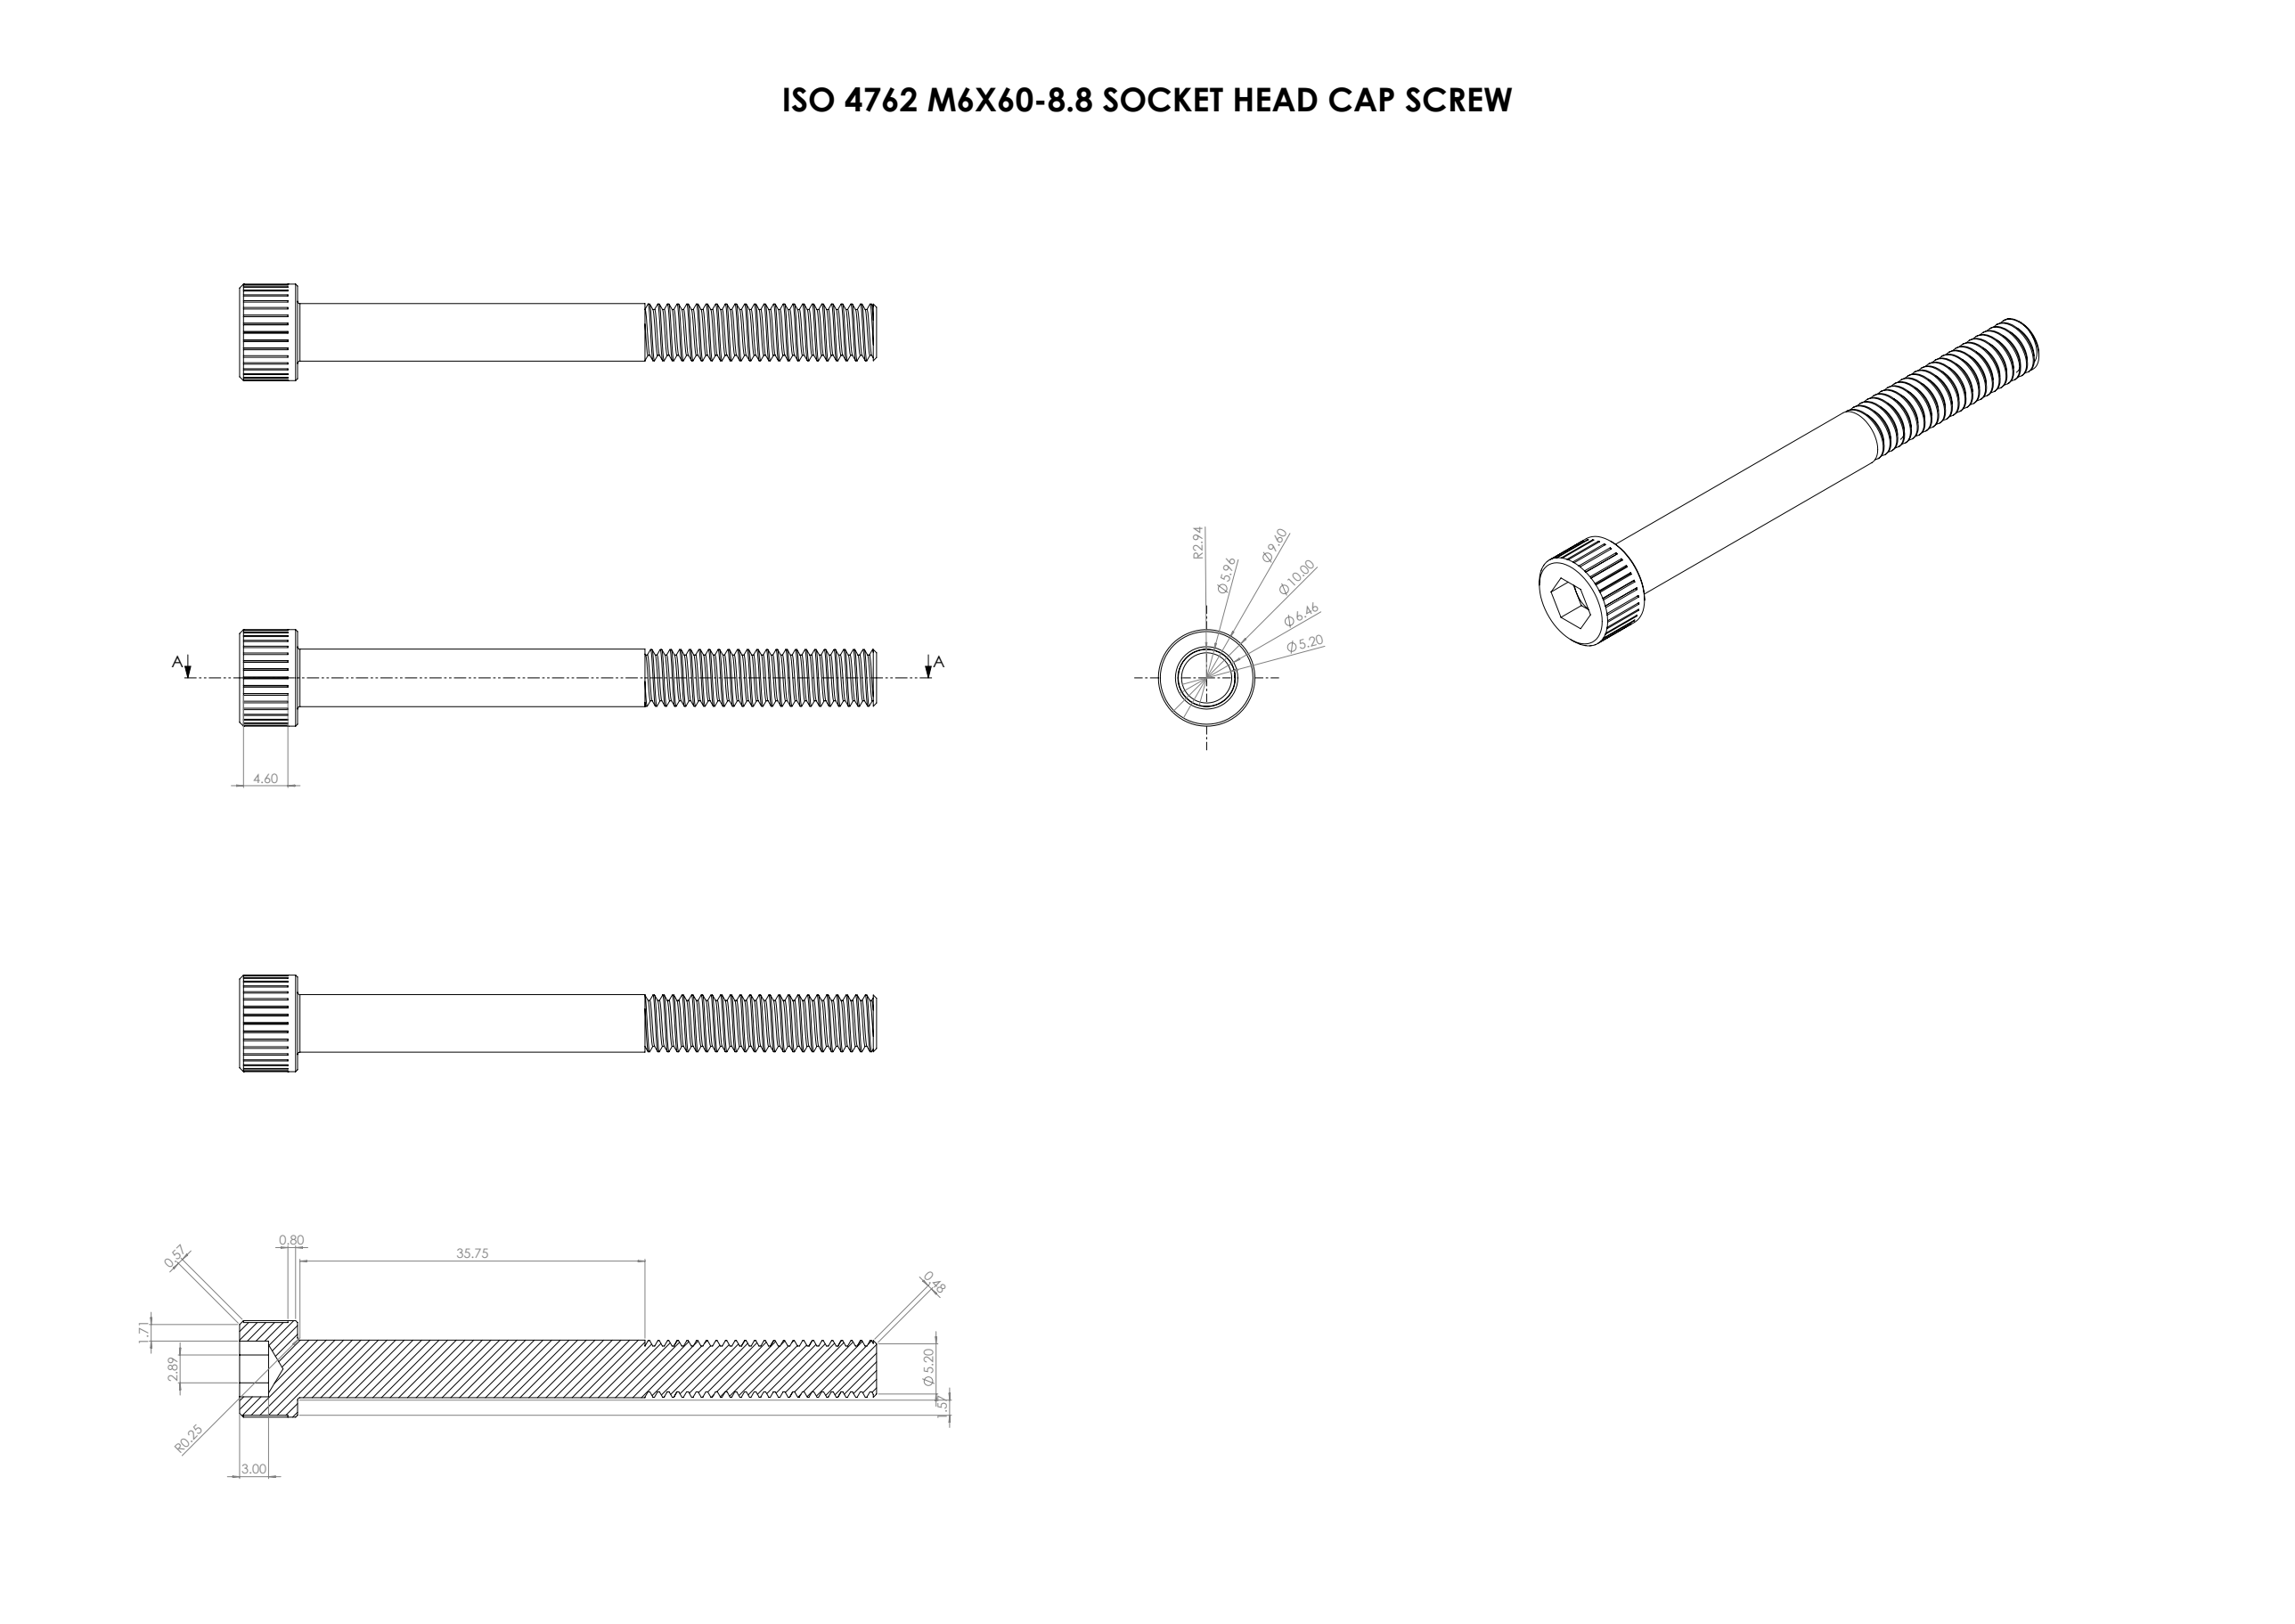
ISO-10303-21;
HEADER;
/* Generated by software containing ST-Developer
 * from STEP Tools, Inc. (www.steptools.com) 
 */

FILE_DESCRIPTION(
/* description */ (''),
/* implementation_level */ '2;1');

FILE_NAME(
/* name */ 
'09_ISO_4762_M6x60-8.8_Socket_Head_Cap_Screw.step',
/* time_stamp */ '2026-10-22T00:21:42-07:00',
/* author */ (''),
/* organization */ (''),
/* preprocessor_version */ 'ST-DEVELOPER v20.2',
/* originating_system */ 'Autodesk Translation Framework v15.15.0.0',
/* authorisation */ '');

FILE_SCHEMA (('AUTOMOTIVE_DESIGN { 1 0 10303 214 3 1 1 }'));
ENDSEC;

DATA;
#10=MECHANICAL_DESIGN_GEOMETRIC_PRESENTATION_REPRESENTATION('',(#213),#31638);
#191=SHAPE_REPRESENTATION_RELATIONSHIP('SRR','None',#31713,#202);
#202=ADVANCED_BREP_SHAPE_REPRESENTATION('',(#224),#31635);
#213=STYLED_ITEM('',(#31837),#224);
#224=MANIFOLD_SOLID_BREP('Socket head cap screw',#12488);
#245=TOROIDAL_SURFACE('',#13459,0.323,0.025);
#307=CYLINDRICAL_SURFACE('',#13176,0.2942);
#308=CYLINDRICAL_SURFACE('',#13178,0.2942);
#309=CYLINDRICAL_SURFACE('',#13179,0.2942);
#310=CYLINDRICAL_SURFACE('',#13180,0.2942);
#311=CYLINDRICAL_SURFACE('',#13181,0.2942);
#312=CYLINDRICAL_SURFACE('',#13182,0.2942);
#313=CYLINDRICAL_SURFACE('',#13183,0.2942);
#314=CYLINDRICAL_SURFACE('',#13184,0.2942);
#315=CYLINDRICAL_SURFACE('',#13185,0.2942);
#316=CYLINDRICAL_SURFACE('',#13186,0.2942);
#317=CYLINDRICAL_SURFACE('',#13187,0.2942);
#318=CYLINDRICAL_SURFACE('',#13188,0.2942);
#319=CYLINDRICAL_SURFACE('',#13189,0.2942);
#320=CYLINDRICAL_SURFACE('',#13190,0.2942);
#321=CYLINDRICAL_SURFACE('',#13191,0.2942);
#322=CYLINDRICAL_SURFACE('',#13192,0.2942);
#323=CYLINDRICAL_SURFACE('',#13193,0.2942);
#324=CYLINDRICAL_SURFACE('',#13194,0.2942);
#325=CYLINDRICAL_SURFACE('',#13195,0.2942);
#326=CYLINDRICAL_SURFACE('',#13196,0.2942);
#327=CYLINDRICAL_SURFACE('',#13197,0.2942);
#328=CYLINDRICAL_SURFACE('',#13198,0.2942);
#329=CYLINDRICAL_SURFACE('',#13199,0.2942);
#330=CYLINDRICAL_SURFACE('',#13200,0.2942);
#331=CYLINDRICAL_SURFACE('',#13201,0.237175);
#332=CYLINDRICAL_SURFACE('',#13203,0.237175);
#333=CYLINDRICAL_SURFACE('',#13205,0.237175);
#334=CYLINDRICAL_SURFACE('',#13206,0.237175);
#335=CYLINDRICAL_SURFACE('',#13207,0.237175);
#336=CYLINDRICAL_SURFACE('',#13208,0.237175);
#337=CYLINDRICAL_SURFACE('',#13209,0.237175);
#338=CYLINDRICAL_SURFACE('',#13210,0.237175);
#339=CYLINDRICAL_SURFACE('',#13211,0.237175);
#340=CYLINDRICAL_SURFACE('',#13212,0.237175);
#341=CYLINDRICAL_SURFACE('',#13213,0.237175);
#342=CYLINDRICAL_SURFACE('',#13214,0.237175);
#343=CYLINDRICAL_SURFACE('',#13215,0.237175);
#344=CYLINDRICAL_SURFACE('',#13216,0.237175);
#345=CYLINDRICAL_SURFACE('',#13217,0.237175);
#346=CYLINDRICAL_SURFACE('',#13218,0.237175);
#347=CYLINDRICAL_SURFACE('',#13219,0.237175);
#348=CYLINDRICAL_SURFACE('',#13220,0.237175);
#349=CYLINDRICAL_SURFACE('',#13221,0.237175);
#350=CYLINDRICAL_SURFACE('',#13222,0.237175);
#351=CYLINDRICAL_SURFACE('',#13223,0.237175);
#352=CYLINDRICAL_SURFACE('',#13224,0.237175);
#353=CYLINDRICAL_SURFACE('',#13225,0.237175);
#354=CYLINDRICAL_SURFACE('',#13226,0.237175);
#355=CYLINDRICAL_SURFACE('',#13231,0.237175);
#356=CYLINDRICAL_SURFACE('',#13463,0.298);
#357=CYLINDRICAL_SURFACE('',#13470,0.2942);
#358=CYLINDRICAL_SURFACE('',#13475,0.5);
#437=CONICAL_SURFACE('',#13232,0.124996333279554,1.03037682652431);
#438=CONICAL_SURFACE('',#13469,0.28,0.785398163397448);
#439=CONICAL_SURFACE('',#13473,0.49,0.785398163397449);
#440=CONICAL_SURFACE('',#13512,0.48,0.785398163397448);
#1046=B_SPLINE_CURVE_WITH_KNOTS('',3,(#26914,#26915,#26916,#26917,#26918,
#26919,#26920,#26921,#26922,#26923),.UNSPECIFIED.,.F.,.F.,(4,3,3,4),(-4.09293042013064,
-3.99248307740831,-2.99436230805624,-2.06863817490914),.UNSPECIFIED.);
#1047=B_SPLINE_CURVE_WITH_KNOTS('',3,(#26926,#26927,#26928,#26929,#26930,
#26931,#26932),.UNSPECIFIED.,.F.,.F.,(4,3,4),(0.,0.998120769352068,1.11730040836818),
 .UNSPECIFIED.);
#1048=B_SPLINE_CURVE_WITH_KNOTS('',3,(#26937,#26938,#26939,#26940,#26941,
#26942,#26943,#26944,#26945,#26946,#26947,#26948,#26949,#26950,#26951,#26952,
#26953,#26954,#26955,#26956,#26957,#26958),.UNSPECIFIED.,.F.,.F.,(4,3,3,
3,3,3,3,4),(-10.3761157273103,-9.98120769352079,-8.98308692416871,-7.98496615481663,
-6.98684538546455,-5.98872461611248,-4.99060384676039,-4.09293042013064),
 .UNSPECIFIED.);
#1049=B_SPLINE_CURVE_WITH_KNOTS('',3,(#26959,#26960,#26961,#26962,#26963,
#26964,#26965,#26966,#26967,#26968,#26969,#26970,#26971,#26972,#26973,#26974,
#26975,#26976,#26977,#26978,#26979,#26980),.UNSPECIFIED.,.F.,.F.,(4,3,3,
3,3,3,3,4),(1.11730040836818,1.99624153870415,2.99436230805623,3.99248307740831,
4.99060384676039,5.98872461611247,6.98684538546454,7.40048571554779),
 .UNSPECIFIED.);
#1050=B_SPLINE_CURVE_WITH_KNOTS('',3,(#26985,#26986,#26987,#26988,#26989,
#26990,#26991,#26992,#26993,#26994,#26995,#26996,#26997,#26998,#26999,#27000,
#27001,#27002,#27003,#27004,#27005,#27006),.UNSPECIFIED.,.F.,.F.,(4,3,3,
3,3,3,3,4),(-16.6593010344898,-15.9699323096333,-14.9718115402812,-13.9736907709291,
-12.975570001577,-11.9774492322249,-10.9793284628729,-10.3761157273103),
 .UNSPECIFIED.);
#1051=B_SPLINE_CURVE_WITH_KNOTS('',3,(#27007,#27008,#27009,#27010,#27011,
#27012,#27013,#27014,#27015,#27016,#27017,#27018,#27019,#27020,#27021,#27022,
#27023,#27024,#27025,#27026,#27027,#27028),.UNSPECIFIED.,.F.,.F.,(4,3,3,
3,3,3,3,4),(7.40048571554779,7.98496615481663,8.9830869241687,9.98120769352078,
10.9793284628729,11.9774492322249,12.975570001577,13.6836710227274),
 .UNSPECIFIED.);
#1052=B_SPLINE_CURVE_WITH_KNOTS('',3,(#27033,#27034,#27035,#27036,#27037,
#27038,#27039,#27040,#27041,#27042,#27043,#27044,#27045,#27046,#27047,#27048,
#27049,#27050,#27051,#27052,#27053,#27054),.UNSPECIFIED.,.F.,.F.,(4,3,3,
3,3,3,3,4),(-22.9424863416694,-21.9586569257457,-20.9605361563937,-19.9624153870416,
-18.9642946176895,-17.9661738483374,-16.9680530789853,-16.6593010344898),
 .UNSPECIFIED.);
#1053=B_SPLINE_CURVE_WITH_KNOTS('',3,(#27055,#27056,#27057,#27058,#27059,
#27060,#27061,#27062,#27063,#27064,#27065,#27066,#27067,#27068,#27069,#27070,
#27071,#27072,#27073,#27074,#27075,#27076,#27077,#27078,#27079),
 .UNSPECIFIED.,.F.,.F.,(4,3,3,3,3,3,3,3,4),(13.6836710227274,13.9736907709291,
14.9718115402812,15.9699323096333,16.9680530789853,17.9661738483374,18.9642946176895,
19.9624153870416,19.966856329907),.UNSPECIFIED.);
#1054=B_SPLINE_CURVE_WITH_KNOTS('',3,(#27084,#27085,#27086,#27087,#27088,
#27089,#27090,#27091,#27092,#27093,#27094,#27095,#27096,#27097,#27098,#27099,
#27100,#27101,#27102,#27103,#27104,#27105,#27106,#27107,#27108),
 .UNSPECIFIED.,.F.,.F.,(4,3,3,3,3,3,3,3,4),(-29.225671648849,-28.9455023112103,
-27.9473815418582,-26.9492607725061,-25.9511400031541,-24.953019233802,
-23.9548984644499,-22.9567776950978,-22.9424863416694),.UNSPECIFIED.);
#1055=B_SPLINE_CURVE_WITH_KNOTS('',3,(#27109,#27110,#27111,#27112,#27113,
#27114,#27115,#27116,#27117,#27118,#27119,#27120,#27121,#27122,#27123,#27124,
#27125,#27126,#27127,#27128,#27129,#27130),.UNSPECIFIED.,.F.,.F.,(4,3,3,
3,3,3,3,4),(19.966856329907,20.9605361563937,21.9586569257457,22.9567776950978,
23.9548984644499,24.953019233802,25.9511400031541,26.2500416370865),
 .UNSPECIFIED.);
#1056=B_SPLINE_CURVE_WITH_KNOTS('',3,(#27135,#27136,#27137,#27138,#27139,
#27140,#27141,#27142,#27143,#27144,#27145,#27146,#27147,#27148,#27149,#27150,
#27151,#27152,#27153,#27154,#27155,#27156),.UNSPECIFIED.,.F.,.F.,(4,3,3,
3,3,3,3,4),(-35.5088569560286,-34.9342269273228,-33.9361061579707,-32.9379853886186,
-31.9398646192665,-30.9417438499144,-29.9436230805624,-29.225671648849),
 .UNSPECIFIED.);
#1057=B_SPLINE_CURVE_WITH_KNOTS('',3,(#27157,#27158,#27159,#27160,#27161,
#27162,#27163,#27164,#27165,#27166,#27167,#27168,#27169,#27170,#27171,#27172,
#27173,#27174,#27175,#27176,#27177,#27178),.UNSPECIFIED.,.F.,.F.,(4,3,3,
3,3,3,3,4),(26.2500416370865,26.9492607725061,27.9473815418582,28.9455023112103,
29.9436230805624,30.9417438499144,31.9398646192665,32.5332269442662),
 .UNSPECIFIED.);
#1058=B_SPLINE_CURVE_WITH_KNOTS('',3,(#27183,#27184,#27185,#27186,#27187,
#27188,#27189,#27190,#27191,#27192,#27193,#27194,#27195,#27196,#27197,#27198,
#27199,#27200,#27201,#27202,#27203,#27204),.UNSPECIFIED.,.F.,.F.,(4,3,3,
3,3,3,3,4),(-41.7920422632082,-40.9229515434352,-39.9248307740831,-38.9267100047311,
-37.928589235379,-36.9304684660269,-35.9323476966748,-35.5088569560286),
 .UNSPECIFIED.);
#1059=B_SPLINE_CURVE_WITH_KNOTS('',3,(#27205,#27206,#27207,#27208,#27209,
#27210,#27211,#27212,#27213,#27214,#27215,#27216,#27217,#27218,#27219,#27220,
#27221,#27222,#27223,#27224,#27225,#27226),.UNSPECIFIED.,.F.,.F.,(4,3,3,
3,3,3,3,4),(32.5332269442662,32.9379853886186,33.9361061579707,34.9342269273227,
35.9323476966748,36.9304684660269,37.928589235379,38.8164122514457),
 .UNSPECIFIED.);
#1060=B_SPLINE_CURVE_WITH_KNOTS('',3,(#27231,#27232,#27233,#27234,#27235,
#27236,#27237,#27238,#27239,#27240,#27241,#27242,#27243,#27244,#27245,#27246,
#27247,#27248,#27249,#27250,#27251,#27252,#27253,#27254,#27255),
 .UNSPECIFIED.,.F.,.F.,(4,3,3,3,3,3,3,3,4),(-48.0752275703878,-47.9097969288998,
-46.9116761595477,-45.9135553901956,-44.9154346208435,-43.9173138514915,
-42.9191930821394,-41.9210723127873,-41.7920422632082),.UNSPECIFIED.);
#1061=B_SPLINE_CURVE_WITH_KNOTS('',3,(#27256,#27257,#27258,#27259,#27260,
#27261,#27262,#27263,#27264,#27265,#27266,#27267,#27268,#27269,#27270,#27271,
#27272,#27273,#27274,#27275,#27276,#27277,#27278,#27279,#27280),
 .UNSPECIFIED.,.F.,.F.,(4,3,3,3,3,3,3,3,4),(38.8164122514457,38.9267100047311,
39.9248307740831,40.9229515434352,41.9210723127873,42.9191930821394,43.9173138514915,
44.9154346208435,45.0995975586253),.UNSPECIFIED.);
#1062=B_SPLINE_CURVE_WITH_KNOTS('',3,(#27285,#27286,#27287,#27288,#27289,
#27290,#27291,#27292,#27293,#27294,#27295,#27296,#27297,#27298,#27299,#27300,
#27301,#27302,#27303,#27304,#27305,#27306),.UNSPECIFIED.,.F.,.F.,(4,3,3,
3,3,3,3,4),(-54.3584128775674,-53.8985215450123,-52.9004007756602,-51.9022800063081,
-50.904159236956,-49.9060384676039,-48.9079176982519,-48.0752275703878),
 .UNSPECIFIED.);
#1063=B_SPLINE_CURVE_WITH_KNOTS('',3,(#27307,#27308,#27309,#27310,#27311,
#27312,#27313,#27314,#27315,#27316,#27317,#27318,#27319,#27320,#27321,#27322,
#27323,#27324,#27325,#27326,#27327,#27328),.UNSPECIFIED.,.F.,.F.,(4,3,3,
3,3,3,3,4),(45.0995975586253,45.9135553901956,46.9116761595477,47.9097969288998,
48.9079176982519,49.9060384676039,50.904159236956,51.3827828658049),
 .UNSPECIFIED.);
#1064=B_SPLINE_CURVE_WITH_KNOTS('',3,(#27333,#27334,#27335,#27336,#27337,
#27338,#27339,#27340,#27341,#27342,#27343,#27344,#27345,#27346,#27347,#27348,
#27349,#27350,#27351,#27352,#27353,#27354),.UNSPECIFIED.,.F.,.F.,(4,3,3,
3,3,3,3,4),(-60.6415981847469,-59.8872461611247,-58.8891253917727,-57.8910046224206,
-56.8928838530685,-55.8947630837164,-54.8966423143643,-54.3584128775674),
 .UNSPECIFIED.);
#1065=B_SPLINE_CURVE_WITH_KNOTS('',3,(#27355,#27356,#27357,#27358,#27359,
#27360,#27361,#27362,#27363,#27364,#27365,#27366,#27367,#27368,#27369,#27370,
#27371,#27372,#27373,#27374,#27375,#27376),.UNSPECIFIED.,.F.,.F.,(4,3,3,
3,3,3,3,4),(51.3827828658049,51.9022800063081,52.9004007756602,53.8985215450123,
54.8966423143643,55.8947630837164,56.8928838530685,57.6659681729845),
 .UNSPECIFIED.);
#1066=B_SPLINE_CURVE_WITH_KNOTS('',3,(#27381,#27382,#27383,#27384,#27385,
#27386,#27387,#27388,#27389,#27390,#27391,#27392,#27393,#27394,#27395,#27396,
#27397,#27398,#27399,#27400,#27401,#27402,#27403,#27404,#27405),
 .UNSPECIFIED.,.F.,.F.,(4,3,3,3,3,3,3,3,4),(-66.9247834919266,-66.8740915465893,
-65.8759707772372,-64.8778500078851,-63.879729238533,-62.881608469181,-61.8834876998289,
-60.8853669304768,-60.6415981847469),.UNSPECIFIED.);
#1067=B_SPLINE_CURVE_WITH_KNOTS('',3,(#27406,#27407,#27408,#27409,#27410,
#27411,#27412,#27413,#27414,#27415,#27416,#27417,#27418,#27419,#27420,#27421,
#27422,#27423,#27424,#27425,#27426,#27427,#27428,#27429,#27430),
 .UNSPECIFIED.,.F.,.F.,(4,3,3,3,3,3,3,3,4),(57.6659681729845,57.8910046224206,
58.8891253917727,59.8872461611247,60.8853669304768,61.8834876998289,62.881608469181,
63.8797292385331,63.9491534801641),.UNSPECIFIED.);
#1068=B_SPLINE_CURVE_WITH_KNOTS('',3,(#27435,#27436,#27437,#27438,#27439,
#27440,#27441,#27442,#27443,#27444,#27445,#27446,#27447,#27448,#27449,#27450,
#27451,#27452,#27453,#27454,#27455,#27456),.UNSPECIFIED.,.F.,.F.,(4,3,3,
3,3,3,3,4),(-73.2079687991062,-72.8628161627017,-71.8646953933497,-70.8665746239976,
-69.8684538546455,-68.8703330852934,-67.8722123159413,-66.9247834919266),
 .UNSPECIFIED.);
#1069=B_SPLINE_CURVE_WITH_KNOTS('',3,(#27457,#27458,#27459,#27460,#27461,
#27462,#27463,#27464,#27465,#27466,#27467,#27468,#27469,#27470,#27471,#27472,
#27473,#27474,#27475,#27476,#27477,#27478),.UNSPECIFIED.,.F.,.F.,(4,3,3,
3,3,3,3,4),(63.9491534801641,64.8778500078851,65.8759707772372,66.8740915465893,
67.8722123159414,68.8703330852934,69.8684538546455,70.2323387873437),
 .UNSPECIFIED.);
#1070=B_SPLINE_CURVE_WITH_KNOTS('',3,(#27483,#27484,#27485,#27486,#27487,
#27488,#27489,#27490,#27491,#27492,#27493,#27494,#27495,#27496,#27497,#27498,
#27499,#27500,#27501,#27502,#27503,#27504),.UNSPECIFIED.,.F.,.F.,(4,3,3,
3,3,3,3,4),(-79.4911541062857,-78.8515407788142,-77.8534200094622,-76.8552992401101,
-75.857178470758,-74.8590577014059,-73.8609369320538,-73.2079687991062),
 .UNSPECIFIED.);
#1071=B_SPLINE_CURVE_WITH_KNOTS('',3,(#27505,#27506,#27507,#27508,#27509,
#27510,#27511,#27512,#27513,#27514,#27515,#27516,#27517,#27518,#27519,#27520,
#27521,#27522,#27523,#27524,#27525,#27526),.UNSPECIFIED.,.F.,.F.,(4,3,3,
3,3,3,3,4),(70.2323387873437,70.8665746239976,71.8646953933497,72.8628161627017,
73.8609369320538,74.8590577014059,75.857178470758,76.5155240945233),
 .UNSPECIFIED.);
#1072=B_SPLINE_CURVE_WITH_KNOTS('',3,(#27531,#27532,#27533,#27534,#27535,
#27536,#27537,#27538,#27539,#27540,#27541,#27542,#27543,#27544,#27545,#27546,
#27547,#27548,#27549,#27550,#27551,#27552),.UNSPECIFIED.,.F.,.F.,(4,3,3,
3,3,3,3,4),(-85.7743394134653,-84.8402653949267,-83.8421446255746,-82.8440238562225,
-81.8459030868705,-80.8477823175184,-79.8496615481663,-79.4911541062857),
 .UNSPECIFIED.);
#1073=B_SPLINE_CURVE_WITH_KNOTS('',3,(#27553,#27554,#27555,#27556,#27557,
#27558,#27559,#27560,#27561,#27562,#27563,#27564,#27565,#27566,#27567,#27568,
#27569,#27570,#27571,#27572,#27573,#27574),.UNSPECIFIED.,.F.,.F.,(4,3,3,
3,3,3,3,4),(76.5155240945233,76.8552992401101,77.8534200094622,78.8515407788142,
79.8496615481663,80.8477823175184,81.8459030868705,82.7987094017029),
 .UNSPECIFIED.);
#1074=B_SPLINE_CURVE_WITH_KNOTS('',3,(#27579,#27580,#27581,#27582,#27583,
#27584,#27585,#27586,#27587,#27588,#27589,#27590,#27591,#27592,#27593,#27594,
#27595,#27596,#27597,#27598,#27599,#27600,#27601,#27602,#27603),
 .UNSPECIFIED.,.F.,.F.,(4,3,3,3,3,3,3,3,4),(-92.0575247206449,-91.8271107803912,
-90.8289900110392,-89.8308692416871,-88.832748472335,-87.8346277029829,
-86.8365069336308,-85.8383861642788,-85.7743394134653),.UNSPECIFIED.);
#1075=B_SPLINE_CURVE_WITH_KNOTS('',3,(#27604,#27605,#27606,#27607,#27608,
#27609,#27610,#27611,#27612,#27613,#27614,#27615,#27616,#27617,#27618,#27619,
#27620,#27621,#27622,#27623,#27624,#27625,#27626,#27627,#27628),
 .UNSPECIFIED.,.F.,.F.,(4,3,3,3,3,3,3,3,4),(82.7987094017029,82.8440238562225,
83.8421446255746,84.8402653949267,85.8383861642788,86.8365069336308,87.834627702983,
88.832748472335,89.0818947088825),.UNSPECIFIED.);
#1076=B_SPLINE_CURVE_WITH_KNOTS('',3,(#27633,#27634,#27635,#27636,#27637,
#27638,#27639,#27640,#27641,#27642,#27643,#27644,#27645,#27646,#27647,#27648,
#27649,#27650,#27651,#27652,#27653,#27654),.UNSPECIFIED.,.F.,.F.,(4,3,3,
3,3,3,3,4),(-98.3407100278245,-97.8158353965037,-96.8177146271516,-95.8195938577995,
-94.8214730884475,-93.8233523190954,-92.8252315497433,-92.0575247206449),
 .UNSPECIFIED.);
#1077=B_SPLINE_CURVE_WITH_KNOTS('',3,(#27655,#27656,#27657,#27658,#27659,
#27660,#27661,#27662,#27663,#27664,#27665,#27666,#27667,#27668,#27669,#27670,
#27671,#27672,#27673,#27674,#27675,#27676),.UNSPECIFIED.,.F.,.F.,(4,3,3,
3,3,3,3,4),(89.0818947088825,89.8308692416871,90.8289900110392,91.8271107803912,
92.8252315497433,93.8233523190954,94.8214730884475,95.3650800160621),
 .UNSPECIFIED.);
#1078=B_SPLINE_CURVE_WITH_KNOTS('',3,(#27681,#27682,#27683,#27684,#27685,
#27686,#27687,#27688,#27689,#27690,#27691,#27692,#27693,#27694,#27695,#27696,
#27697,#27698,#27699,#27700,#27701,#27702),.UNSPECIFIED.,.F.,.F.,(4,3,3,
3,3,3,3,4),(-104.623895335004,-103.804560012616,-102.806439243264,-101.808318473912,
-100.81019770456,-99.8120769352079,-98.8139561658558,-98.3407100278245),
 .UNSPECIFIED.);
#1079=B_SPLINE_CURVE_WITH_KNOTS('',3,(#27703,#27704,#27705,#27706,#27707,
#27708,#27709,#27710,#27711,#27712,#27713,#27714,#27715,#27716,#27717,#27718,
#27719,#27720,#27721,#27722,#27723,#27724),.UNSPECIFIED.,.F.,.F.,(4,3,3,
3,3,3,3,4),(95.3650800160621,95.8195938577996,96.8177146271516,97.8158353965037,
98.8139561658558,99.8120769352079,100.81019770456,101.648265323242),
 .UNSPECIFIED.);
#1080=B_SPLINE_CURVE_WITH_KNOTS('',3,(#27729,#27730,#27731,#27732,#27733,
#27734,#27735,#27736,#27737,#27738,#27739,#27740,#27741,#27742,#27743,#27744,
#27745,#27746,#27747,#27748,#27749,#27750,#27751,#27752,#27753),
 .UNSPECIFIED.,.F.,.F.,(4,3,3,3,3,3,3,3,4),(-110.907080642184,-110.791405398081,
-109.793284628729,-108.795163859377,-107.797043090025,-106.798922320672,
-105.80080155132,-104.802680781968,-104.623895335004),.UNSPECIFIED.);
#1081=B_SPLINE_CURVE_WITH_KNOTS('',3,(#27754,#27755,#27756,#27757,#27758,
#27759,#27760,#27761,#27762,#27763,#27764,#27765,#27766,#27767,#27768,#27769,
#27770,#27771,#27772,#27773,#27774,#27775,#27776,#27777,#27778),
 .UNSPECIFIED.,.F.,.F.,(4,3,3,3,3,3,3,3,4),(101.648265323242,101.808318473912,
102.806439243264,103.804560012616,104.802680781968,105.80080155132,106.798922320672,
107.797043090025,107.931450630421),.UNSPECIFIED.);
#1082=B_SPLINE_CURVE_WITH_KNOTS('',3,(#27783,#27784,#27785,#27786,#27787,
#27788,#27789,#27790,#27791,#27792,#27793,#27794,#27795,#27796,#27797,#27798,
#27799,#27800,#27801,#27802,#27803,#27804),.UNSPECIFIED.,.F.,.F.,(4,3,3,
3,3,3,3,4),(-117.190265949363,-116.780130014193,-115.782009244841,-114.783888475489,
-113.785767706137,-112.787646936785,-111.789526167433,-110.907080642184),
 .UNSPECIFIED.);
#1083=B_SPLINE_CURVE_WITH_KNOTS('',3,(#27805,#27806,#27807,#27808,#27809,
#27810,#27811,#27812,#27813,#27814,#27815,#27816,#27817,#27818,#27819,#27820,
#27821,#27822,#27823,#27824,#27825,#27826),.UNSPECIFIED.,.F.,.F.,(4,3,3,
3,3,3,3,4),(107.931450630421,108.795163859377,109.793284628729,110.791405398081,
111.789526167433,112.787646936785,113.785767706137,114.214635937601),
 .UNSPECIFIED.);
#1084=B_SPLINE_CURVE_WITH_KNOTS('',3,(#27831,#27832,#27833,#27834,#27835,
#27836,#27837,#27838,#27839,#27840,#27841,#27842,#27843,#27844,#27845,#27846,
#27847,#27848,#27849,#27850,#27851,#27852),.UNSPECIFIED.,.F.,.F.,(4,3,3,
3,3,3,3,4),(-123.473451256543,-122.768854630306,-121.770733860954,-120.772613091602,
-119.774492322249,-118.776371552897,-117.778250783545,-117.190265949363),
 .UNSPECIFIED.);
#1085=B_SPLINE_CURVE_WITH_KNOTS('',3,(#27853,#27854,#27855,#27856,#27857,
#27858,#27859,#27860,#27861,#27862,#27863,#27864,#27865,#27866,#27867,#27868,
#27869,#27870,#27871,#27872,#27873,#27874),.UNSPECIFIED.,.F.,.F.,(4,3,3,
3,3,3,3,4),(114.214635937601,114.783888475489,115.782009244841,116.780130014193,
117.778250783545,118.776371552897,119.774492322249,120.49782124478),
 .UNSPECIFIED.);
#1086=B_SPLINE_CURVE_WITH_KNOTS('',3,(#27879,#27880,#27881,#27882,#27883,
#27884,#27885,#27886,#27887,#27888,#27889,#27890,#27891,#27892,#27893,#27894,
#27895,#27896,#27897,#27898,#27899,#27900),.UNSPECIFIED.,.F.,.F.,(4,3,3,
3,3,3,3,4),(-129.756636563722,-128.757579246418,-127.759458477066,-126.761337707714,
-125.763216938362,-124.76509616901,-123.766975399658,-123.473451256543),
 .UNSPECIFIED.);
#1087=B_SPLINE_CURVE_WITH_KNOTS('',3,(#27901,#27902,#27903,#27904,#27905,
#27906,#27907,#27908,#27909,#27910,#27911,#27912,#27913,#27914,#27915,#27916,
#27917,#27918,#27919,#27920,#27921,#27922,#27923,#27924,#27925),
 .UNSPECIFIED.,.F.,.F.,(4,3,3,3,3,3,3,3,4),(120.49782124478,120.772613091602,
121.770733860954,122.768854630306,123.766975399658,124.76509616901,125.763216938362,
126.761337707714,126.78100655196),.UNSPECIFIED.);
#1088=B_SPLINE_CURVE_WITH_KNOTS('',3,(#27930,#27931,#27932,#27933,#27934,
#27935,#27936,#27937,#27938,#27939,#27940,#27941,#27942,#27943,#27944,#27945,
#27946,#27947,#27948,#27949,#27950,#27951),.UNSPECIFIED.,.F.,.F.,(4,3,3,
3,3,3,3,4),(-136.039821870902,-135.744424631883,-134.746303862531,-133.748183093179,
-132.750062323826,-131.751941554474,-130.753820785122,-129.756636563722),
 .UNSPECIFIED.);
#1089=B_SPLINE_CURVE_WITH_KNOTS('',3,(#27952,#27953,#27954,#27955,#27956,
#27957,#27958,#27959,#27960,#27961,#27962,#27963,#27964,#27965,#27966,#27967,
#27968,#27969,#27970,#27971,#27972,#27973),.UNSPECIFIED.,.F.,.F.,(4,3,3,
3,3,3,3,4),(126.78100655196,127.759458477066,128.757579246418,129.75570001577,
130.753820785122,131.751941554474,132.750062323826,133.06419185914),
 .UNSPECIFIED.);
#1090=B_SPLINE_CURVE_WITH_KNOTS('',3,(#27978,#27979,#27980,#27981,#27982,
#27983,#27984,#27985,#27986,#27987,#27988,#27989,#27990,#27991,#27992,#27993,
#27994,#27995,#27996,#27997,#27998,#27999),.UNSPECIFIED.,.F.,.F.,(4,3,3,
3,3,3,3,4),(-142.323007178082,-141.733149247995,-140.735028478643,-139.736907709291,
-138.738786939939,-137.740666170587,-136.742545401235,-136.039821870902),
 .UNSPECIFIED.);
#1091=B_SPLINE_CURVE_WITH_KNOTS('',3,(#28000,#28001,#28002,#28003,#28004,
#28005,#28006,#28007,#28008,#28009,#28010,#28011,#28012,#28013,#28014,#28015,
#28016,#28017,#28018,#28019,#28020,#28021),.UNSPECIFIED.,.F.,.F.,(4,3,3,
3,3,3,3,4),(133.06419185914,133.748183093179,134.746303862531,135.744424631883,
136.742545401235,137.740666170587,138.738786939939,139.347377166319),
 .UNSPECIFIED.);
#1092=B_SPLINE_CURVE_WITH_KNOTS('',3,(#28026,#28027,#28028,#28029,#28030,
#28031,#28032,#28033,#28034,#28035,#28036,#28037,#28038,#28039,#28040,#28041,
#28042,#28043,#28044,#28045,#28046,#28047),.UNSPECIFIED.,.F.,.F.,(4,3,3,
3,3,3,3,4),(-148.606192485261,-147.721873864108,-146.723753094756,-145.725632325403,
-144.727511556051,-143.729390786699,-142.731270017347,-142.323007178082),
 .UNSPECIFIED.);
#1093=B_SPLINE_CURVE_WITH_KNOTS('',3,(#28048,#28049,#28050,#28051,#28052,
#28053,#28054,#28055,#28056,#28057,#28058,#28059,#28060,#28061,#28062,#28063,
#28064,#28065,#28066,#28067,#28068,#28069),.UNSPECIFIED.,.F.,.F.,(4,3,3,
3,3,3,3,4),(139.347377166319,139.736907709291,140.735028478643,141.733149247995,
142.731270017347,143.729390786699,144.727511556051,145.630562473499),
 .UNSPECIFIED.);
#1094=B_SPLINE_CURVE_WITH_KNOTS('',3,(#28075,#28076,#28077,#28078),
 .UNSPECIFIED.,.F.,.F.,(4,4),(160.221225333079,160.262630845073),
 .UNSPECIFIED.);
#1095=B_SPLINE_CURVE_WITH_KNOTS('',3,(#28084,#28085,#28086,#28087,#28088,
#28089,#28090,#28091,#28092,#28093),.UNSPECIFIED.,.F.,.F.,(4,1,1,1,1,1,
1,4),(153.9380400259,154.346302865166,155.344423634518,156.34254440387,
157.340665173222,158.338785942574,159.336906711926,160.221225333079),
 .UNSPECIFIED.);
#1096=B_SPLINE_CURVE_WITH_KNOTS('',3,(#28096,#28097,#28098,#28099,#28100,
#28101,#28102,#28103,#28104),.UNSPECIFIED.,.F.,.F.,(4,1,1,1,1,1,4),(153.9380400259,
154.033109877805,155.031230647157,156.029351416509,157.027472185861,158.025592955213,
159.023713724565),.UNSPECIFIED.);
#1097=B_SPLINE_CURVE_WITH_KNOTS('',3,(#28109,#28110,#28111,#28112,#28113,
#28114,#28115,#28116,#28117,#28118),.UNSPECIFIED.,.F.,.F.,(4,1,1,1,1,1,
1,4),(147.65485471872,148.357578249053,149.355699018405,150.353819787757,
151.351940557109,152.350061326461,153.348182095814,153.9380400259),
 .UNSPECIFIED.);
#1098=B_SPLINE_CURVE_WITH_KNOTS('',3,(#28119,#28120,#28121,#28122,#28123,
#28124,#28125,#28126,#28127,#28128),.UNSPECIFIED.,.F.,.F.,(4,1,1,1,1,1,
1,4),(147.65485471872,148.044385261692,149.042506031044,150.040626800396,
151.038747569748,152.0368683391,153.034989108453,153.9380400259),
 .UNSPECIFIED.);
#1099=B_SPLINE_CURVE_WITH_KNOTS('',3,(#28133,#28134,#28135,#28136,#28137,
#28138,#28139,#28140,#28141,#28142),.UNSPECIFIED.,.F.,.F.,(4,1,1,1,1,1,
1,4),(141.371669411541,142.368853632941,143.366974402293,144.365095171645,
145.363215940997,146.361336710349,147.359457479701,147.65485471872),
 .UNSPECIFIED.);
#1100=B_SPLINE_CURVE_WITH_KNOTS('',3,(#28143,#28144,#28145,#28146,#28147,
#28148,#28149,#28150,#28151,#28152),.UNSPECIFIED.,.F.,.F.,(4,1,1,1,1,1,
1,4),(141.371669411541,142.05566064558,143.053781414932,144.051902184284,
145.050022953636,146.048143722988,147.04626449234,147.65485471872),
 .UNSPECIFIED.);
#1101=B_SPLINE_CURVE_WITH_KNOTS('',3,(#28157,#28158,#28159,#28160,#28161,
#28162,#28163,#28164,#28165,#28166,#28167),.UNSPECIFIED.,.F.,.F.,(4,1,1,
1,1,1,1,1,4),(135.088484104361,135.382008247476,136.380129016828,137.37824978618,
138.376370555532,139.374491324884,140.372612094236,141.370732863589,141.371669411541),
 .UNSPECIFIED.);
#1102=B_SPLINE_CURVE_WITH_KNOTS('',3,(#28168,#28169,#28170,#28171,#28172,
#28173,#28174,#28175,#28176,#28177),.UNSPECIFIED.,.F.,.F.,(4,1,1,1,1,1,
1,4),(135.088484104361,136.066936029467,137.065056798819,138.063177568171,
139.061298337523,140.059419106876,141.057539876228,141.371669411541),
 .UNSPECIFIED.);
#1103=B_SPLINE_CURVE_WITH_KNOTS('',3,(#28182,#28183,#28184,#28185,#28186,
#28187,#28188,#28189,#28190,#28191),.UNSPECIFIED.,.F.,.F.,(4,1,1,1,1,1,
1,4),(128.805298797182,129.393283631364,130.391404400716,131.389525170068,
132.38764593942,133.385766708772,134.383887478124,135.088484104361),
 .UNSPECIFIED.);
#1104=B_SPLINE_CURVE_WITH_KNOTS('',3,(#28192,#28193,#28194,#28195,#28196,
#28197,#28198,#28199,#28200,#28201,#28202),.UNSPECIFIED.,.F.,.F.,(4,1,1,
1,1,1,1,1,4),(128.805298797182,129.080090644003,130.078211413355,131.076332182707,
132.074452952059,133.072573721411,134.070694490763,135.068815260115,135.088484104361),
 .UNSPECIFIED.);
#1105=B_SPLINE_CURVE_WITH_KNOTS('',3,(#28207,#28208,#28209,#28210,#28211,
#28212,#28213,#28214,#28215,#28216),.UNSPECIFIED.,.F.,.F.,(4,1,1,1,1,1,
1,4),(122.522113490002,123.404559015251,124.402679784603,125.400800553955,
126.398921323307,127.397042092659,128.395162862012,128.805298797182),
 .UNSPECIFIED.);
#1106=B_SPLINE_CURVE_WITH_KNOTS('',3,(#28217,#28218,#28219,#28220,#28221,
#28222,#28223,#28224,#28225,#28226),.UNSPECIFIED.,.F.,.F.,(4,1,1,1,1,1,
1,4),(122.522113490002,123.09136602789,124.089486797242,125.087607566594,
126.085728335946,127.083849105298,128.081969874651,128.805298797182),
 .UNSPECIFIED.);
#1107=B_SPLINE_CURVE_WITH_KNOTS('',3,(#28231,#28232,#28233,#28234,#28235,
#28236,#28237,#28238,#28239,#28240,#28241),.UNSPECIFIED.,.F.,.F.,(4,1,1,
1,1,1,1,1,4),(116.238928182822,116.417713629787,117.415834399139,118.413955168491,
119.412075937843,120.410196707195,121.408317476547,122.406438245899,122.522113490002),
 .UNSPECIFIED.);
#1108=B_SPLINE_CURVE_WITH_KNOTS('',3,(#28242,#28243,#28244,#28245,#28246,
#28247,#28248,#28249,#28250,#28251),.UNSPECIFIED.,.F.,.F.,(4,1,1,1,1,1,
1,4),(116.238928182822,117.102641411778,118.10076218113,119.098882950482,
120.097003719834,121.095124489186,122.093245258538,122.522113490002),
 .UNSPECIFIED.);
#1109=B_SPLINE_CURVE_WITH_KNOTS('',3,(#28256,#28257,#28258,#28259,#28260,
#28261,#28262,#28263,#28264,#28265),.UNSPECIFIED.,.F.,.F.,(4,1,1,1,1,1,
1,4),(109.955742875643,110.428989013674,111.427109783026,112.425230552378,
113.42335132173,114.421472091082,115.419592860435,116.238928182822),
 .UNSPECIFIED.);
#1110=B_SPLINE_CURVE_WITH_KNOTS('',3,(#28266,#28267,#28268,#28269,#28270,
#28271,#28272,#28273,#28274,#28275,#28276),.UNSPECIFIED.,.F.,.F.,(4,1,1,
1,1,1,1,1,4),(109.955742875643,110.115796026313,111.113916795665,112.112037565017,
113.110158334369,114.108279103721,115.106399873074,116.104520642426,116.238928182822),
 .UNSPECIFIED.);
#1111=B_SPLINE_CURVE_WITH_KNOTS('',3,(#28281,#28282,#28283,#28284,#28285,
#28286,#28287,#28288,#28289,#28290),.UNSPECIFIED.,.F.,.F.,(4,1,1,1,1,1,
1,4),(103.672557568463,104.440264397562,105.438385166914,106.436505936266,
107.434626705618,108.43274747497,109.430868244322,109.955742875643),
 .UNSPECIFIED.);
#1112=B_SPLINE_CURVE_WITH_KNOTS('',3,(#28291,#28292,#28293,#28294,#28295,
#28296,#28297,#28298,#28299,#28300),.UNSPECIFIED.,.F.,.F.,(4,1,1,1,1,1,
1,4),(103.672557568463,104.127071410201,105.125192179553,106.123312948905,
107.121433718257,108.119554487609,109.117675256961,109.955742875643),
 .UNSPECIFIED.);
#1113=B_SPLINE_CURVE_WITH_KNOTS('',3,(#28305,#28306,#28307,#28308,#28309,
#28310,#28311,#28312,#28313,#28314,#28315),.UNSPECIFIED.,.F.,.F.,(4,1,1,
1,1,1,1,1,4),(97.3893722612836,97.4534190120971,98.4515397814492,99.4496605508013,
100.447781320153,101.445902089505,102.444022858857,103.44214362821,103.672557568463),
 .UNSPECIFIED.);
#1114=B_SPLINE_CURVE_WITH_KNOTS('',3,(#28316,#28317,#28318,#28319,#28320,
#28321,#28322,#28323,#28324,#28325),.UNSPECIFIED.,.F.,.F.,(4,1,1,1,1,1,
1,4),(97.3893722612836,98.1383467940882,99.1364675634403,100.134588332792,
101.132709102144,102.130829871497,103.128950640849,103.672557568463),
 .UNSPECIFIED.);
#1115=B_SPLINE_CURVE_WITH_KNOTS('',3,(#28330,#28331,#28332,#28333,#28334,
#28335,#28336,#28337,#28338,#28339),.UNSPECIFIED.,.F.,.F.,(4,1,1,1,1,1,
1,4),(91.106186954104,91.4646943959846,92.4628151653367,93.4609359346888,
94.4590567040409,95.4571774733929,96.455298242745,97.3893722612836),
 .UNSPECIFIED.);
#1116=B_SPLINE_CURVE_WITH_KNOTS('',3,(#28340,#28341,#28342,#28343,#28344,
#28345,#28346,#28347,#28348,#28349,#28350),.UNSPECIFIED.,.F.,.F.,(4,1,1,
1,1,1,1,1,4),(91.106186954104,91.1515014086236,92.1496221779757,93.1477429473278,
94.1458637166799,95.143984486032,96.142105255384,97.1402260247361,97.3893722612836),
 .UNSPECIFIED.);
#1117=B_SPLINE_CURVE_WITH_KNOTS('',3,(#28355,#28356,#28357,#28358,#28359,
#28360,#28361,#28362,#28363,#28364),.UNSPECIFIED.,.F.,.F.,(4,1,1,1,1,1,
1,4),(84.8230016469245,85.4759697798722,86.4740905492242,87.4722113185763,
88.4703320879284,89.4684528572805,90.4665736266326,91.106186954104),
 .UNSPECIFIED.);
#1118=B_SPLINE_CURVE_WITH_KNOTS('',3,(#28365,#28366,#28367,#28368,#28369,
#28370,#28371,#28372,#28373,#28374),.UNSPECIFIED.,.F.,.F.,(4,1,1,1,1,1,
1,4),(84.8230016469245,85.1627767925112,86.1608975618633,87.1590183312153,
88.1571391005674,89.1552598699195,90.1533806392716,91.106186954104),
 .UNSPECIFIED.);
#1119=B_SPLINE_CURVE_WITH_KNOTS('',3,(#28379,#28380,#28381,#28382,#28383,
#28384,#28385,#28386,#28387,#28388),.UNSPECIFIED.,.F.,.F.,(4,1,1,1,1,1,
1,4),(78.5398163397449,79.4872451637597,80.4853659331118,81.4834867024638,
82.4816074718159,83.479728241168,84.4778490105201,84.8230016469245),
 .UNSPECIFIED.);
#1120=B_SPLINE_CURVE_WITH_KNOTS('',3,(#28389,#28390,#28391,#28392,#28393,
#28394,#28395,#28396,#28397,#28398),.UNSPECIFIED.,.F.,.F.,(4,1,1,1,1,1,
1,4),(78.5398163397449,79.1740521763987,80.1721729457508,81.1702937151029,
82.1684144844549,83.166535253807,84.1646560231591,84.8230016469245),
 .UNSPECIFIED.);
#1121=B_SPLINE_CURVE_WITH_KNOTS('',3,(#28403,#28404,#28405,#28406,#28407,
#28408,#28409,#28410,#28411,#28412,#28413),.UNSPECIFIED.,.F.,.F.,(4,1,1,
1,1,1,1,1,4),(72.2566310325653,72.5003997782951,73.4985205476472,74.4966413169993,
75.4947620863514,76.4928828557034,77.4910036250555,78.4891243944076,78.5398163397449),
 .UNSPECIFIED.);
#1122=B_SPLINE_CURVE_WITH_KNOTS('',3,(#28414,#28415,#28416,#28417,#28418,
#28419,#28420,#28421,#28422,#28423),.UNSPECIFIED.,.F.,.F.,(4,1,1,1,1,1,
1,4),(72.2566310325653,73.1853275602862,74.1834483296383,75.1815690989904,
76.1796898683425,77.1778106376945,78.1759314070466,78.5398163397449),
 .UNSPECIFIED.);
#1123=B_SPLINE_CURVE_WITH_KNOTS('',3,(#28428,#28429,#28430,#28431,#28432,
#28433,#28434,#28435,#28436,#28437),.UNSPECIFIED.,.F.,.F.,(4,1,1,1,1,1,
1,4),(65.9734457253857,66.5116751621827,67.5097959315347,68.5079167008868,
69.5060374702389,70.504158239591,71.502279008943,72.2566310325653),
 .UNSPECIFIED.);
#1124=B_SPLINE_CURVE_WITH_KNOTS('',3,(#28438,#28439,#28440,#28441,#28442,
#28443,#28444,#28445,#28446,#28447,#28448),.UNSPECIFIED.,.F.,.F.,(4,1,1,
1,1,1,1,1,4),(65.9734457253857,66.1984821748217,67.1966029441738,68.1947237135258,
69.1928444828779,70.19096525223,71.1890860215821,72.1872067909342,72.2566310325653),
 .UNSPECIFIED.);
#1125=B_SPLINE_CURVE_WITH_KNOTS('',3,(#28453,#28454,#28455,#28456,#28457,
#28458,#28459,#28460,#28461,#28462),.UNSPECIFIED.,.F.,.F.,(4,1,1,1,1,1,
1,4),(59.6902604182061,60.5229505460702,61.5210713154223,62.5191920847743,
63.5173128541264,64.5154336234785,65.5135543928306,65.9734457253857),
 .UNSPECIFIED.);
#1126=B_SPLINE_CURVE_WITH_KNOTS('',3,(#28463,#28464,#28465,#28466,#28467,
#28468,#28469,#28470,#28471,#28472),.UNSPECIFIED.,.F.,.F.,(4,1,1,1,1,1,
1,4),(59.6902604182061,60.2097575587092,61.2078783280613,62.2059990974134,
63.2041198667654,64.2022406361175,65.2003614054696,65.9734457253857),
 .UNSPECIFIED.);
#1127=B_SPLINE_CURVE_WITH_KNOTS('',3,(#28477,#28478,#28479,#28480,#28481,
#28482,#28483,#28484,#28485,#28486,#28487),.UNSPECIFIED.,.F.,.F.,(4,1,1,
1,1,1,1,1,4),(53.4070751110265,53.5361051606056,54.5342259299577,55.5323466993098,
56.5304674686619,57.528588238014,58.526709007366,59.5248297767181,59.6902604182061),
 .UNSPECIFIED.);
#1128=B_SPLINE_CURVE_WITH_KNOTS('',3,(#28488,#28489,#28490,#28491,#28492,
#28493,#28494,#28495,#28496,#28497),.UNSPECIFIED.,.F.,.F.,(4,1,1,1,1,1,
1,4),(53.4070751110265,54.2210329425967,55.2191537119488,56.2172744813009,
57.215395250653,58.213516020005,59.2116367893571,59.6902604182061),
 .UNSPECIFIED.);
#1129=B_SPLINE_CURVE_WITH_KNOTS('',3,(#28502,#28503,#28504,#28505,#28506,
#28507,#28508,#28509,#28510,#28511),.UNSPECIFIED.,.F.,.F.,(4,1,1,1,1,1,
1,4),(47.1238898038469,47.5473805444932,48.5455013138453,49.5436220831973,
50.5417428525494,51.5398636219015,52.5379843912536,53.4070751110265),
 .UNSPECIFIED.);
#1130=B_SPLINE_CURVE_WITH_KNOTS('',3,(#28512,#28513,#28514,#28515,#28516,
#28517,#28518,#28519,#28520,#28521,#28522),.UNSPECIFIED.,.F.,.F.,(4,1,1,
1,1,1,1,1,4),(47.1238898038469,47.2341875571322,48.2323083264843,49.2304290958363,
50.2285498651884,51.2266706345405,52.2247914038926,53.2229121732447,53.4070751110265),
 .UNSPECIFIED.);
#1131=B_SPLINE_CURVE_WITH_KNOTS('',3,(#28527,#28528,#28529,#28530,#28531,
#28532,#28533,#28534,#28535,#28536),.UNSPECIFIED.,.F.,.F.,(4,1,1,1,1,1,
1,4),(40.8407044966673,41.5586559283807,42.5567766977328,43.5548974670848,
44.5530182364369,45.551139005789,46.5492597751411,47.1238898038469),
 .UNSPECIFIED.);
#1132=B_SPLINE_CURVE_WITH_KNOTS('',3,(#28537,#28538,#28539,#28540,#28541,
#28542,#28543,#28544,#28545,#28546),.UNSPECIFIED.,.F.,.F.,(4,1,1,1,1,1,
1,4),(40.8407044966673,41.2454629410197,42.2435837103718,43.2417044797239,
44.2398252490759,45.237946018428,46.2360667877801,47.1238898038469),
 .UNSPECIFIED.);
#1133=B_SPLINE_CURVE_WITH_KNOTS('',3,(#28551,#28552,#28553,#28554,#28555,
#28556,#28557,#28558,#28559,#28560,#28561),.UNSPECIFIED.,.F.,.F.,(4,1,1,
1,1,1,1,1,4),(34.5575191894877,34.5718105429161,35.5699313122682,36.5680520816203,
37.5661728509724,38.5642936203245,39.5624143896765,40.5605351590286,40.8407044966673),
 .UNSPECIFIED.);
#1134=B_SPLINE_CURVE_WITH_KNOTS('',3,(#28562,#28563,#28564,#28565,#28566,
#28567,#28568,#28569,#28570,#28571),.UNSPECIFIED.,.F.,.F.,(4,1,1,1,1,1,
1,4),(34.5575191894877,35.2567383249072,36.2548590942593,37.2529798636114,
38.2511006329635,39.2492214023156,40.2473421716676,40.8407044966673),
 .UNSPECIFIED.);
#1135=B_SPLINE_CURVE_WITH_KNOTS('',3,(#28576,#28577,#28578,#28579,#28580,
#28581,#28582,#28583,#28584,#28585),.UNSPECIFIED.,.F.,.F.,(4,1,1,1,1,1,
1,4),(28.2743338823081,28.5830859268037,29.5812066961557,30.5793274655078,
31.5774482348599,32.575569004212,33.5736897735641,34.5575191894877),
 .UNSPECIFIED.);
#1136=B_SPLINE_CURVE_WITH_KNOTS('',3,(#28586,#28587,#28588,#28589,#28590,
#28591,#28592,#28593,#28594,#28595),.UNSPECIFIED.,.F.,.F.,(4,1,1,1,1,1,
1,4),(28.2743338823081,29.2680137087948,30.2661344781468,31.2642552474989,
32.262376016851,33.2604967862031,34.2586175555552,34.5575191894877),
 .UNSPECIFIED.);
#1137=B_SPLINE_CURVE_WITH_KNOTS('',3,(#28600,#28601,#28602,#28603,#28604,
#28605,#28606,#28607,#28608,#28609),.UNSPECIFIED.,.F.,.F.,(4,1,1,1,1,1,
1,4),(21.9911485751285,22.5943613106912,23.5924820800433,24.5906028493954,
25.5887236187474,26.5868443880995,27.5849651574516,28.2743338823081),
 .UNSPECIFIED.);
#1138=B_SPLINE_CURVE_WITH_KNOTS('',3,(#28610,#28611,#28612,#28613,#28614,
#28615,#28616,#28617,#28618,#28619,#28620),.UNSPECIFIED.,.F.,.F.,(4,1,1,
1,1,1,1,1,4),(21.9911485751285,22.2811683233302,23.2792890926823,24.2774098620344,
25.2755306313865,26.2736514007385,27.2717721700906,28.2698929394427,28.2743338823081),
 .UNSPECIFIED.);
#1139=B_SPLINE_CURVE_WITH_KNOTS('',3,(#28625,#28626,#28627,#28628,#28629,
#28630,#28631,#28632,#28633,#28634),.UNSPECIFIED.,.F.,.F.,(4,1,1,1,1,1,
1,4),(15.707963267949,16.6056366945787,17.6037574639308,18.6018782332829,
19.599999002635,20.598119771987,21.5962405413391,21.9911485751285),
 .UNSPECIFIED.);
#1140=B_SPLINE_CURVE_WITH_KNOTS('',3,(#28635,#28636,#28637,#28638,#28639,
#28640,#28641,#28642,#28643,#28644),.UNSPECIFIED.,.F.,.F.,(4,1,1,1,1,1,
1,4),(15.707963267949,16.2924437072177,17.2905644765698,18.2886852459219,
19.286806015274,20.2849267846261,21.2830475539781,21.9911485751285),
 .UNSPECIFIED.);
#1141=B_SPLINE_CURVE_WITH_KNOTS('',3,(#29262,#29263,#29264,#29265,#29266,
#29267,#29268,#29269,#29270,#29271,#29272,#29273,#29274,#29275,#29276,#29277,
#29278,#29279,#29280,#29281,#29282,#29283,#29284,#29285,#29286,#29287,#29288,
#29289,#29290,#29291,#29292,#29293,#29294,#29295,#29296,#29297,#29298,#29299,
#29300,#29301,#29302,#29303,#29304,#29305,#29306,#29307,#29308,#29309,#29310,
#29311,#29312,#29313,#29314,#29315,#29316,#29317,#29318,#29319),
 .UNSPECIFIED.,.F.,.F.,(4,3,3,3,3,3,3,3,3,3,3,3,3,3,3,3,3,3,3,4),(-0.552745378375043,
-0.531489243744843,-0.495108433985232,-0.477867666908701,-0.459926783852948,
-0.40834015484357,-0.390564261242345,-0.340650422189222,-0.308207347384289,
-0.294851172015872,-0.28154967607649,-0.252476072145833,-0.202914686431521,
-0.190042837184204,-0.142532127888153,-0.10590131786763,-0.092666137023641,
-0.0463330685118205,-0.0028441867201021,0.),.UNSPECIFIED.);
#1142=B_SPLINE_CURVE_WITH_KNOTS('',3,(#29320,#29321,#29322,#29323,#29324,
#29325,#29326,#29327,#29328,#29329,#29330,#29331,#29332),.UNSPECIFIED.,
 .F.,.F.,(4,3,3,3,4),(145.630562473499,145.725632325403,146.723753094756,
147.721873864108,148.647597997255),.UNSPECIFIED.);
#1143=B_SPLINE_CURVE_WITH_KNOTS('',3,(#29334,#29335,#29336,#29337,#29338,
#29339,#29340,#29341,#29342,#29343,#29344,#29345,#29346,#29347,#29348,#29349,
#29350,#29351,#29352,#29353,#29354,#29355,#29356,#29357,#29358,#29359,#29360,
#29361,#29362,#29363,#29364,#29365,#29366,#29367,#29368,#29369,#29370,#29371,
#29372,#29373,#29374,#29375,#29376,#29377,#29378,#29379,#29380,#29381,#29382,
#29383,#29384,#29385,#29386,#29387,#29388),.UNSPECIFIED.,.F.,.F.,(4,3,3,
3,3,3,3,3,3,3,3,3,3,3,3,3,3,3,4),(-0.555272788399391,-0.537829475145404,
-0.501151444327474,-0.480433685752521,-0.449607979278525,-0.430089933902533,
-0.415584630121194,-0.367513977288793,-0.334452546673387,-0.315854971100898,
-0.282472195537201,-0.247163171095051,-0.224831098912879,-0.211454760083625,
-0.161528020768348,-0.11601494941692,-0.102547348706884,-0.050144009897631,
0.),.UNSPECIFIED.);
#1144=B_SPLINE_CURVE_WITH_KNOTS('',3,(#29389,#29390,#29391,#29392,#29393,
#29394,#29395,#29396,#29397),.UNSPECIFIED.,.F.,.F.,(4,1,1,1,1,1,4),(10.3761157273103,
11.3018398604573,12.2999606298094,13.2980813991615,14.2962021685136,15.2943229378657,
15.707963267949),.UNSPECIFIED.);
#1145=B_SPLINE_CURVE_WITH_KNOTS('',3,(#29403,#29404,#29405,#29406,#29407,
#29408,#29409,#29410,#29411,#29412,#29413,#29414,#29415,#29416,#29417,#29418,
#29419,#29420,#29421,#29422,#29423,#29424,#29425,#29426,#29427,#29428,#29429,
#29430,#29431,#29432,#29433,#29434,#29435,#29436,#29437,#29438,#29439,#29440,
#29441,#29442,#29443,#29444,#29445,#29446,#29447,#29448,#29449,#29450,#29451,
#29452,#29453,#29454,#29455,#29456,#29457,#29458,#29459,#29460),
 .UNSPECIFIED.,.F.,.F.,(4,3,3,3,3,3,3,3,3,3,3,3,3,3,3,3,3,3,3,4),(-0.552745378375056,
-0.531489243744835,-0.495108428311827,-0.477867651520537,-0.45992677828748,
-0.408340146860344,-0.39056425606813,-0.34065040901948,-0.308207314423746,
-0.294851132888488,-0.28154966653563,-0.252476072145832,-0.202914855082696,
-0.190043155762275,-0.142532366821707,-0.105901640544872,-0.0926664448836297,
-0.0463332224418149,-0.00284436592965125,0.),.UNSPECIFIED.);
#1146=B_SPLINE_CURVE_WITH_KNOTS('',3,(#29463,#29464,#29465,#29466,#29467,
#29468,#29469,#29470),.UNSPECIFIED.,.F.,.F.,(4,1,1,1,1,4),(11.6150328478183,
12.6131536171704,13.6112743865225,14.6093951558746,15.6075159252266,15.707963267949),
 .UNSPECIFIED.);
#1147=B_SPLINE_CURVE_WITH_KNOTS('',3,(#30088,#30089,#30090,#30091,#30092,
#30093,#30094,#30095,#30096,#30097,#30098,#30099,#30100,#30101,#30102,#30103,
#30104,#30105,#30106,#30107,#30108,#30109,#30110,#30111,#30112,#30113,#30114,
#30115,#30116,#30117,#30118,#30119,#30120,#30121,#30122,#30123,#30124,#30125,
#30126,#30127,#30128,#30129,#30130,#30131,#30132,#30133,#30134,#30135,#30136,
#30137,#30138,#30139,#30140,#30141,#30142),.UNSPECIFIED.,.F.,.F.,(4,3,3,
3,3,3,3,3,3,3,3,3,3,3,3,3,3,3,4),(-0.55527278839943,-0.537829475145452,
-0.501151443157722,-0.480433683572202,-0.449608208717037,-0.430090720039549,
-0.415584982436066,-0.367514333548957,-0.334452908269952,-0.315854921314816,
-0.282472195537241,-0.247163171095086,-0.224831104408066,-0.211454765807094,
-0.161528018350323,-0.116014945472013,-0.102547346883912,-0.0501440159489521,
0.),.UNSPECIFIED.);
#1148=B_SPLINE_CURVE_WITH_KNOTS('',3,(#30143,#30144,#30145,#30146,#30147,
#30148,#30149,#30150,#30151,#30152),.UNSPECIFIED.,.F.,.F.,(4,3,3,4),(-150.716236172164,
-149.718115402812,-148.71999463346,-148.606192485261),.UNSPECIFIED.);
#1332=B_SPLINE_SURFACE_WITH_KNOTS('',3,3,((#28645,#28646,#28647,#28648,
#28649,#28650,#28651,#28652,#28653,#28654,#28655,#28656,#28657,#28658,#28659,
#28660,#28661,#28662,#28663,#28664,#28665,#28666,#28667,#28668,#28669,#28670,
#28671,#28672,#28673,#28674,#28675,#28676,#28677,#28678,#28679,#28680,#28681,
#28682,#28683,#28684,#28685,#28686,#28687,#28688,#28689,#28690,#28691,#28692,
#28693,#28694,#28695,#28696,#28697,#28698,#28699,#28700,#28701,#28702,#28703,
#28704,#28705,#28706,#28707,#28708,#28709,#28710,#28711,#28712,#28713,#28714,
#28715,#28716,#28717,#28718,#28719,#28720,#28721,#28722,#28723,#28724,#28725,
#28726,#28727,#28728,#28729,#28730,#28731,#28732,#28733,#28734,#28735,#28736,
#28737,#28738,#28739,#28740,#28741,#28742,#28743,#28744,#28745,#28746,#28747,
#28748,#28749,#28750,#28751,#28752,#28753,#28754,#28755,#28756,#28757,#28758,
#28759,#28760,#28761,#28762,#28763,#28764,#28765,#28766,#28767,#28768,#28769,
#28770,#28771,#28772,#28773,#28774,#28775,#28776,#28777,#28778,#28779,#28780,
#28781,#28782,#28783,#28784,#28785,#28786,#28787,#28788,#28789,#28790,#28791,
#28792,#28793,#28794,#28795,#28796,#28797,#28798),(#28799,#28800,#28801,
#28802,#28803,#28804,#28805,#28806,#28807,#28808,#28809,#28810,#28811,#28812,
#28813,#28814,#28815,#28816,#28817,#28818,#28819,#28820,#28821,#28822,#28823,
#28824,#28825,#28826,#28827,#28828,#28829,#28830,#28831,#28832,#28833,#28834,
#28835,#28836,#28837,#28838,#28839,#28840,#28841,#28842,#28843,#28844,#28845,
#28846,#28847,#28848,#28849,#28850,#28851,#28852,#28853,#28854,#28855,#28856,
#28857,#28858,#28859,#28860,#28861,#28862,#28863,#28864,#28865,#28866,#28867,
#28868,#28869,#28870,#28871,#28872,#28873,#28874,#28875,#28876,#28877,#28878,
#28879,#28880,#28881,#28882,#28883,#28884,#28885,#28886,#28887,#28888,#28889,
#28890,#28891,#28892,#28893,#28894,#28895,#28896,#28897,#28898,#28899,#28900,
#28901,#28902,#28903,#28904,#28905,#28906,#28907,#28908,#28909,#28910,#28911,
#28912,#28913,#28914,#28915,#28916,#28917,#28918,#28919,#28920,#28921,#28922,
#28923,#28924,#28925,#28926,#28927,#28928,#28929,#28930,#28931,#28932,#28933,
#28934,#28935,#28936,#28937,#28938,#28939,#28940,#28941,#28942,#28943,#28944,
#28945,#28946,#28947,#28948,#28949,#28950,#28951,#28952),(#28953,#28954,
#28955,#28956,#28957,#28958,#28959,#28960,#28961,#28962,#28963,#28964,#28965,
#28966,#28967,#28968,#28969,#28970,#28971,#28972,#28973,#28974,#28975,#28976,
#28977,#28978,#28979,#28980,#28981,#28982,#28983,#28984,#28985,#28986,#28987,
#28988,#28989,#28990,#28991,#28992,#28993,#28994,#28995,#28996,#28997,#28998,
#28999,#29000,#29001,#29002,#29003,#29004,#29005,#29006,#29007,#29008,#29009,
#29010,#29011,#29012,#29013,#29014,#29015,#29016,#29017,#29018,#29019,#29020,
#29021,#29022,#29023,#29024,#29025,#29026,#29027,#29028,#29029,#29030,#29031,
#29032,#29033,#29034,#29035,#29036,#29037,#29038,#29039,#29040,#29041,#29042,
#29043,#29044,#29045,#29046,#29047,#29048,#29049,#29050,#29051,#29052,#29053,
#29054,#29055,#29056,#29057,#29058,#29059,#29060,#29061,#29062,#29063,#29064,
#29065,#29066,#29067,#29068,#29069,#29070,#29071,#29072,#29073,#29074,#29075,
#29076,#29077,#29078,#29079,#29080,#29081,#29082,#29083,#29084,#29085,#29086,
#29087,#29088,#29089,#29090,#29091,#29092,#29093,#29094,#29095,#29096,#29097,
#29098,#29099,#29100,#29101,#29102,#29103,#29104,#29105,#29106),(#29107,
#29108,#29109,#29110,#29111,#29112,#29113,#29114,#29115,#29116,#29117,#29118,
#29119,#29120,#29121,#29122,#29123,#29124,#29125,#29126,#29127,#29128,#29129,
#29130,#29131,#29132,#29133,#29134,#29135,#29136,#29137,#29138,#29139,#29140,
#29141,#29142,#29143,#29144,#29145,#29146,#29147,#29148,#29149,#29150,#29151,
#29152,#29153,#29154,#29155,#29156,#29157,#29158,#29159,#29160,#29161,#29162,
#29163,#29164,#29165,#29166,#29167,#29168,#29169,#29170,#29171,#29172,#29173,
#29174,#29175,#29176,#29177,#29178,#29179,#29180,#29181,#29182,#29183,#29184,
#29185,#29186,#29187,#29188,#29189,#29190,#29191,#29192,#29193,#29194,#29195,
#29196,#29197,#29198,#29199,#29200,#29201,#29202,#29203,#29204,#29205,#29206,
#29207,#29208,#29209,#29210,#29211,#29212,#29213,#29214,#29215,#29216,#29217,
#29218,#29219,#29220,#29221,#29222,#29223,#29224,#29225,#29226,#29227,#29228,
#29229,#29230,#29231,#29232,#29233,#29234,#29235,#29236,#29237,#29238,#29239,
#29240,#29241,#29242,#29243,#29244,#29245,#29246,#29247,#29248,#29249,#29250,
#29251,#29252,#29253,#29254,#29255,#29256,#29257,#29258,#29259,#29260)),
 .UNSPECIFIED.,.F.,.F.,.F.,(4,4),(4,1,1,1,1,1,1,1,1,1,1,1,1,1,1,1,1,1,1,
1,1,1,1,1,1,1,1,1,1,1,1,1,1,1,1,1,1,1,1,1,1,1,1,1,1,1,1,1,1,1,1,1,1,1,1,
1,1,1,1,1,1,1,1,1,1,1,1,1,1,1,1,1,1,1,1,1,1,1,1,1,1,1,1,1,1,1,1,1,1,1,1,
1,1,1,1,1,1,1,1,1,1,1,1,1,1,1,1,1,1,1,1,1,1,1,1,1,1,1,1,1,1,1,1,1,1,1,1,
1,1,1,1,1,1,1,1,1,1,1,1,1,1,1,1,1,1,1,1,1,1,1,1,4),(0.,0.0658467982010769),
(8.30747755240111,9.30559832175319,10.3037190911053,11.3018398604573,12.2999606298094,
13.2980813991615,14.2962021685136,15.2943229378657,16.2924437072177,17.2905644765698,
18.2886852459219,19.286806015274,20.2849267846261,21.2830475539781,22.2811683233302,
23.2792890926823,24.2774098620344,25.2755306313865,26.2736514007385,27.2717721700906,
28.2698929394427,29.2680137087948,30.2661344781468,31.2642552474989,32.262376016851,
33.2604967862031,34.2586175555552,35.2567383249072,36.2548590942593,37.2529798636114,
38.2511006329635,39.2492214023156,40.2473421716676,41.2454629410197,42.2435837103718,
43.2417044797239,44.2398252490759,45.237946018428,46.2360667877801,47.2341875571322,
48.2323083264843,49.2304290958363,50.2285498651884,51.2266706345405,52.2247914038926,
53.2229121732447,54.2210329425967,55.2191537119488,56.2172744813009,57.215395250653,
58.213516020005,59.2116367893571,60.2097575587092,61.2078783280613,62.2059990974134,
63.2041198667654,64.2022406361175,65.2003614054696,66.1984821748217,67.1966029441738,
68.1947237135258,69.1928444828779,70.19096525223,71.1890860215821,72.1872067909342,
73.1853275602862,74.1834483296383,75.1815690989904,76.1796898683425,77.1778106376945,
78.1759314070466,79.1740521763987,80.1721729457508,81.1702937151029,82.1684144844549,
83.166535253807,84.1646560231591,85.1627767925112,86.1608975618633,87.1590183312153,
88.1571391005674,89.1552598699195,90.1533806392716,91.1515014086236,92.1496221779757,
93.1477429473278,94.1458637166799,95.143984486032,96.142105255384,97.1402260247361,
98.1383467940882,99.1364675634403,100.134588332792,101.132709102144,102.130829871497,
103.128950640849,104.127071410201,105.125192179553,106.123312948905,107.121433718257,
108.119554487609,109.117675256961,110.115796026313,111.113916795665,112.112037565017,
113.110158334369,114.108279103721,115.106399873074,116.104520642426,117.102641411778,
118.10076218113,119.098882950482,120.097003719834,121.095124489186,122.093245258538,
123.09136602789,124.089486797242,125.087607566594,126.085728335946,127.083849105298,
128.081969874651,129.080090644003,130.078211413355,131.076332182707,132.074452952059,
133.072573721411,134.070694490763,135.068815260115,136.066936029467,137.065056798819,
138.063177568171,139.061298337523,140.059419106876,141.057539876228,142.05566064558,
143.053781414932,144.051902184284,145.050022953636,146.048143722988,147.04626449234,
148.044385261692,149.042506031044,150.040626800396,151.038747569748,152.0368683391,
153.034989108453,154.033109877805,155.031230647157,156.029351416509,157.027472185861,
158.025592955213,159.023713724565),.UNSPECIFIED.);
#1333=B_SPLINE_SURFACE_WITH_KNOTS('',3,3,((#29471,#29472,#29473,#29474,
#29475,#29476,#29477,#29478,#29479,#29480,#29481,#29482,#29483,#29484,#29485,
#29486,#29487,#29488,#29489,#29490,#29491,#29492,#29493,#29494,#29495,#29496,
#29497,#29498,#29499,#29500,#29501,#29502,#29503,#29504,#29505,#29506,#29507,
#29508,#29509,#29510,#29511,#29512,#29513,#29514,#29515,#29516,#29517,#29518,
#29519,#29520,#29521,#29522,#29523,#29524,#29525,#29526,#29527,#29528,#29529,
#29530,#29531,#29532,#29533,#29534,#29535,#29536,#29537,#29538,#29539,#29540,
#29541,#29542,#29543,#29544,#29545,#29546,#29547,#29548,#29549,#29550,#29551,
#29552,#29553,#29554,#29555,#29556,#29557,#29558,#29559,#29560,#29561,#29562,
#29563,#29564,#29565,#29566,#29567,#29568,#29569,#29570,#29571,#29572,#29573,
#29574,#29575,#29576,#29577,#29578,#29579,#29580,#29581,#29582,#29583,#29584,
#29585,#29586,#29587,#29588,#29589,#29590,#29591,#29592,#29593,#29594,#29595,
#29596,#29597,#29598,#29599,#29600,#29601,#29602,#29603,#29604,#29605,#29606,
#29607,#29608,#29609,#29610,#29611,#29612,#29613,#29614,#29615,#29616,#29617,
#29618,#29619,#29620,#29621,#29622,#29623,#29624),(#29625,#29626,#29627,
#29628,#29629,#29630,#29631,#29632,#29633,#29634,#29635,#29636,#29637,#29638,
#29639,#29640,#29641,#29642,#29643,#29644,#29645,#29646,#29647,#29648,#29649,
#29650,#29651,#29652,#29653,#29654,#29655,#29656,#29657,#29658,#29659,#29660,
#29661,#29662,#29663,#29664,#29665,#29666,#29667,#29668,#29669,#29670,#29671,
#29672,#29673,#29674,#29675,#29676,#29677,#29678,#29679,#29680,#29681,#29682,
#29683,#29684,#29685,#29686,#29687,#29688,#29689,#29690,#29691,#29692,#29693,
#29694,#29695,#29696,#29697,#29698,#29699,#29700,#29701,#29702,#29703,#29704,
#29705,#29706,#29707,#29708,#29709,#29710,#29711,#29712,#29713,#29714,#29715,
#29716,#29717,#29718,#29719,#29720,#29721,#29722,#29723,#29724,#29725,#29726,
#29727,#29728,#29729,#29730,#29731,#29732,#29733,#29734,#29735,#29736,#29737,
#29738,#29739,#29740,#29741,#29742,#29743,#29744,#29745,#29746,#29747,#29748,
#29749,#29750,#29751,#29752,#29753,#29754,#29755,#29756,#29757,#29758,#29759,
#29760,#29761,#29762,#29763,#29764,#29765,#29766,#29767,#29768,#29769,#29770,
#29771,#29772,#29773,#29774,#29775,#29776,#29777,#29778),(#29779,#29780,
#29781,#29782,#29783,#29784,#29785,#29786,#29787,#29788,#29789,#29790,#29791,
#29792,#29793,#29794,#29795,#29796,#29797,#29798,#29799,#29800,#29801,#29802,
#29803,#29804,#29805,#29806,#29807,#29808,#29809,#29810,#29811,#29812,#29813,
#29814,#29815,#29816,#29817,#29818,#29819,#29820,#29821,#29822,#29823,#29824,
#29825,#29826,#29827,#29828,#29829,#29830,#29831,#29832,#29833,#29834,#29835,
#29836,#29837,#29838,#29839,#29840,#29841,#29842,#29843,#29844,#29845,#29846,
#29847,#29848,#29849,#29850,#29851,#29852,#29853,#29854,#29855,#29856,#29857,
#29858,#29859,#29860,#29861,#29862,#29863,#29864,#29865,#29866,#29867,#29868,
#29869,#29870,#29871,#29872,#29873,#29874,#29875,#29876,#29877,#29878,#29879,
#29880,#29881,#29882,#29883,#29884,#29885,#29886,#29887,#29888,#29889,#29890,
#29891,#29892,#29893,#29894,#29895,#29896,#29897,#29898,#29899,#29900,#29901,
#29902,#29903,#29904,#29905,#29906,#29907,#29908,#29909,#29910,#29911,#29912,
#29913,#29914,#29915,#29916,#29917,#29918,#29919,#29920,#29921,#29922,#29923,
#29924,#29925,#29926,#29927,#29928,#29929,#29930,#29931,#29932),(#29933,
#29934,#29935,#29936,#29937,#29938,#29939,#29940,#29941,#29942,#29943,#29944,
#29945,#29946,#29947,#29948,#29949,#29950,#29951,#29952,#29953,#29954,#29955,
#29956,#29957,#29958,#29959,#29960,#29961,#29962,#29963,#29964,#29965,#29966,
#29967,#29968,#29969,#29970,#29971,#29972,#29973,#29974,#29975,#29976,#29977,
#29978,#29979,#29980,#29981,#29982,#29983,#29984,#29985,#29986,#29987,#29988,
#29989,#29990,#29991,#29992,#29993,#29994,#29995,#29996,#29997,#29998,#29999,
#30000,#30001,#30002,#30003,#30004,#30005,#30006,#30007,#30008,#30009,#30010,
#30011,#30012,#30013,#30014,#30015,#30016,#30017,#30018,#30019,#30020,#30021,
#30022,#30023,#30024,#30025,#30026,#30027,#30028,#30029,#30030,#30031,#30032,
#30033,#30034,#30035,#30036,#30037,#30038,#30039,#30040,#30041,#30042,#30043,
#30044,#30045,#30046,#30047,#30048,#30049,#30050,#30051,#30052,#30053,#30054,
#30055,#30056,#30057,#30058,#30059,#30060,#30061,#30062,#30063,#30064,#30065,
#30066,#30067,#30068,#30069,#30070,#30071,#30072,#30073,#30074,#30075,#30076,
#30077,#30078,#30079,#30080,#30081,#30082,#30083,#30084,#30085,#30086)),
 .UNSPECIFIED.,.F.,.F.,.F.,(4,4),(4,1,1,1,1,1,1,1,1,1,1,1,1,1,1,1,1,1,1,
1,1,1,1,1,1,1,1,1,1,1,1,1,1,1,1,1,1,1,1,1,1,1,1,1,1,1,1,1,1,1,1,1,1,1,1,
1,1,1,1,1,1,1,1,1,1,1,1,1,1,1,1,1,1,1,1,1,1,1,1,1,1,1,1,1,1,1,1,1,1,1,1,
1,1,1,1,1,1,1,1,1,1,1,1,1,1,1,1,1,1,1,1,1,1,1,1,1,1,1,1,1,1,1,1,1,1,1,1,
1,1,1,1,1,1,1,1,1,1,1,1,1,1,1,1,1,1,1,1,1,1,1,1,4),(0.,0.0658467982010769),
(11.6150328478183,12.6131536171704,13.6112743865225,14.6093951558746,15.6075159252266,
16.6056366945787,17.6037574639308,18.6018782332829,19.599999002635,20.598119771987,
21.5962405413391,22.5943613106912,23.5924820800433,24.5906028493954,25.5887236187474,
26.5868443880995,27.5849651574516,28.5830859268037,29.5812066961557,30.5793274655078,
31.5774482348599,32.575569004212,33.5736897735641,34.5718105429161,35.5699313122682,
36.5680520816203,37.5661728509724,38.5642936203245,39.5624143896765,40.5605351590286,
41.5586559283807,42.5567766977328,43.5548974670848,44.5530182364369,45.551139005789,
46.5492597751411,47.5473805444932,48.5455013138453,49.5436220831973,50.5417428525494,
51.5398636219015,52.5379843912536,53.5361051606056,54.5342259299577,55.5323466993098,
56.5304674686619,57.528588238014,58.526709007366,59.5248297767181,60.5229505460702,
61.5210713154223,62.5191920847743,63.5173128541264,64.5154336234785,65.5135543928306,
66.5116751621827,67.5097959315347,68.5079167008868,69.5060374702389,70.504158239591,
71.502279008943,72.5003997782951,73.4985205476472,74.4966413169993,75.4947620863514,
76.4928828557034,77.4910036250555,78.4891243944076,79.4872451637597,80.4853659331118,
81.4834867024638,82.4816074718159,83.479728241168,84.4778490105201,85.4759697798722,
86.4740905492242,87.4722113185763,88.4703320879284,89.4684528572805,90.4665736266326,
91.4646943959846,92.4628151653367,93.4609359346888,94.4590567040409,95.4571774733929,
96.455298242745,97.4534190120971,98.4515397814492,99.4496605508013,100.447781320153,
101.445902089505,102.444022858857,103.44214362821,104.440264397562,105.438385166914,
106.436505936266,107.434626705618,108.43274747497,109.430868244322,110.428989013674,
111.427109783026,112.425230552378,113.42335132173,114.421472091082,115.419592860435,
116.417713629787,117.415834399139,118.413955168491,119.412075937843,120.410196707195,
121.408317476547,122.406438245899,123.404559015251,124.402679784603,125.400800553955,
126.398921323307,127.397042092659,128.395162862012,129.393283631364,130.391404400716,
131.389525170068,132.38764593942,133.385766708772,134.383887478124,135.382008247476,
136.380129016828,137.37824978618,138.376370555532,139.374491324884,140.372612094236,
141.370732863589,142.368853632941,143.366974402293,144.365095171645,145.363215940997,
146.361336710349,147.359457479701,148.357578249053,149.355699018405,150.353819787757,
151.351940557109,152.350061326461,153.348182095814,154.346302865166,155.344423634518,
156.34254440387,157.340665173222,158.338785942574,159.336906711926,160.335027481278,
161.33314825063,162.331269019982),.UNSPECIFIED.);
#1397=FACE_BOUND('',#3062,.T.);
#1398=FACE_BOUND('',#3210,.T.);
#1399=FACE_BOUND('',#3215,.T.);
#1400=FACE_BOUND('',#3220,.T.);
#1668=CIRCLE('',#13177,0.2942);
#1669=CIRCLE('',#13202,0.237175);
#1670=CIRCLE('',#13204,0.237175);
#1671=CIRCLE('',#13228,0.2942);
#1672=CIRCLE('',#13229,0.2942);
#1673=CIRCLE('',#13230,0.237175);
#1674=CIRCLE('',#13233,0.249992666559108);
#1675=CIRCLE('',#13243,0.5);
#1676=CIRCLE('',#13246,0.5);
#1677=CIRCLE('',#13249,0.5);
#1678=CIRCLE('',#13252,0.5);
#1679=CIRCLE('',#13255,0.5);
#1680=CIRCLE('',#13258,0.5);
#1681=CIRCLE('',#13261,0.5);
#1682=CIRCLE('',#13264,0.5);
#1683=CIRCLE('',#13267,0.5);
#1684=CIRCLE('',#13270,0.5);
#1685=CIRCLE('',#13273,0.5);
#1686=CIRCLE('',#13276,0.5);
#1687=CIRCLE('',#13279,0.5);
#1688=CIRCLE('',#13282,0.5);
#1689=CIRCLE('',#13285,0.5);
#1690=CIRCLE('',#13288,0.5);
#1691=CIRCLE('',#13291,0.5);
#1692=CIRCLE('',#13292,0.5);
#1693=CIRCLE('',#13295,0.5);
#1694=CIRCLE('',#13296,0.5);
#1695=CIRCLE('',#13299,0.5);
#1696=CIRCLE('',#13302,0.5);
#1697=CIRCLE('',#13305,0.5);
#1698=CIRCLE('',#13308,0.5);
#1699=CIRCLE('',#13311,0.5);
#1700=CIRCLE('',#13314,0.5);
#1701=CIRCLE('',#13317,0.5);
#1702=CIRCLE('',#13320,0.5);
#1703=CIRCLE('',#13323,0.5);
#1704=CIRCLE('',#13326,0.5);
#1705=CIRCLE('',#13329,0.5);
#1706=CIRCLE('',#13332,0.5);
#1707=CIRCLE('',#13335,0.5);
#1708=CIRCLE('',#13338,0.5);
#1709=CIRCLE('',#13341,0.5);
#1710=CIRCLE('',#13344,0.5);
#1711=CIRCLE('',#13347,0.5);
#1712=CIRCLE('',#13350,0.5);
#1713=CIRCLE('',#13353,0.5);
#1714=CIRCLE('',#13356,0.5);
#1715=CIRCLE('',#13359,0.5);
#1716=CIRCLE('',#13362,0.5);
#1717=CIRCLE('',#13365,0.5);
#1718=CIRCLE('',#13368,0.5);
#1719=CIRCLE('',#13371,0.5);
#1720=CIRCLE('',#13374,0.5);
#1721=CIRCLE('',#13377,0.5);
#1722=CIRCLE('',#13380,0.5);
#1723=CIRCLE('',#13383,0.5);
#1724=CIRCLE('',#13386,0.5);
#1725=CIRCLE('',#13389,0.5);
#1726=CIRCLE('',#13392,0.5);
#1727=CIRCLE('',#13395,0.5);
#1728=CIRCLE('',#13398,0.5);
#1729=CIRCLE('',#13400,0.5);
#1730=CIRCLE('',#13404,0.5);
#1731=CIRCLE('',#13407,0.5);
#1732=CIRCLE('',#13410,0.5);
#1733=CIRCLE('',#13413,0.5);
#1734=CIRCLE('',#13416,0.5);
#1735=CIRCLE('',#13419,0.5);
#1736=CIRCLE('',#13422,0.5);
#1737=CIRCLE('',#13425,0.5);
#1738=CIRCLE('',#13428,0.5);
#1739=CIRCLE('',#13431,0.5);
#1740=CIRCLE('',#13434,0.5);
#1741=CIRCLE('',#13437,0.5);
#1742=CIRCLE('',#13440,0.5);
#1743=CIRCLE('',#13443,0.5);
#1744=CIRCLE('',#13446,0.5);
#1745=CIRCLE('',#13449,0.5);
#1746=CIRCLE('',#13452,0.5);
#1747=CIRCLE('',#13455,0.5);
#1748=CIRCLE('',#13458,0.5);
#1749=CIRCLE('',#13460,0.298);
#1750=CIRCLE('',#13461,0.025);
#1751=CIRCLE('',#13462,0.323);
#1752=CIRCLE('',#13464,0.298);
#1753=CIRCLE('',#13466,0.48);
#1754=CIRCLE('',#13468,0.26);
#1755=CIRCLE('',#13471,0.2942);
#1756=CIRCLE('',#13474,0.5);
#1757=CIRCLE('',#13476,0.5);
#1758=CIRCLE('',#13477,0.5);
#1759=CIRCLE('',#13478,0.5);
#1760=CIRCLE('',#13479,0.5);
#1761=CIRCLE('',#13480,0.5);
#1762=CIRCLE('',#13481,0.5);
#1763=CIRCLE('',#13482,0.5);
#1764=CIRCLE('',#13483,0.5);
#1765=CIRCLE('',#13484,0.5);
#1766=CIRCLE('',#13485,0.5);
#1767=CIRCLE('',#13486,0.5);
#1768=CIRCLE('',#13487,0.5);
#1769=CIRCLE('',#13488,0.5);
#1770=CIRCLE('',#13489,0.5);
#1771=CIRCLE('',#13490,0.5);
#1772=CIRCLE('',#13491,0.5);
#1773=CIRCLE('',#13492,0.5);
#1774=CIRCLE('',#13493,0.5);
#1775=CIRCLE('',#13494,0.5);
#1776=CIRCLE('',#13495,0.5);
#1777=CIRCLE('',#13496,0.5);
#1778=CIRCLE('',#13497,0.5);
#1779=CIRCLE('',#13498,0.5);
#1780=CIRCLE('',#13499,0.5);
#1781=CIRCLE('',#13500,0.5);
#1782=CIRCLE('',#13501,0.5);
#1783=CIRCLE('',#13502,0.5);
#1784=CIRCLE('',#13503,0.5);
#1785=CIRCLE('',#13504,0.5);
#1786=CIRCLE('',#13505,0.5);
#1787=CIRCLE('',#13506,0.5);
#1788=CIRCLE('',#13507,0.5);
#1789=CIRCLE('',#13508,0.5);
#1790=CIRCLE('',#13509,0.5);
#1791=CIRCLE('',#13510,0.5);
#1792=CIRCLE('',#13511,0.5);
#1793=CIRCLE('',#13513,0.46);
#2251=FACE_OUTER_BOUND('',#3002,.T.);
#2252=FACE_OUTER_BOUND('',#3003,.T.);
#2253=FACE_OUTER_BOUND('',#3004,.T.);
#2254=FACE_OUTER_BOUND('',#3005,.T.);
#2255=FACE_OUTER_BOUND('',#3006,.T.);
#2256=FACE_OUTER_BOUND('',#3007,.T.);
#2257=FACE_OUTER_BOUND('',#3008,.T.);
#2258=FACE_OUTER_BOUND('',#3009,.T.);
#2259=FACE_OUTER_BOUND('',#3010,.T.);
#2260=FACE_OUTER_BOUND('',#3011,.T.);
#2261=FACE_OUTER_BOUND('',#3012,.T.);
#2262=FACE_OUTER_BOUND('',#3013,.T.);
#2263=FACE_OUTER_BOUND('',#3014,.T.);
#2264=FACE_OUTER_BOUND('',#3015,.T.);
#2265=FACE_OUTER_BOUND('',#3016,.T.);
#2266=FACE_OUTER_BOUND('',#3017,.T.);
#2267=FACE_OUTER_BOUND('',#3018,.T.);
#2268=FACE_OUTER_BOUND('',#3019,.T.);
#2269=FACE_OUTER_BOUND('',#3020,.T.);
#2270=FACE_OUTER_BOUND('',#3021,.T.);
#2271=FACE_OUTER_BOUND('',#3022,.T.);
#2272=FACE_OUTER_BOUND('',#3023,.T.);
#2273=FACE_OUTER_BOUND('',#3024,.T.);
#2274=FACE_OUTER_BOUND('',#3025,.T.);
#2275=FACE_OUTER_BOUND('',#3026,.T.);
#2276=FACE_OUTER_BOUND('',#3027,.T.);
#2277=FACE_OUTER_BOUND('',#3028,.T.);
#2278=FACE_OUTER_BOUND('',#3029,.T.);
#2279=FACE_OUTER_BOUND('',#3030,.T.);
#2280=FACE_OUTER_BOUND('',#3031,.T.);
#2281=FACE_OUTER_BOUND('',#3032,.T.);
#2282=FACE_OUTER_BOUND('',#3033,.T.);
#2283=FACE_OUTER_BOUND('',#3034,.T.);
#2284=FACE_OUTER_BOUND('',#3035,.T.);
#2285=FACE_OUTER_BOUND('',#3036,.T.);
#2286=FACE_OUTER_BOUND('',#3037,.T.);
#2287=FACE_OUTER_BOUND('',#3038,.T.);
#2288=FACE_OUTER_BOUND('',#3039,.T.);
#2289=FACE_OUTER_BOUND('',#3040,.T.);
#2290=FACE_OUTER_BOUND('',#3041,.T.);
#2291=FACE_OUTER_BOUND('',#3042,.T.);
#2292=FACE_OUTER_BOUND('',#3043,.T.);
#2293=FACE_OUTER_BOUND('',#3044,.T.);
#2294=FACE_OUTER_BOUND('',#3045,.T.);
#2295=FACE_OUTER_BOUND('',#3046,.T.);
#2296=FACE_OUTER_BOUND('',#3047,.T.);
#2297=FACE_OUTER_BOUND('',#3048,.T.);
#2298=FACE_OUTER_BOUND('',#3049,.T.);
#2299=FACE_OUTER_BOUND('',#3050,.T.);
#2300=FACE_OUTER_BOUND('',#3051,.T.);
#2301=FACE_OUTER_BOUND('',#3052,.T.);
#2302=FACE_OUTER_BOUND('',#3053,.T.);
#2303=FACE_OUTER_BOUND('',#3054,.T.);
#2304=FACE_OUTER_BOUND('',#3055,.T.);
#2305=FACE_OUTER_BOUND('',#3056,.T.);
#2306=FACE_OUTER_BOUND('',#3057,.T.);
#2307=FACE_OUTER_BOUND('',#3058,.T.);
#2308=FACE_OUTER_BOUND('',#3059,.T.);
#2309=FACE_OUTER_BOUND('',#3060,.T.);
#2310=FACE_OUTER_BOUND('',#3061,.T.);
#2311=FACE_OUTER_BOUND('',#3063,.T.);
#2312=FACE_OUTER_BOUND('',#3064,.T.);
#2313=FACE_OUTER_BOUND('',#3065,.T.);
#2314=FACE_OUTER_BOUND('',#3066,.T.);
#2315=FACE_OUTER_BOUND('',#3067,.T.);
#2316=FACE_OUTER_BOUND('',#3068,.T.);
#2317=FACE_OUTER_BOUND('',#3069,.T.);
#2318=FACE_OUTER_BOUND('',#3070,.T.);
#2319=FACE_OUTER_BOUND('',#3071,.T.);
#2320=FACE_OUTER_BOUND('',#3072,.T.);
#2321=FACE_OUTER_BOUND('',#3073,.T.);
#2322=FACE_OUTER_BOUND('',#3074,.T.);
#2323=FACE_OUTER_BOUND('',#3075,.T.);
#2324=FACE_OUTER_BOUND('',#3076,.T.);
#2325=FACE_OUTER_BOUND('',#3077,.T.);
#2326=FACE_OUTER_BOUND('',#3078,.T.);
#2327=FACE_OUTER_BOUND('',#3079,.T.);
#2328=FACE_OUTER_BOUND('',#3080,.T.);
#2329=FACE_OUTER_BOUND('',#3081,.T.);
#2330=FACE_OUTER_BOUND('',#3082,.T.);
#2331=FACE_OUTER_BOUND('',#3083,.T.);
#2332=FACE_OUTER_BOUND('',#3084,.T.);
#2333=FACE_OUTER_BOUND('',#3085,.T.);
#2334=FACE_OUTER_BOUND('',#3086,.T.);
#2335=FACE_OUTER_BOUND('',#3087,.T.);
#2336=FACE_OUTER_BOUND('',#3088,.T.);
#2337=FACE_OUTER_BOUND('',#3089,.T.);
#2338=FACE_OUTER_BOUND('',#3090,.T.);
#2339=FACE_OUTER_BOUND('',#3091,.T.);
#2340=FACE_OUTER_BOUND('',#3092,.T.);
#2341=FACE_OUTER_BOUND('',#3093,.T.);
#2342=FACE_OUTER_BOUND('',#3094,.T.);
#2343=FACE_OUTER_BOUND('',#3095,.T.);
#2344=FACE_OUTER_BOUND('',#3096,.T.);
#2345=FACE_OUTER_BOUND('',#3097,.T.);
#2346=FACE_OUTER_BOUND('',#3098,.T.);
#2347=FACE_OUTER_BOUND('',#3099,.T.);
#2348=FACE_OUTER_BOUND('',#3100,.T.);
#2349=FACE_OUTER_BOUND('',#3101,.T.);
#2350=FACE_OUTER_BOUND('',#3102,.T.);
#2351=FACE_OUTER_BOUND('',#3103,.T.);
#2352=FACE_OUTER_BOUND('',#3104,.T.);
#2353=FACE_OUTER_BOUND('',#3105,.T.);
#2354=FACE_OUTER_BOUND('',#3106,.T.);
#2355=FACE_OUTER_BOUND('',#3107,.T.);
#2356=FACE_OUTER_BOUND('',#3108,.T.);
#2357=FACE_OUTER_BOUND('',#3109,.T.);
#2358=FACE_OUTER_BOUND('',#3110,.T.);
#2359=FACE_OUTER_BOUND('',#3111,.T.);
#2360=FACE_OUTER_BOUND('',#3112,.T.);
#2361=FACE_OUTER_BOUND('',#3113,.T.);
#2362=FACE_OUTER_BOUND('',#3114,.T.);
#2363=FACE_OUTER_BOUND('',#3115,.T.);
#2364=FACE_OUTER_BOUND('',#3116,.T.);
#2365=FACE_OUTER_BOUND('',#3117,.T.);
#2366=FACE_OUTER_BOUND('',#3118,.T.);
#2367=FACE_OUTER_BOUND('',#3119,.T.);
#2368=FACE_OUTER_BOUND('',#3120,.T.);
#2369=FACE_OUTER_BOUND('',#3121,.T.);
#2370=FACE_OUTER_BOUND('',#3122,.T.);
#2371=FACE_OUTER_BOUND('',#3123,.T.);
#2372=FACE_OUTER_BOUND('',#3124,.T.);
#2373=FACE_OUTER_BOUND('',#3125,.T.);
#2374=FACE_OUTER_BOUND('',#3126,.T.);
#2375=FACE_OUTER_BOUND('',#3127,.T.);
#2376=FACE_OUTER_BOUND('',#3128,.T.);
#2377=FACE_OUTER_BOUND('',#3129,.T.);
#2378=FACE_OUTER_BOUND('',#3130,.T.);
#2379=FACE_OUTER_BOUND('',#3131,.T.);
#2380=FACE_OUTER_BOUND('',#3132,.T.);
#2381=FACE_OUTER_BOUND('',#3133,.T.);
#2382=FACE_OUTER_BOUND('',#3134,.T.);
#2383=FACE_OUTER_BOUND('',#3135,.T.);
#2384=FACE_OUTER_BOUND('',#3136,.T.);
#2385=FACE_OUTER_BOUND('',#3137,.T.);
#2386=FACE_OUTER_BOUND('',#3138,.T.);
#2387=FACE_OUTER_BOUND('',#3139,.T.);
#2388=FACE_OUTER_BOUND('',#3140,.T.);
#2389=FACE_OUTER_BOUND('',#3141,.T.);
#2390=FACE_OUTER_BOUND('',#3142,.T.);
#2391=FACE_OUTER_BOUND('',#3143,.T.);
#2392=FACE_OUTER_BOUND('',#3144,.T.);
#2393=FACE_OUTER_BOUND('',#3145,.T.);
#2394=FACE_OUTER_BOUND('',#3146,.T.);
#2395=FACE_OUTER_BOUND('',#3147,.T.);
#2396=FACE_OUTER_BOUND('',#3148,.T.);
#2397=FACE_OUTER_BOUND('',#3149,.T.);
#2398=FACE_OUTER_BOUND('',#3150,.T.);
#2399=FACE_OUTER_BOUND('',#3151,.T.);
#2400=FACE_OUTER_BOUND('',#3152,.T.);
#2401=FACE_OUTER_BOUND('',#3153,.T.);
#2402=FACE_OUTER_BOUND('',#3154,.T.);
#2403=FACE_OUTER_BOUND('',#3155,.T.);
#2404=FACE_OUTER_BOUND('',#3156,.T.);
#2405=FACE_OUTER_BOUND('',#3157,.T.);
#2406=FACE_OUTER_BOUND('',#3158,.T.);
#2407=FACE_OUTER_BOUND('',#3159,.T.);
#2408=FACE_OUTER_BOUND('',#3160,.T.);
#2409=FACE_OUTER_BOUND('',#3161,.T.);
#2410=FACE_OUTER_BOUND('',#3162,.T.);
#2411=FACE_OUTER_BOUND('',#3163,.T.);
#2412=FACE_OUTER_BOUND('',#3164,.T.);
#2413=FACE_OUTER_BOUND('',#3165,.T.);
#2414=FACE_OUTER_BOUND('',#3166,.T.);
#2415=FACE_OUTER_BOUND('',#3167,.T.);
#2416=FACE_OUTER_BOUND('',#3168,.T.);
#2417=FACE_OUTER_BOUND('',#3169,.T.);
#2418=FACE_OUTER_BOUND('',#3170,.T.);
#2419=FACE_OUTER_BOUND('',#3171,.T.);
#2420=FACE_OUTER_BOUND('',#3172,.T.);
#2421=FACE_OUTER_BOUND('',#3173,.T.);
#2422=FACE_OUTER_BOUND('',#3174,.T.);
#2423=FACE_OUTER_BOUND('',#3175,.T.);
#2424=FACE_OUTER_BOUND('',#3176,.T.);
#2425=FACE_OUTER_BOUND('',#3177,.T.);
#2426=FACE_OUTER_BOUND('',#3178,.T.);
#2427=FACE_OUTER_BOUND('',#3179,.T.);
#2428=FACE_OUTER_BOUND('',#3180,.T.);
#2429=FACE_OUTER_BOUND('',#3181,.T.);
#2430=FACE_OUTER_BOUND('',#3182,.T.);
#2431=FACE_OUTER_BOUND('',#3183,.T.);
#2432=FACE_OUTER_BOUND('',#3184,.T.);
#2433=FACE_OUTER_BOUND('',#3185,.T.);
#2434=FACE_OUTER_BOUND('',#3186,.T.);
#2435=FACE_OUTER_BOUND('',#3187,.T.);
#2436=FACE_OUTER_BOUND('',#3188,.T.);
#2437=FACE_OUTER_BOUND('',#3189,.T.);
#2438=FACE_OUTER_BOUND('',#3190,.T.);
#2439=FACE_OUTER_BOUND('',#3191,.T.);
#2440=FACE_OUTER_BOUND('',#3192,.T.);
#2441=FACE_OUTER_BOUND('',#3193,.T.);
#2442=FACE_OUTER_BOUND('',#3194,.T.);
#2443=FACE_OUTER_BOUND('',#3195,.T.);
#2444=FACE_OUTER_BOUND('',#3196,.T.);
#2445=FACE_OUTER_BOUND('',#3197,.T.);
#2446=FACE_OUTER_BOUND('',#3198,.T.);
#2447=FACE_OUTER_BOUND('',#3199,.T.);
#2448=FACE_OUTER_BOUND('',#3200,.T.);
#2449=FACE_OUTER_BOUND('',#3201,.T.);
#2450=FACE_OUTER_BOUND('',#3202,.T.);
#2451=FACE_OUTER_BOUND('',#3203,.T.);
#2452=FACE_OUTER_BOUND('',#3204,.T.);
#2453=FACE_OUTER_BOUND('',#3205,.T.);
#2454=FACE_OUTER_BOUND('',#3206,.T.);
#2455=FACE_OUTER_BOUND('',#3207,.T.);
#2456=FACE_OUTER_BOUND('',#3208,.T.);
#2457=FACE_OUTER_BOUND('',#3209,.T.);
#2458=FACE_OUTER_BOUND('',#3211,.T.);
#2459=FACE_OUTER_BOUND('',#3212,.T.);
#2460=FACE_OUTER_BOUND('',#3213,.T.);
#2461=FACE_OUTER_BOUND('',#3214,.T.);
#2462=FACE_OUTER_BOUND('',#3216,.T.);
#2463=FACE_OUTER_BOUND('',#3217,.T.);
#2464=FACE_OUTER_BOUND('',#3218,.T.);
#2465=FACE_OUTER_BOUND('',#3219,.T.);
#3002=EDGE_LOOP('',(#10165,#10166,#10167,#10168));
#3003=EDGE_LOOP('',(#10169,#10170,#10171,#10172));
#3004=EDGE_LOOP('',(#10173,#10174,#10175,#10176));
#3005=EDGE_LOOP('',(#10177,#10178,#10179,#10180));
#3006=EDGE_LOOP('',(#10181,#10182,#10183,#10184));
#3007=EDGE_LOOP('',(#10185,#10186,#10187,#10188));
#3008=EDGE_LOOP('',(#10189,#10190,#10191,#10192));
#3009=EDGE_LOOP('',(#10193,#10194,#10195,#10196));
#3010=EDGE_LOOP('',(#10197,#10198,#10199,#10200));
#3011=EDGE_LOOP('',(#10201,#10202,#10203,#10204));
#3012=EDGE_LOOP('',(#10205,#10206,#10207,#10208));
#3013=EDGE_LOOP('',(#10209,#10210,#10211,#10212));
#3014=EDGE_LOOP('',(#10213,#10214,#10215,#10216));
#3015=EDGE_LOOP('',(#10217,#10218,#10219,#10220));
#3016=EDGE_LOOP('',(#10221,#10222,#10223,#10224));
#3017=EDGE_LOOP('',(#10225,#10226,#10227,#10228));
#3018=EDGE_LOOP('',(#10229,#10230,#10231,#10232));
#3019=EDGE_LOOP('',(#10233,#10234,#10235,#10236));
#3020=EDGE_LOOP('',(#10237,#10238,#10239,#10240));
#3021=EDGE_LOOP('',(#10241,#10242,#10243,#10244));
#3022=EDGE_LOOP('',(#10245,#10246,#10247,#10248));
#3023=EDGE_LOOP('',(#10249,#10250,#10251,#10252));
#3024=EDGE_LOOP('',(#10253,#10254,#10255,#10256));
#3025=EDGE_LOOP('',(#10257,#10258,#10259,#10260));
#3026=EDGE_LOOP('',(#10261,#10262,#10263));
#3027=EDGE_LOOP('',(#10264,#10265,#10266,#10267,#10268));
#3028=EDGE_LOOP('',(#10269,#10270,#10271,#10272));
#3029=EDGE_LOOP('',(#10273,#10274,#10275,#10276));
#3030=EDGE_LOOP('',(#10277,#10278,#10279,#10280));
#3031=EDGE_LOOP('',(#10281,#10282,#10283,#10284));
#3032=EDGE_LOOP('',(#10285,#10286,#10287,#10288));
#3033=EDGE_LOOP('',(#10289,#10290,#10291,#10292));
#3034=EDGE_LOOP('',(#10293,#10294,#10295,#10296));
#3035=EDGE_LOOP('',(#10297,#10298,#10299,#10300));
#3036=EDGE_LOOP('',(#10301,#10302,#10303,#10304));
#3037=EDGE_LOOP('',(#10305,#10306,#10307,#10308));
#3038=EDGE_LOOP('',(#10309,#10310,#10311,#10312));
#3039=EDGE_LOOP('',(#10313,#10314,#10315,#10316));
#3040=EDGE_LOOP('',(#10317,#10318,#10319,#10320));
#3041=EDGE_LOOP('',(#10321,#10322,#10323,#10324));
#3042=EDGE_LOOP('',(#10325,#10326,#10327,#10328));
#3043=EDGE_LOOP('',(#10329,#10330,#10331,#10332));
#3044=EDGE_LOOP('',(#10333,#10334,#10335,#10336));
#3045=EDGE_LOOP('',(#10337,#10338,#10339,#10340));
#3046=EDGE_LOOP('',(#10341,#10342,#10343,#10344));
#3047=EDGE_LOOP('',(#10345,#10346,#10347,#10348));
#3048=EDGE_LOOP('',(#10349,#10350,#10351,#10352));
#3049=EDGE_LOOP('',(#10353,#10354,#10355,#10356));
#3050=EDGE_LOOP('',(#10357,#10358,#10359,#10360,#10361,#10362,#10363,#10364,
#10365,#10366,#10367,#10368,#10369,#10370,#10371,#10372,#10373,#10374,#10375,
#10376,#10377,#10378,#10379,#10380,#10381,#10382,#10383,#10384,#10385,#10386,
#10387,#10388,#10389,#10390,#10391,#10392,#10393,#10394,#10395,#10396,#10397,
#10398,#10399,#10400,#10401,#10402,#10403,#10404,#10405,#10406,#10407));
#3051=EDGE_LOOP('',(#10408,#10409,#10410,#10411,#10412));
#3052=EDGE_LOOP('',(#10413,#10414,#10415,#10416));
#3053=EDGE_LOOP('',(#10417,#10418,#10419,#10420,#10421,#10422,#10423,#10424,
#10425,#10426,#10427,#10428,#10429,#10430,#10431,#10432,#10433,#10434,#10435,
#10436,#10437,#10438,#10439,#10440,#10441,#10442,#10443,#10444,#10445,#10446,
#10447,#10448,#10449,#10450,#10451,#10452,#10453,#10454,#10455,#10456,#10457,
#10458,#10459,#10460,#10461,#10462,#10463,#10464,#10465,#10466,#10467,#10468));
#3054=EDGE_LOOP('',(#10469,#10470,#10471));
#3055=EDGE_LOOP('',(#10472,#10473,#10474,#10475));
#3056=EDGE_LOOP('',(#10476,#10477,#10478,#10479));
#3057=EDGE_LOOP('',(#10480,#10481,#10482,#10483));
#3058=EDGE_LOOP('',(#10484,#10485,#10486,#10487));
#3059=EDGE_LOOP('',(#10488,#10489,#10490,#10491));
#3060=EDGE_LOOP('',(#10492,#10493,#10494,#10495));
#3061=EDGE_LOOP('',(#10496,#10497,#10498,#10499,#10500,#10501));
#3062=EDGE_LOOP('',(#10502));
#3063=EDGE_LOOP('',(#10503,#10504,#10505,#10506));
#3064=EDGE_LOOP('',(#10507,#10508,#10509));
#3065=EDGE_LOOP('',(#10510,#10511,#10512,#10513));
#3066=EDGE_LOOP('',(#10514,#10515,#10516));
#3067=EDGE_LOOP('',(#10517,#10518,#10519,#10520));
#3068=EDGE_LOOP('',(#10521,#10522,#10523));
#3069=EDGE_LOOP('',(#10524,#10525,#10526,#10527));
#3070=EDGE_LOOP('',(#10528,#10529,#10530));
#3071=EDGE_LOOP('',(#10531,#10532,#10533,#10534));
#3072=EDGE_LOOP('',(#10535,#10536,#10537));
#3073=EDGE_LOOP('',(#10538,#10539,#10540,#10541));
#3074=EDGE_LOOP('',(#10542,#10543,#10544));
#3075=EDGE_LOOP('',(#10545,#10546,#10547,#10548));
#3076=EDGE_LOOP('',(#10549,#10550,#10551));
#3077=EDGE_LOOP('',(#10552,#10553,#10554,#10555));
#3078=EDGE_LOOP('',(#10556,#10557,#10558));
#3079=EDGE_LOOP('',(#10559,#10560,#10561,#10562));
#3080=EDGE_LOOP('',(#10563,#10564,#10565));
#3081=EDGE_LOOP('',(#10566,#10567,#10568,#10569));
#3082=EDGE_LOOP('',(#10570,#10571,#10572));
#3083=EDGE_LOOP('',(#10573,#10574,#10575,#10576));
#3084=EDGE_LOOP('',(#10577,#10578,#10579));
#3085=EDGE_LOOP('',(#10580,#10581,#10582,#10583));
#3086=EDGE_LOOP('',(#10584,#10585,#10586));
#3087=EDGE_LOOP('',(#10587,#10588,#10589,#10590));
#3088=EDGE_LOOP('',(#10591,#10592,#10593));
#3089=EDGE_LOOP('',(#10594,#10595,#10596,#10597));
#3090=EDGE_LOOP('',(#10598,#10599,#10600));
#3091=EDGE_LOOP('',(#10601,#10602,#10603,#10604));
#3092=EDGE_LOOP('',(#10605,#10606,#10607));
#3093=EDGE_LOOP('',(#10608,#10609,#10610,#10611));
#3094=EDGE_LOOP('',(#10612,#10613,#10614));
#3095=EDGE_LOOP('',(#10615,#10616,#10617,#10618));
#3096=EDGE_LOOP('',(#10619,#10620,#10621,#10622));
#3097=EDGE_LOOP('',(#10623,#10624,#10625,#10626));
#3098=EDGE_LOOP('',(#10627,#10628,#10629,#10630));
#3099=EDGE_LOOP('',(#10631,#10632,#10633,#10634));
#3100=EDGE_LOOP('',(#10635,#10636,#10637));
#3101=EDGE_LOOP('',(#10638,#10639,#10640,#10641));
#3102=EDGE_LOOP('',(#10642,#10643,#10644));
#3103=EDGE_LOOP('',(#10645,#10646,#10647,#10648));
#3104=EDGE_LOOP('',(#10649,#10650,#10651));
#3105=EDGE_LOOP('',(#10652,#10653,#10654,#10655));
#3106=EDGE_LOOP('',(#10656,#10657,#10658));
#3107=EDGE_LOOP('',(#10659,#10660,#10661,#10662));
#3108=EDGE_LOOP('',(#10663,#10664,#10665));
#3109=EDGE_LOOP('',(#10666,#10667,#10668,#10669));
#3110=EDGE_LOOP('',(#10670,#10671,#10672));
#3111=EDGE_LOOP('',(#10673,#10674,#10675,#10676));
#3112=EDGE_LOOP('',(#10677,#10678,#10679));
#3113=EDGE_LOOP('',(#10680,#10681,#10682,#10683));
#3114=EDGE_LOOP('',(#10684,#10685,#10686));
#3115=EDGE_LOOP('',(#10687,#10688,#10689,#10690));
#3116=EDGE_LOOP('',(#10691,#10692,#10693));
#3117=EDGE_LOOP('',(#10694,#10695,#10696,#10697));
#3118=EDGE_LOOP('',(#10698,#10699,#10700));
#3119=EDGE_LOOP('',(#10701,#10702,#10703,#10704));
#3120=EDGE_LOOP('',(#10705,#10706,#10707));
#3121=EDGE_LOOP('',(#10708,#10709,#10710,#10711));
#3122=EDGE_LOOP('',(#10712,#10713,#10714));
#3123=EDGE_LOOP('',(#10715,#10716,#10717,#10718));
#3124=EDGE_LOOP('',(#10719,#10720,#10721));
#3125=EDGE_LOOP('',(#10722,#10723,#10724,#10725));
#3126=EDGE_LOOP('',(#10726,#10727,#10728));
#3127=EDGE_LOOP('',(#10729,#10730,#10731,#10732));
#3128=EDGE_LOOP('',(#10733,#10734,#10735));
#3129=EDGE_LOOP('',(#10736,#10737,#10738,#10739));
#3130=EDGE_LOOP('',(#10740,#10741,#10742));
#3131=EDGE_LOOP('',(#10743,#10744,#10745,#10746));
#3132=EDGE_LOOP('',(#10747,#10748,#10749));
#3133=EDGE_LOOP('',(#10750,#10751,#10752,#10753));
#3134=EDGE_LOOP('',(#10754,#10755,#10756));
#3135=EDGE_LOOP('',(#10757,#10758,#10759,#10760));
#3136=EDGE_LOOP('',(#10761,#10762,#10763));
#3137=EDGE_LOOP('',(#10764,#10765,#10766,#10767));
#3138=EDGE_LOOP('',(#10768,#10769,#10770));
#3139=EDGE_LOOP('',(#10771,#10772,#10773,#10774));
#3140=EDGE_LOOP('',(#10775,#10776,#10777));
#3141=EDGE_LOOP('',(#10778,#10779,#10780,#10781));
#3142=EDGE_LOOP('',(#10782,#10783,#10784));
#3143=EDGE_LOOP('',(#10785,#10786,#10787,#10788));
#3144=EDGE_LOOP('',(#10789,#10790,#10791));
#3145=EDGE_LOOP('',(#10792,#10793,#10794,#10795));
#3146=EDGE_LOOP('',(#10796,#10797,#10798));
#3147=EDGE_LOOP('',(#10799,#10800,#10801,#10802));
#3148=EDGE_LOOP('',(#10803,#10804,#10805));
#3149=EDGE_LOOP('',(#10806,#10807,#10808,#10809));
#3150=EDGE_LOOP('',(#10810,#10811,#10812));
#3151=EDGE_LOOP('',(#10813,#10814,#10815,#10816));
#3152=EDGE_LOOP('',(#10817,#10818,#10819));
#3153=EDGE_LOOP('',(#10820,#10821,#10822,#10823));
#3154=EDGE_LOOP('',(#10824,#10825,#10826));
#3155=EDGE_LOOP('',(#10827,#10828,#10829,#10830));
#3156=EDGE_LOOP('',(#10831,#10832,#10833));
#3157=EDGE_LOOP('',(#10834,#10835,#10836,#10837));
#3158=EDGE_LOOP('',(#10838,#10839,#10840));
#3159=EDGE_LOOP('',(#10841,#10842,#10843,#10844));
#3160=EDGE_LOOP('',(#10845,#10846,#10847));
#3161=EDGE_LOOP('',(#10848,#10849,#10850,#10851));
#3162=EDGE_LOOP('',(#10852,#10853,#10854));
#3163=EDGE_LOOP('',(#10855,#10856,#10857,#10858));
#3164=EDGE_LOOP('',(#10859,#10860,#10861));
#3165=EDGE_LOOP('',(#10862,#10863,#10864,#10865));
#3166=EDGE_LOOP('',(#10866,#10867,#10868));
#3167=EDGE_LOOP('',(#10869,#10870,#10871));
#3168=EDGE_LOOP('',(#10872,#10873,#10874,#10875));
#3169=EDGE_LOOP('',(#10876,#10877,#10878,#10879));
#3170=EDGE_LOOP('',(#10880,#10881,#10882));
#3171=EDGE_LOOP('',(#10883,#10884,#10885,#10886));
#3172=EDGE_LOOP('',(#10887,#10888,#10889));
#3173=EDGE_LOOP('',(#10890,#10891,#10892,#10893));
#3174=EDGE_LOOP('',(#10894,#10895,#10896));
#3175=EDGE_LOOP('',(#10897,#10898,#10899,#10900));
#3176=EDGE_LOOP('',(#10901,#10902,#10903));
#3177=EDGE_LOOP('',(#10904,#10905,#10906,#10907));
#3178=EDGE_LOOP('',(#10908,#10909,#10910));
#3179=EDGE_LOOP('',(#10911,#10912,#10913,#10914));
#3180=EDGE_LOOP('',(#10915,#10916,#10917));
#3181=EDGE_LOOP('',(#10918,#10919,#10920,#10921));
#3182=EDGE_LOOP('',(#10922,#10923,#10924));
#3183=EDGE_LOOP('',(#10925,#10926,#10927,#10928));
#3184=EDGE_LOOP('',(#10929,#10930,#10931));
#3185=EDGE_LOOP('',(#10932,#10933,#10934,#10935));
#3186=EDGE_LOOP('',(#10936,#10937,#10938));
#3187=EDGE_LOOP('',(#10939,#10940,#10941,#10942));
#3188=EDGE_LOOP('',(#10943,#10944,#10945));
#3189=EDGE_LOOP('',(#10946,#10947,#10948,#10949));
#3190=EDGE_LOOP('',(#10950,#10951,#10952));
#3191=EDGE_LOOP('',(#10953,#10954,#10955,#10956));
#3192=EDGE_LOOP('',(#10957,#10958,#10959));
#3193=EDGE_LOOP('',(#10960,#10961,#10962,#10963));
#3194=EDGE_LOOP('',(#10964,#10965,#10966));
#3195=EDGE_LOOP('',(#10967,#10968,#10969,#10970));
#3196=EDGE_LOOP('',(#10971,#10972,#10973));
#3197=EDGE_LOOP('',(#10974,#10975,#10976,#10977));
#3198=EDGE_LOOP('',(#10978,#10979,#10980));
#3199=EDGE_LOOP('',(#10981,#10982,#10983,#10984));
#3200=EDGE_LOOP('',(#10985,#10986,#10987));
#3201=EDGE_LOOP('',(#10988,#10989,#10990,#10991));
#3202=EDGE_LOOP('',(#10992,#10993,#10994));
#3203=EDGE_LOOP('',(#10995,#10996,#10997,#10998));
#3204=EDGE_LOOP('',(#10999,#11000,#11001));
#3205=EDGE_LOOP('',(#11002,#11003,#11004,#11005));
#3206=EDGE_LOOP('',(#11006,#11007,#11008));
#3207=EDGE_LOOP('',(#11009,#11010,#11011,#11012));
#3208=EDGE_LOOP('',(#11013,#11014,#11015,#11016));
#3209=EDGE_LOOP('',(#11017));
#3210=EDGE_LOOP('',(#11018));
#3211=EDGE_LOOP('',(#11019));
#3212=EDGE_LOOP('',(#11020,#11021,#11022,#11023,#11024,#11025));
#3213=EDGE_LOOP('',(#11026,#11027,#11028,#11029));
#3214=EDGE_LOOP('',(#11030));
#3215=EDGE_LOOP('',(#11031,#11032,#11033,#11034,#11035));
#3216=EDGE_LOOP('',(#11036,#11037,#11038,#11039));
#3217=EDGE_LOOP('',(#11040,#11041,#11042,#11043,#11044,#11045,#11046,#11047,
#11048,#11049,#11050,#11051,#11052,#11053,#11054,#11055,#11056,#11057,#11058,
#11059,#11060,#11061,#11062,#11063,#11064,#11065,#11066,#11067,#11068,#11069,
#11070,#11071,#11072,#11073,#11074,#11075,#11076,#11077,#11078,#11079,#11080,
#11081,#11082,#11083,#11084,#11085,#11086,#11087,#11088,#11089,#11090,#11091,
#11092,#11093,#11094,#11095,#11096,#11097,#11098,#11099,#11100,#11101,#11102,
#11103,#11104,#11105,#11106,#11107,#11108,#11109,#11110,#11111,#11112,#11113,
#11114,#11115,#11116,#11117,#11118,#11119,#11120,#11121,#11122,#11123,#11124,
#11125,#11126,#11127,#11128,#11129,#11130,#11131,#11132,#11133,#11134,#11135,
#11136,#11137,#11138,#11139,#11140,#11141,#11142,#11143,#11144,#11145,#11146,
#11147,#11148,#11149,#11150,#11151,#11152,#11153,#11154,#11155,#11156,#11157,
#11158,#11159,#11160,#11161,#11162,#11163,#11164,#11165,#11166,#11167,#11168,
#11169,#11170,#11171,#11172,#11173,#11174,#11175,#11176,#11177,#11178,#11179,
#11180,#11181,#11182,#11183,#11184,#11185,#11186,#11187));
#3218=EDGE_LOOP('',(#11188,#11189,#11190,#11191,#11192,#11193,#11194,#11195,
#11196,#11197,#11198,#11199,#11200,#11201,#11202,#11203,#11204,#11205,#11206,
#11207,#11208,#11209,#11210,#11211,#11212,#11213,#11214,#11215,#11216,#11217,
#11218,#11219,#11220,#11221,#11222,#11223,#11224,#11225,#11226,#11227,#11228,
#11229,#11230,#11231,#11232,#11233,#11234,#11235,#11236,#11237,#11238,#11239,
#11240,#11241,#11242,#11243,#11244,#11245,#11246,#11247,#11248,#11249,#11250,
#11251,#11252,#11253,#11254,#11255,#11256,#11257,#11258,#11259,#11260,#11261,
#11262,#11263));
#3219=EDGE_LOOP('',(#11264));
#3220=EDGE_LOOP('',(#11265,#11266,#11267,#11268,#11269,#11270));
#3622=LINE('',#26912,#4327);
#3623=LINE('',#26936,#4328);
#3624=LINE('',#26984,#4329);
#3625=LINE('',#27032,#4330);
#3626=LINE('',#27083,#4331);
#3627=LINE('',#27134,#4332);
#3628=LINE('',#27182,#4333);
#3629=LINE('',#27230,#4334);
#3630=LINE('',#27284,#4335);
#3631=LINE('',#27332,#4336);
#3632=LINE('',#27380,#4337);
#3633=LINE('',#27434,#4338);
#3634=LINE('',#27482,#4339);
#3635=LINE('',#27530,#4340);
#3636=LINE('',#27578,#4341);
#3637=LINE('',#27632,#4342);
#3638=LINE('',#27680,#4343);
#3639=LINE('',#27728,#4344);
#3640=LINE('',#27782,#4345);
#3641=LINE('',#27830,#4346);
#3642=LINE('',#27878,#4347);
#3643=LINE('',#27929,#4348);
#3644=LINE('',#27977,#4349);
#3645=LINE('',#28025,#4350);
#3646=LINE('',#28073,#4351);
#3647=LINE('',#28083,#4352);
#3648=LINE('',#28108,#4353);
#3649=LINE('',#28132,#4354);
#3650=LINE('',#28156,#4355);
#3651=LINE('',#28181,#4356);
#3652=LINE('',#28206,#4357);
#3653=LINE('',#28230,#4358);
#3654=LINE('',#28255,#4359);
#3655=LINE('',#28280,#4360);
#3656=LINE('',#28304,#4361);
#3657=LINE('',#28329,#4362);
#3658=LINE('',#28354,#4363);
#3659=LINE('',#28378,#4364);
#3660=LINE('',#28402,#4365);
#3661=LINE('',#28427,#4366);
#3662=LINE('',#28452,#4367);
#3663=LINE('',#28476,#4368);
#3664=LINE('',#28501,#4369);
#3665=LINE('',#28526,#4370);
#3666=LINE('',#28550,#4371);
#3667=LINE('',#28575,#4372);
#3668=LINE('',#28599,#4373);
#3669=LINE('',#28624,#4374);
#3670=LINE('',#30156,#4375);
#3671=LINE('',#30161,#4376);
#3672=LINE('',#30163,#4377);
#3673=LINE('',#30165,#4378);
#3674=LINE('',#30166,#4379);
#3675=LINE('',#30169,#4380);
#3676=LINE('',#30171,#4381);
#3677=LINE('',#30172,#4382);
#3678=LINE('',#30175,#4383);
#3679=LINE('',#30177,#4384);
#3680=LINE('',#30178,#4385);
#3681=LINE('',#30181,#4386);
#3682=LINE('',#30183,#4387);
#3683=LINE('',#30184,#4388);
#3684=LINE('',#30187,#4389);
#3685=LINE('',#30189,#4390);
#3686=LINE('',#30190,#4391);
#3687=LINE('',#30192,#4392);
#3688=LINE('',#30193,#4393);
#3689=LINE('',#30198,#4394);
#3690=LINE('',#30200,#4395);
#3691=LINE('',#30202,#4396);
#3692=LINE('',#30203,#4397);
#3693=LINE('',#30207,#4398);
#3694=LINE('',#30210,#4399);
#3695=LINE('',#30211,#4400);
#3696=LINE('',#30217,#4401);
#3697=LINE('',#30219,#4402);
#3698=LINE('',#30221,#4403);
#3699=LINE('',#30222,#4404);
#3700=LINE('',#30226,#4405);
#3701=LINE('',#30229,#4406);
#3702=LINE('',#30230,#4407);
#3703=LINE('',#30236,#4408);
#3704=LINE('',#30238,#4409);
#3705=LINE('',#30240,#4410);
#3706=LINE('',#30241,#4411);
#3707=LINE('',#30245,#4412);
#3708=LINE('',#30248,#4413);
#3709=LINE('',#30249,#4414);
#3710=LINE('',#30255,#4415);
#3711=LINE('',#30257,#4416);
#3712=LINE('',#30259,#4417);
#3713=LINE('',#30260,#4418);
#3714=LINE('',#30264,#4419);
#3715=LINE('',#30267,#4420);
#3716=LINE('',#30268,#4421);
#3717=LINE('',#30274,#4422);
#3718=LINE('',#30276,#4423);
#3719=LINE('',#30278,#4424);
#3720=LINE('',#30279,#4425);
#3721=LINE('',#30283,#4426);
#3722=LINE('',#30286,#4427);
#3723=LINE('',#30287,#4428);
#3724=LINE('',#30293,#4429);
#3725=LINE('',#30295,#4430);
#3726=LINE('',#30297,#4431);
#3727=LINE('',#30298,#4432);
#3728=LINE('',#30302,#4433);
#3729=LINE('',#30305,#4434);
#3730=LINE('',#30306,#4435);
#3731=LINE('',#30312,#4436);
#3732=LINE('',#30314,#4437);
#3733=LINE('',#30316,#4438);
#3734=LINE('',#30317,#4439);
#3735=LINE('',#30321,#4440);
#3736=LINE('',#30324,#4441);
#3737=LINE('',#30325,#4442);
#3738=LINE('',#30331,#4443);
#3739=LINE('',#30333,#4444);
#3740=LINE('',#30335,#4445);
#3741=LINE('',#30336,#4446);
#3742=LINE('',#30340,#4447);
#3743=LINE('',#30343,#4448);
#3744=LINE('',#30344,#4449);
#3745=LINE('',#30350,#4450);
#3746=LINE('',#30352,#4451);
#3747=LINE('',#30354,#4452);
#3748=LINE('',#30355,#4453);
#3749=LINE('',#30360,#4454);
#3750=LINE('',#30364,#4455);
#3751=LINE('',#30365,#4456);
#3752=LINE('',#30373,#4457);
#3753=LINE('',#30375,#4458);
#3754=LINE('',#30377,#4459);
#3755=LINE('',#30378,#4460);
#3756=LINE('',#30382,#4461);
#3757=LINE('',#30385,#4462);
#3758=LINE('',#30386,#4463);
#3759=LINE('',#30392,#4464);
#3760=LINE('',#30394,#4465);
#3761=LINE('',#30396,#4466);
#3762=LINE('',#30397,#4467);
#3763=LINE('',#30401,#4468);
#3764=LINE('',#30404,#4469);
#3765=LINE('',#30405,#4470);
#3766=LINE('',#30411,#4471);
#3767=LINE('',#30413,#4472);
#3768=LINE('',#30415,#4473);
#3769=LINE('',#30416,#4474);
#3770=LINE('',#30420,#4475);
#3771=LINE('',#30423,#4476);
#3772=LINE('',#30424,#4477);
#3773=LINE('',#30430,#4478);
#3774=LINE('',#30432,#4479);
#3775=LINE('',#30434,#4480);
#3776=LINE('',#30435,#4481);
#3777=LINE('',#30439,#4482);
#3778=LINE('',#30442,#4483);
#3779=LINE('',#30443,#4484);
#3780=LINE('',#30449,#4485);
#3781=LINE('',#30451,#4486);
#3782=LINE('',#30453,#4487);
#3783=LINE('',#30454,#4488);
#3784=LINE('',#30458,#4489);
#3785=LINE('',#30461,#4490);
#3786=LINE('',#30462,#4491);
#3787=LINE('',#30468,#4492);
#3788=LINE('',#30470,#4493);
#3789=LINE('',#30472,#4494);
#3790=LINE('',#30473,#4495);
#3791=LINE('',#30477,#4496);
#3792=LINE('',#30480,#4497);
#3793=LINE('',#30481,#4498);
#3794=LINE('',#30487,#4499);
#3795=LINE('',#30489,#4500);
#3796=LINE('',#30491,#4501);
#3797=LINE('',#30492,#4502);
#3798=LINE('',#30496,#4503);
#3799=LINE('',#30499,#4504);
#3800=LINE('',#30500,#4505);
#3801=LINE('',#30506,#4506);
#3802=LINE('',#30508,#4507);
#3803=LINE('',#30510,#4508);
#3804=LINE('',#30511,#4509);
#3805=LINE('',#30515,#4510);
#3806=LINE('',#30518,#4511);
#3807=LINE('',#30519,#4512);
#3808=LINE('',#30525,#4513);
#3809=LINE('',#30527,#4514);
#3810=LINE('',#30529,#4515);
#3811=LINE('',#30530,#4516);
#3812=LINE('',#30534,#4517);
#3813=LINE('',#30537,#4518);
#3814=LINE('',#30538,#4519);
#3815=LINE('',#30544,#4520);
#3816=LINE('',#30546,#4521);
#3817=LINE('',#30548,#4522);
#3818=LINE('',#30549,#4523);
#3819=LINE('',#30553,#4524);
#3820=LINE('',#30556,#4525);
#3821=LINE('',#30557,#4526);
#3822=LINE('',#30563,#4527);
#3823=LINE('',#30565,#4528);
#3824=LINE('',#30567,#4529);
#3825=LINE('',#30568,#4530);
#3826=LINE('',#30572,#4531);
#3827=LINE('',#30575,#4532);
#3828=LINE('',#30576,#4533);
#3829=LINE('',#30582,#4534);
#3830=LINE('',#30584,#4535);
#3831=LINE('',#30586,#4536);
#3832=LINE('',#30587,#4537);
#3833=LINE('',#30591,#4538);
#3834=LINE('',#30594,#4539);
#3835=LINE('',#30595,#4540);
#3836=LINE('',#30601,#4541);
#3837=LINE('',#30603,#4542);
#3838=LINE('',#30605,#4543);
#3839=LINE('',#30606,#4544);
#3840=LINE('',#30610,#4545);
#3841=LINE('',#30613,#4546);
#3842=LINE('',#30614,#4547);
#3843=LINE('',#30620,#4548);
#3844=LINE('',#30622,#4549);
#3845=LINE('',#30624,#4550);
#3846=LINE('',#30625,#4551);
#3847=LINE('',#30629,#4552);
#3848=LINE('',#30632,#4553);
#3849=LINE('',#30633,#4554);
#3850=LINE('',#30639,#4555);
#3851=LINE('',#30641,#4556);
#3852=LINE('',#30643,#4557);
#3853=LINE('',#30644,#4558);
#3854=LINE('',#30648,#4559);
#3855=LINE('',#30651,#4560);
#3856=LINE('',#30652,#4561);
#3857=LINE('',#30658,#4562);
#3858=LINE('',#30660,#4563);
#3859=LINE('',#30662,#4564);
#3860=LINE('',#30663,#4565);
#3861=LINE('',#30667,#4566);
#3862=LINE('',#30670,#4567);
#3863=LINE('',#30671,#4568);
#3864=LINE('',#30677,#4569);
#3865=LINE('',#30679,#4570);
#3866=LINE('',#30681,#4571);
#3867=LINE('',#30682,#4572);
#3868=LINE('',#30686,#4573);
#3869=LINE('',#30689,#4574);
#3870=LINE('',#30690,#4575);
#3871=LINE('',#30698,#4576);
#3872=LINE('',#30699,#4577);
#3873=LINE('',#30702,#4578);
#3874=LINE('',#30704,#4579);
#3875=LINE('',#30705,#4580);
#3876=LINE('',#30708,#4581);
#3877=LINE('',#30709,#4582);
#3878=LINE('',#30715,#4583);
#3879=LINE('',#30717,#4584);
#3880=LINE('',#30719,#4585);
#3881=LINE('',#30720,#4586);
#3882=LINE('',#30724,#4587);
#3883=LINE('',#30727,#4588);
#3884=LINE('',#30728,#4589);
#3885=LINE('',#30734,#4590);
#3886=LINE('',#30736,#4591);
#3887=LINE('',#30738,#4592);
#3888=LINE('',#30739,#4593);
#3889=LINE('',#30743,#4594);
#3890=LINE('',#30746,#4595);
#3891=LINE('',#30747,#4596);
#3892=LINE('',#30753,#4597);
#3893=LINE('',#30755,#4598);
#3894=LINE('',#30757,#4599);
#3895=LINE('',#30758,#4600);
#3896=LINE('',#30762,#4601);
#3897=LINE('',#30765,#4602);
#3898=LINE('',#30766,#4603);
#3899=LINE('',#30772,#4604);
#3900=LINE('',#30774,#4605);
#3901=LINE('',#30776,#4606);
#3902=LINE('',#30777,#4607);
#3903=LINE('',#30781,#4608);
#3904=LINE('',#30784,#4609);
#3905=LINE('',#30785,#4610);
#3906=LINE('',#30791,#4611);
#3907=LINE('',#30793,#4612);
#3908=LINE('',#30795,#4613);
#3909=LINE('',#30796,#4614);
#3910=LINE('',#30800,#4615);
#3911=LINE('',#30803,#4616);
#3912=LINE('',#30804,#4617);
#3913=LINE('',#30810,#4618);
#3914=LINE('',#30812,#4619);
#3915=LINE('',#30814,#4620);
#3916=LINE('',#30815,#4621);
#3917=LINE('',#30819,#4622);
#3918=LINE('',#30822,#4623);
#3919=LINE('',#30823,#4624);
#3920=LINE('',#30829,#4625);
#3921=LINE('',#30831,#4626);
#3922=LINE('',#30833,#4627);
#3923=LINE('',#30834,#4628);
#3924=LINE('',#30838,#4629);
#3925=LINE('',#30841,#4630);
#3926=LINE('',#30842,#4631);
#3927=LINE('',#30848,#4632);
#3928=LINE('',#30850,#4633);
#3929=LINE('',#30852,#4634);
#3930=LINE('',#30853,#4635);
#3931=LINE('',#30857,#4636);
#3932=LINE('',#30860,#4637);
#3933=LINE('',#30861,#4638);
#3934=LINE('',#30867,#4639);
#3935=LINE('',#30869,#4640);
#3936=LINE('',#30871,#4641);
#3937=LINE('',#30872,#4642);
#3938=LINE('',#30876,#4643);
#3939=LINE('',#30879,#4644);
#3940=LINE('',#30880,#4645);
#3941=LINE('',#30891,#4646);
#3942=LINE('',#30900,#4647);
#3943=LINE('',#30907,#4648);
#3944=LINE('',#30925,#4649);
#3945=LINE('',#30949,#4650);
#4327=VECTOR('',#15098,0.3);
#4328=VECTOR('',#15103,0.3);
#4329=VECTOR('',#15106,0.3);
#4330=VECTOR('',#15109,0.3);
#4331=VECTOR('',#15112,0.3);
#4332=VECTOR('',#15115,0.3);
#4333=VECTOR('',#15118,0.3);
#4334=VECTOR('',#15121,0.3);
#4335=VECTOR('',#15124,0.3);
#4336=VECTOR('',#15127,0.3);
#4337=VECTOR('',#15130,0.3);
#4338=VECTOR('',#15133,0.3);
#4339=VECTOR('',#15136,0.3);
#4340=VECTOR('',#15139,0.3);
#4341=VECTOR('',#15142,0.3);
#4342=VECTOR('',#15145,0.3);
#4343=VECTOR('',#15148,0.3);
#4344=VECTOR('',#15151,0.3);
#4345=VECTOR('',#15154,0.3);
#4346=VECTOR('',#15157,0.3);
#4347=VECTOR('',#15160,0.3);
#4348=VECTOR('',#15163,0.3);
#4349=VECTOR('',#15166,0.3);
#4350=VECTOR('',#15169,0.3);
#4351=VECTOR('',#15172,0.237175);
#4352=VECTOR('',#15177,0.237175);
#4353=VECTOR('',#15182,0.237175);
#4354=VECTOR('',#15185,0.237175);
#4355=VECTOR('',#15188,0.237175);
#4356=VECTOR('',#15191,0.237175);
#4357=VECTOR('',#15194,0.237175);
#4358=VECTOR('',#15197,0.237175);
#4359=VECTOR('',#15200,0.237175);
#4360=VECTOR('',#15203,0.237175);
#4361=VECTOR('',#15206,0.237175);
#4362=VECTOR('',#15209,0.237175);
#4363=VECTOR('',#15212,0.237175);
#4364=VECTOR('',#15215,0.237175);
#4365=VECTOR('',#15218,0.237175);
#4366=VECTOR('',#15221,0.237175);
#4367=VECTOR('',#15224,0.237175);
#4368=VECTOR('',#15227,0.237175);
#4369=VECTOR('',#15230,0.237175);
#4370=VECTOR('',#15233,0.237175);
#4371=VECTOR('',#15236,0.237175);
#4372=VECTOR('',#15239,0.237175);
#4373=VECTOR('',#15242,0.237175);
#4374=VECTOR('',#15245,0.237175);
#4375=VECTOR('',#15258,0.124996333279554);
#4376=VECTOR('',#15263,1.);
#4377=VECTOR('',#15264,1.);
#4378=VECTOR('',#15265,1.);
#4379=VECTOR('',#15266,1.);
#4380=VECTOR('',#15269,1.);
#4381=VECTOR('',#15270,1.);
#4382=VECTOR('',#15271,1.);
#4383=VECTOR('',#15274,1.);
#4384=VECTOR('',#15275,1.);
#4385=VECTOR('',#15276,1.);
#4386=VECTOR('',#15279,1.);
#4387=VECTOR('',#15280,1.);
#4388=VECTOR('',#15281,1.);
#4389=VECTOR('',#15284,1.);
#4390=VECTOR('',#15285,1.);
#4391=VECTOR('',#15286,1.);
#4392=VECTOR('',#15289,1.);
#4393=VECTOR('',#15290,1.);
#4394=VECTOR('',#15295,1.);
#4395=VECTOR('',#15296,1.);
#4396=VECTOR('',#15297,1.);
#4397=VECTOR('',#15298,1.);
#4398=VECTOR('',#15303,1.);
#4399=VECTOR('',#15306,1.);
#4400=VECTOR('',#15307,1.);
#4401=VECTOR('',#15314,1.);
#4402=VECTOR('',#15315,1.);
#4403=VECTOR('',#15316,1.);
#4404=VECTOR('',#15317,1.);
#4405=VECTOR('',#15322,1.);
#4406=VECTOR('',#15325,1.);
#4407=VECTOR('',#15326,1.);
#4408=VECTOR('',#15333,1.);
#4409=VECTOR('',#15334,1.);
#4410=VECTOR('',#15335,1.);
#4411=VECTOR('',#15336,1.);
#4412=VECTOR('',#15341,1.);
#4413=VECTOR('',#15344,1.);
#4414=VECTOR('',#15345,1.);
#4415=VECTOR('',#15352,1.);
#4416=VECTOR('',#15353,1.);
#4417=VECTOR('',#15354,1.);
#4418=VECTOR('',#15355,1.);
#4419=VECTOR('',#15360,1.);
#4420=VECTOR('',#15363,1.);
#4421=VECTOR('',#15364,1.);
#4422=VECTOR('',#15371,1.);
#4423=VECTOR('',#15372,1.);
#4424=VECTOR('',#15373,1.);
#4425=VECTOR('',#15374,1.);
#4426=VECTOR('',#15379,1.);
#4427=VECTOR('',#15382,1.);
#4428=VECTOR('',#15383,1.);
#4429=VECTOR('',#15390,1.);
#4430=VECTOR('',#15391,1.);
#4431=VECTOR('',#15392,1.);
#4432=VECTOR('',#15393,1.);
#4433=VECTOR('',#15398,1.);
#4434=VECTOR('',#15401,1.);
#4435=VECTOR('',#15402,1.);
#4436=VECTOR('',#15409,1.);
#4437=VECTOR('',#15410,1.);
#4438=VECTOR('',#15411,1.);
#4439=VECTOR('',#15412,1.);
#4440=VECTOR('',#15417,1.);
#4441=VECTOR('',#15420,1.);
#4442=VECTOR('',#15421,1.);
#4443=VECTOR('',#15428,1.);
#4444=VECTOR('',#15429,1.);
#4445=VECTOR('',#15430,1.);
#4446=VECTOR('',#15431,1.);
#4447=VECTOR('',#15436,1.);
#4448=VECTOR('',#15439,1.);
#4449=VECTOR('',#15440,1.);
#4450=VECTOR('',#15447,1.);
#4451=VECTOR('',#15448,1.);
#4452=VECTOR('',#15449,1.);
#4453=VECTOR('',#15450,1.);
#4454=VECTOR('',#15455,1.);
#4455=VECTOR('',#15460,1.);
#4456=VECTOR('',#15461,1.);
#4457=VECTOR('',#15470,1.);
#4458=VECTOR('',#15471,1.);
#4459=VECTOR('',#15472,1.);
#4460=VECTOR('',#15473,1.);
#4461=VECTOR('',#15478,1.);
#4462=VECTOR('',#15481,1.);
#4463=VECTOR('',#15482,1.);
#4464=VECTOR('',#15489,1.);
#4465=VECTOR('',#15490,1.);
#4466=VECTOR('',#15491,1.);
#4467=VECTOR('',#15492,1.);
#4468=VECTOR('',#15497,1.);
#4469=VECTOR('',#15500,1.);
#4470=VECTOR('',#15501,1.);
#4471=VECTOR('',#15508,1.);
#4472=VECTOR('',#15509,1.);
#4473=VECTOR('',#15510,1.);
#4474=VECTOR('',#15511,1.);
#4475=VECTOR('',#15516,1.);
#4476=VECTOR('',#15519,1.);
#4477=VECTOR('',#15520,1.);
#4478=VECTOR('',#15527,1.);
#4479=VECTOR('',#15528,1.);
#4480=VECTOR('',#15529,1.);
#4481=VECTOR('',#15530,1.);
#4482=VECTOR('',#15535,1.);
#4483=VECTOR('',#15538,1.);
#4484=VECTOR('',#15539,1.);
#4485=VECTOR('',#15546,1.);
#4486=VECTOR('',#15547,1.);
#4487=VECTOR('',#15548,1.);
#4488=VECTOR('',#15549,1.);
#4489=VECTOR('',#15554,1.);
#4490=VECTOR('',#15557,1.);
#4491=VECTOR('',#15558,1.);
#4492=VECTOR('',#15565,1.);
#4493=VECTOR('',#15566,1.);
#4494=VECTOR('',#15567,1.);
#4495=VECTOR('',#15568,1.);
#4496=VECTOR('',#15573,1.);
#4497=VECTOR('',#15576,1.);
#4498=VECTOR('',#15577,1.);
#4499=VECTOR('',#15584,1.);
#4500=VECTOR('',#15585,1.);
#4501=VECTOR('',#15586,1.);
#4502=VECTOR('',#15587,1.);
#4503=VECTOR('',#15592,1.);
#4504=VECTOR('',#15595,1.);
#4505=VECTOR('',#15596,1.);
#4506=VECTOR('',#15603,1.);
#4507=VECTOR('',#15604,1.);
#4508=VECTOR('',#15605,1.);
#4509=VECTOR('',#15606,1.);
#4510=VECTOR('',#15611,1.);
#4511=VECTOR('',#15614,1.);
#4512=VECTOR('',#15615,1.);
#4513=VECTOR('',#15622,1.);
#4514=VECTOR('',#15623,1.);
#4515=VECTOR('',#15624,1.);
#4516=VECTOR('',#15625,1.);
#4517=VECTOR('',#15630,1.);
#4518=VECTOR('',#15633,1.);
#4519=VECTOR('',#15634,1.);
#4520=VECTOR('',#15641,1.);
#4521=VECTOR('',#15642,1.);
#4522=VECTOR('',#15643,1.);
#4523=VECTOR('',#15644,1.);
#4524=VECTOR('',#15649,1.);
#4525=VECTOR('',#15652,1.);
#4526=VECTOR('',#15653,1.);
#4527=VECTOR('',#15660,1.);
#4528=VECTOR('',#15661,1.);
#4529=VECTOR('',#15662,1.);
#4530=VECTOR('',#15663,1.);
#4531=VECTOR('',#15668,1.);
#4532=VECTOR('',#15671,1.);
#4533=VECTOR('',#15672,1.);
#4534=VECTOR('',#15679,1.);
#4535=VECTOR('',#15680,1.);
#4536=VECTOR('',#15681,1.);
#4537=VECTOR('',#15682,1.);
#4538=VECTOR('',#15687,1.);
#4539=VECTOR('',#15690,1.);
#4540=VECTOR('',#15691,1.);
#4541=VECTOR('',#15698,1.);
#4542=VECTOR('',#15699,1.);
#4543=VECTOR('',#15700,1.);
#4544=VECTOR('',#15701,1.);
#4545=VECTOR('',#15706,1.);
#4546=VECTOR('',#15709,1.);
#4547=VECTOR('',#15710,1.);
#4548=VECTOR('',#15717,1.);
#4549=VECTOR('',#15718,1.);
#4550=VECTOR('',#15719,1.);
#4551=VECTOR('',#15720,1.);
#4552=VECTOR('',#15725,1.);
#4553=VECTOR('',#15728,1.);
#4554=VECTOR('',#15729,1.);
#4555=VECTOR('',#15736,1.);
#4556=VECTOR('',#15737,1.);
#4557=VECTOR('',#15738,1.);
#4558=VECTOR('',#15739,1.);
#4559=VECTOR('',#15744,1.);
#4560=VECTOR('',#15747,1.);
#4561=VECTOR('',#15748,1.);
#4562=VECTOR('',#15755,1.);
#4563=VECTOR('',#15756,1.);
#4564=VECTOR('',#15757,1.);
#4565=VECTOR('',#15758,1.);
#4566=VECTOR('',#15763,1.);
#4567=VECTOR('',#15766,1.);
#4568=VECTOR('',#15767,1.);
#4569=VECTOR('',#15774,1.);
#4570=VECTOR('',#15775,1.);
#4571=VECTOR('',#15776,1.);
#4572=VECTOR('',#15777,1.);
#4573=VECTOR('',#15782,1.);
#4574=VECTOR('',#15785,1.);
#4575=VECTOR('',#15786,1.);
#4576=VECTOR('',#15795,1.);
#4577=VECTOR('',#15796,1.);
#4578=VECTOR('',#15799,1.);
#4579=VECTOR('',#15800,1.);
#4580=VECTOR('',#15801,1.);
#4581=VECTOR('',#15804,1.);
#4582=VECTOR('',#15805,1.);
#4583=VECTOR('',#15812,1.);
#4584=VECTOR('',#15813,1.);
#4585=VECTOR('',#15814,1.);
#4586=VECTOR('',#15815,1.);
#4587=VECTOR('',#15820,1.);
#4588=VECTOR('',#15823,1.);
#4589=VECTOR('',#15824,1.);
#4590=VECTOR('',#15831,1.);
#4591=VECTOR('',#15832,1.);
#4592=VECTOR('',#15833,1.);
#4593=VECTOR('',#15834,1.);
#4594=VECTOR('',#15839,1.);
#4595=VECTOR('',#15842,1.);
#4596=VECTOR('',#15843,1.);
#4597=VECTOR('',#15850,1.);
#4598=VECTOR('',#15851,1.);
#4599=VECTOR('',#15852,1.);
#4600=VECTOR('',#15853,1.);
#4601=VECTOR('',#15858,1.);
#4602=VECTOR('',#15861,1.);
#4603=VECTOR('',#15862,1.);
#4604=VECTOR('',#15869,1.);
#4605=VECTOR('',#15870,1.);
#4606=VECTOR('',#15871,1.);
#4607=VECTOR('',#15872,1.);
#4608=VECTOR('',#15877,1.);
#4609=VECTOR('',#15880,1.);
#4610=VECTOR('',#15881,1.);
#4611=VECTOR('',#15888,1.);
#4612=VECTOR('',#15889,1.);
#4613=VECTOR('',#15890,1.);
#4614=VECTOR('',#15891,1.);
#4615=VECTOR('',#15896,1.);
#4616=VECTOR('',#15899,1.);
#4617=VECTOR('',#15900,1.);
#4618=VECTOR('',#15907,1.);
#4619=VECTOR('',#15908,1.);
#4620=VECTOR('',#15909,1.);
#4621=VECTOR('',#15910,1.);
#4622=VECTOR('',#15915,1.);
#4623=VECTOR('',#15918,1.);
#4624=VECTOR('',#15919,1.);
#4625=VECTOR('',#15926,1.);
#4626=VECTOR('',#15927,1.);
#4627=VECTOR('',#15928,1.);
#4628=VECTOR('',#15929,1.);
#4629=VECTOR('',#15934,1.);
#4630=VECTOR('',#15937,1.);
#4631=VECTOR('',#15938,1.);
#4632=VECTOR('',#15945,1.);
#4633=VECTOR('',#15946,1.);
#4634=VECTOR('',#15947,1.);
#4635=VECTOR('',#15948,1.);
#4636=VECTOR('',#15953,1.);
#4637=VECTOR('',#15956,1.);
#4638=VECTOR('',#15957,1.);
#4639=VECTOR('',#15964,1.);
#4640=VECTOR('',#15965,1.);
#4641=VECTOR('',#15966,1.);
#4642=VECTOR('',#15967,1.);
#4643=VECTOR('',#15972,1.);
#4644=VECTOR('',#15975,1.);
#4645=VECTOR('',#15976,1.);
#4646=VECTOR('',#15991,0.298);
#4647=VECTOR('',#16004,0.28);
#4648=VECTOR('',#16015,0.49);
#4649=VECTOR('',#16050,0.5);
#4650=VECTOR('',#16095,0.48);
#5481=VERTEX_POINT('',#26910);
#5482=VERTEX_POINT('',#26911);
#5483=VERTEX_POINT('',#26913);
#5484=VERTEX_POINT('',#26924);
#5485=VERTEX_POINT('',#26934);
#5486=VERTEX_POINT('',#26935);
#5487=VERTEX_POINT('',#26982);
#5488=VERTEX_POINT('',#26983);
#5489=VERTEX_POINT('',#27030);
#5490=VERTEX_POINT('',#27031);
#5491=VERTEX_POINT('',#27081);
#5492=VERTEX_POINT('',#27082);
#5493=VERTEX_POINT('',#27132);
#5494=VERTEX_POINT('',#27133);
#5495=VERTEX_POINT('',#27180);
#5496=VERTEX_POINT('',#27181);
#5497=VERTEX_POINT('',#27228);
#5498=VERTEX_POINT('',#27229);
#5499=VERTEX_POINT('',#27282);
#5500=VERTEX_POINT('',#27283);
#5501=VERTEX_POINT('',#27330);
#5502=VERTEX_POINT('',#27331);
#5503=VERTEX_POINT('',#27378);
#5504=VERTEX_POINT('',#27379);
#5505=VERTEX_POINT('',#27432);
#5506=VERTEX_POINT('',#27433);
#5507=VERTEX_POINT('',#27480);
#5508=VERTEX_POINT('',#27481);
#5509=VERTEX_POINT('',#27528);
#5510=VERTEX_POINT('',#27529);
#5511=VERTEX_POINT('',#27576);
#5512=VERTEX_POINT('',#27577);
#5513=VERTEX_POINT('',#27630);
#5514=VERTEX_POINT('',#27631);
#5515=VERTEX_POINT('',#27678);
#5516=VERTEX_POINT('',#27679);
#5517=VERTEX_POINT('',#27726);
#5518=VERTEX_POINT('',#27727);
#5519=VERTEX_POINT('',#27780);
#5520=VERTEX_POINT('',#27781);
#5521=VERTEX_POINT('',#27828);
#5522=VERTEX_POINT('',#27829);
#5523=VERTEX_POINT('',#27876);
#5524=VERTEX_POINT('',#27877);
#5525=VERTEX_POINT('',#27927);
#5526=VERTEX_POINT('',#27928);
#5527=VERTEX_POINT('',#27975);
#5528=VERTEX_POINT('',#27976);
#5529=VERTEX_POINT('',#28023);
#5530=VERTEX_POINT('',#28024);
#5531=VERTEX_POINT('',#28071);
#5532=VERTEX_POINT('',#28072);
#5533=VERTEX_POINT('',#28074);
#5534=VERTEX_POINT('',#28081);
#5535=VERTEX_POINT('',#28082);
#5536=VERTEX_POINT('',#28094);
#5537=VERTEX_POINT('',#28106);
#5538=VERTEX_POINT('',#28107);
#5539=VERTEX_POINT('',#28130);
#5540=VERTEX_POINT('',#28131);
#5541=VERTEX_POINT('',#28154);
#5542=VERTEX_POINT('',#28155);
#5543=VERTEX_POINT('',#28179);
#5544=VERTEX_POINT('',#28180);
#5545=VERTEX_POINT('',#28204);
#5546=VERTEX_POINT('',#28205);
#5547=VERTEX_POINT('',#28228);
#5548=VERTEX_POINT('',#28229);
#5549=VERTEX_POINT('',#28253);
#5550=VERTEX_POINT('',#28254);
#5551=VERTEX_POINT('',#28278);
#5552=VERTEX_POINT('',#28279);
#5553=VERTEX_POINT('',#28302);
#5554=VERTEX_POINT('',#28303);
#5555=VERTEX_POINT('',#28327);
#5556=VERTEX_POINT('',#28328);
#5557=VERTEX_POINT('',#28352);
#5558=VERTEX_POINT('',#28353);
#5559=VERTEX_POINT('',#28376);
#5560=VERTEX_POINT('',#28377);
#5561=VERTEX_POINT('',#28400);
#5562=VERTEX_POINT('',#28401);
#5563=VERTEX_POINT('',#28425);
#5564=VERTEX_POINT('',#28426);
#5565=VERTEX_POINT('',#28450);
#5566=VERTEX_POINT('',#28451);
#5567=VERTEX_POINT('',#28474);
#5568=VERTEX_POINT('',#28475);
#5569=VERTEX_POINT('',#28499);
#5570=VERTEX_POINT('',#28500);
#5571=VERTEX_POINT('',#28524);
#5572=VERTEX_POINT('',#28525);
#5573=VERTEX_POINT('',#28548);
#5574=VERTEX_POINT('',#28549);
#5575=VERTEX_POINT('',#28573);
#5576=VERTEX_POINT('',#28574);
#5577=VERTEX_POINT('',#28597);
#5578=VERTEX_POINT('',#28598);
#5579=VERTEX_POINT('',#28622);
#5580=VERTEX_POINT('',#28623);
#5581=VERTEX_POINT('',#29261);
#5582=VERTEX_POINT('',#29333);
#5583=VERTEX_POINT('',#29399);
#5584=VERTEX_POINT('',#29402);
#5585=VERTEX_POINT('',#30087);
#5586=VERTEX_POINT('',#30154);
#5587=VERTEX_POINT('',#30155);
#5588=VERTEX_POINT('',#30159);
#5589=VERTEX_POINT('',#30160);
#5590=VERTEX_POINT('',#30162);
#5591=VERTEX_POINT('',#30164);
#5592=VERTEX_POINT('',#30168);
#5593=VERTEX_POINT('',#30170);
#5594=VERTEX_POINT('',#30174);
#5595=VERTEX_POINT('',#30176);
#5596=VERTEX_POINT('',#30180);
#5597=VERTEX_POINT('',#30182);
#5598=VERTEX_POINT('',#30186);
#5599=VERTEX_POINT('',#30188);
#5600=VERTEX_POINT('',#30196);
#5601=VERTEX_POINT('',#30197);
#5602=VERTEX_POINT('',#30199);
#5603=VERTEX_POINT('',#30201);
#5604=VERTEX_POINT('',#30205);
#5605=VERTEX_POINT('',#30209);
#5606=VERTEX_POINT('',#30215);
#5607=VERTEX_POINT('',#30216);
#5608=VERTEX_POINT('',#30218);
#5609=VERTEX_POINT('',#30220);
#5610=VERTEX_POINT('',#30224);
#5611=VERTEX_POINT('',#30228);
#5612=VERTEX_POINT('',#30234);
#5613=VERTEX_POINT('',#30235);
#5614=VERTEX_POINT('',#30237);
#5615=VERTEX_POINT('',#30239);
#5616=VERTEX_POINT('',#30243);
#5617=VERTEX_POINT('',#30247);
#5618=VERTEX_POINT('',#30253);
#5619=VERTEX_POINT('',#30254);
#5620=VERTEX_POINT('',#30256);
#5621=VERTEX_POINT('',#30258);
#5622=VERTEX_POINT('',#30262);
#5623=VERTEX_POINT('',#30266);
#5624=VERTEX_POINT('',#30272);
#5625=VERTEX_POINT('',#30273);
#5626=VERTEX_POINT('',#30275);
#5627=VERTEX_POINT('',#30277);
#5628=VERTEX_POINT('',#30281);
#5629=VERTEX_POINT('',#30285);
#5630=VERTEX_POINT('',#30291);
#5631=VERTEX_POINT('',#30292);
#5632=VERTEX_POINT('',#30294);
#5633=VERTEX_POINT('',#30296);
#5634=VERTEX_POINT('',#30300);
#5635=VERTEX_POINT('',#30304);
#5636=VERTEX_POINT('',#30310);
#5637=VERTEX_POINT('',#30311);
#5638=VERTEX_POINT('',#30313);
#5639=VERTEX_POINT('',#30315);
#5640=VERTEX_POINT('',#30319);
#5641=VERTEX_POINT('',#30323);
#5642=VERTEX_POINT('',#30329);
#5643=VERTEX_POINT('',#30330);
#5644=VERTEX_POINT('',#30332);
#5645=VERTEX_POINT('',#30334);
#5646=VERTEX_POINT('',#30338);
#5647=VERTEX_POINT('',#30342);
#5648=VERTEX_POINT('',#30348);
#5649=VERTEX_POINT('',#30349);
#5650=VERTEX_POINT('',#30351);
#5651=VERTEX_POINT('',#30353);
#5652=VERTEX_POINT('',#30357);
#5653=VERTEX_POINT('',#30359);
#5654=VERTEX_POINT('',#30363);
#5655=VERTEX_POINT('',#30367);
#5656=VERTEX_POINT('',#30371);
#5657=VERTEX_POINT('',#30372);
#5658=VERTEX_POINT('',#30374);
#5659=VERTEX_POINT('',#30376);
#5660=VERTEX_POINT('',#30380);
#5661=VERTEX_POINT('',#30384);
#5662=VERTEX_POINT('',#30390);
#5663=VERTEX_POINT('',#30391);
#5664=VERTEX_POINT('',#30393);
#5665=VERTEX_POINT('',#30395);
#5666=VERTEX_POINT('',#30399);
#5667=VERTEX_POINT('',#30403);
#5668=VERTEX_POINT('',#30409);
#5669=VERTEX_POINT('',#30410);
#5670=VERTEX_POINT('',#30412);
#5671=VERTEX_POINT('',#30414);
#5672=VERTEX_POINT('',#30418);
#5673=VERTEX_POINT('',#30422);
#5674=VERTEX_POINT('',#30428);
#5675=VERTEX_POINT('',#30429);
#5676=VERTEX_POINT('',#30431);
#5677=VERTEX_POINT('',#30433);
#5678=VERTEX_POINT('',#30437);
#5679=VERTEX_POINT('',#30441);
#5680=VERTEX_POINT('',#30447);
#5681=VERTEX_POINT('',#30448);
#5682=VERTEX_POINT('',#30450);
#5683=VERTEX_POINT('',#30452);
#5684=VERTEX_POINT('',#30456);
#5685=VERTEX_POINT('',#30460);
#5686=VERTEX_POINT('',#30466);
#5687=VERTEX_POINT('',#30467);
#5688=VERTEX_POINT('',#30469);
#5689=VERTEX_POINT('',#30471);
#5690=VERTEX_POINT('',#30475);
#5691=VERTEX_POINT('',#30479);
#5692=VERTEX_POINT('',#30485);
#5693=VERTEX_POINT('',#30486);
#5694=VERTEX_POINT('',#30488);
#5695=VERTEX_POINT('',#30490);
#5696=VERTEX_POINT('',#30494);
#5697=VERTEX_POINT('',#30498);
#5698=VERTEX_POINT('',#30504);
#5699=VERTEX_POINT('',#30505);
#5700=VERTEX_POINT('',#30507);
#5701=VERTEX_POINT('',#30509);
#5702=VERTEX_POINT('',#30513);
#5703=VERTEX_POINT('',#30517);
#5704=VERTEX_POINT('',#30523);
#5705=VERTEX_POINT('',#30524);
#5706=VERTEX_POINT('',#30526);
#5707=VERTEX_POINT('',#30528);
#5708=VERTEX_POINT('',#30532);
#5709=VERTEX_POINT('',#30536);
#5710=VERTEX_POINT('',#30542);
#5711=VERTEX_POINT('',#30543);
#5712=VERTEX_POINT('',#30545);
#5713=VERTEX_POINT('',#30547);
#5714=VERTEX_POINT('',#30551);
#5715=VERTEX_POINT('',#30555);
#5716=VERTEX_POINT('',#30561);
#5717=VERTEX_POINT('',#30562);
#5718=VERTEX_POINT('',#30564);
#5719=VERTEX_POINT('',#30566);
#5720=VERTEX_POINT('',#30570);
#5721=VERTEX_POINT('',#30574);
#5722=VERTEX_POINT('',#30580);
#5723=VERTEX_POINT('',#30581);
#5724=VERTEX_POINT('',#30583);
#5725=VERTEX_POINT('',#30585);
#5726=VERTEX_POINT('',#30589);
#5727=VERTEX_POINT('',#30593);
#5728=VERTEX_POINT('',#30599);
#5729=VERTEX_POINT('',#30600);
#5730=VERTEX_POINT('',#30602);
#5731=VERTEX_POINT('',#30604);
#5732=VERTEX_POINT('',#30608);
#5733=VERTEX_POINT('',#30612);
#5734=VERTEX_POINT('',#30618);
#5735=VERTEX_POINT('',#30619);
#5736=VERTEX_POINT('',#30621);
#5737=VERTEX_POINT('',#30623);
#5738=VERTEX_POINT('',#30627);
#5739=VERTEX_POINT('',#30631);
#5740=VERTEX_POINT('',#30637);
#5741=VERTEX_POINT('',#30638);
#5742=VERTEX_POINT('',#30640);
#5743=VERTEX_POINT('',#30642);
#5744=VERTEX_POINT('',#30646);
#5745=VERTEX_POINT('',#30650);
#5746=VERTEX_POINT('',#30656);
#5747=VERTEX_POINT('',#30657);
#5748=VERTEX_POINT('',#30659);
#5749=VERTEX_POINT('',#30661);
#5750=VERTEX_POINT('',#30665);
#5751=VERTEX_POINT('',#30669);
#5752=VERTEX_POINT('',#30675);
#5753=VERTEX_POINT('',#30676);
#5754=VERTEX_POINT('',#30678);
#5755=VERTEX_POINT('',#30680);
#5756=VERTEX_POINT('',#30684);
#5757=VERTEX_POINT('',#30688);
#5758=VERTEX_POINT('',#30694);
#5759=VERTEX_POINT('',#30695);
#5760=VERTEX_POINT('',#30697);
#5761=VERTEX_POINT('',#30701);
#5762=VERTEX_POINT('',#30703);
#5763=VERTEX_POINT('',#30707);
#5764=VERTEX_POINT('',#30713);
#5765=VERTEX_POINT('',#30714);
#5766=VERTEX_POINT('',#30716);
#5767=VERTEX_POINT('',#30718);
#5768=VERTEX_POINT('',#30722);
#5769=VERTEX_POINT('',#30726);
#5770=VERTEX_POINT('',#30732);
#5771=VERTEX_POINT('',#30733);
#5772=VERTEX_POINT('',#30735);
#5773=VERTEX_POINT('',#30737);
#5774=VERTEX_POINT('',#30741);
#5775=VERTEX_POINT('',#30745);
#5776=VERTEX_POINT('',#30751);
#5777=VERTEX_POINT('',#30752);
#5778=VERTEX_POINT('',#30754);
#5779=VERTEX_POINT('',#30756);
#5780=VERTEX_POINT('',#30760);
#5781=VERTEX_POINT('',#30764);
#5782=VERTEX_POINT('',#30770);
#5783=VERTEX_POINT('',#30771);
#5784=VERTEX_POINT('',#30773);
#5785=VERTEX_POINT('',#30775);
#5786=VERTEX_POINT('',#30779);
#5787=VERTEX_POINT('',#30783);
#5788=VERTEX_POINT('',#30789);
#5789=VERTEX_POINT('',#30790);
#5790=VERTEX_POINT('',#30792);
#5791=VERTEX_POINT('',#30794);
#5792=VERTEX_POINT('',#30798);
#5793=VERTEX_POINT('',#30802);
#5794=VERTEX_POINT('',#30808);
#5795=VERTEX_POINT('',#30809);
#5796=VERTEX_POINT('',#30811);
#5797=VERTEX_POINT('',#30813);
#5798=VERTEX_POINT('',#30817);
#5799=VERTEX_POINT('',#30821);
#5800=VERTEX_POINT('',#30827);
#5801=VERTEX_POINT('',#30828);
#5802=VERTEX_POINT('',#30830);
#5803=VERTEX_POINT('',#30832);
#5804=VERTEX_POINT('',#30836);
#5805=VERTEX_POINT('',#30840);
#5806=VERTEX_POINT('',#30846);
#5807=VERTEX_POINT('',#30847);
#5808=VERTEX_POINT('',#30849);
#5809=VERTEX_POINT('',#30851);
#5810=VERTEX_POINT('',#30855);
#5811=VERTEX_POINT('',#30859);
#5812=VERTEX_POINT('',#30865);
#5813=VERTEX_POINT('',#30866);
#5814=VERTEX_POINT('',#30868);
#5815=VERTEX_POINT('',#30870);
#5816=VERTEX_POINT('',#30874);
#5817=VERTEX_POINT('',#30878);
#5818=VERTEX_POINT('',#30884);
#5819=VERTEX_POINT('',#30886);
#5820=VERTEX_POINT('',#30890);
#5821=VERTEX_POINT('',#30894);
#5822=VERTEX_POINT('',#30897);
#5823=VERTEX_POINT('',#30905);
#5824=VERTEX_POINT('',#30947);
#7094=EDGE_CURVE('',#5481,#5482,#3622,.T.);
#7095=EDGE_CURVE('',#5481,#5483,#1046,.T.);
#7096=EDGE_CURVE('',#5483,#5484,#1668,.T.);
#7097=EDGE_CURVE('',#5484,#5482,#1047,.T.);
#7098=EDGE_CURVE('',#5485,#5486,#3623,.T.);
#7099=EDGE_CURVE('',#5485,#5481,#1048,.T.);
#7100=EDGE_CURVE('',#5482,#5486,#1049,.T.);
#7101=EDGE_CURVE('',#5487,#5488,#3624,.T.);
#7102=EDGE_CURVE('',#5487,#5485,#1050,.T.);
#7103=EDGE_CURVE('',#5486,#5488,#1051,.T.);
#7104=EDGE_CURVE('',#5489,#5490,#3625,.T.);
#7105=EDGE_CURVE('',#5489,#5487,#1052,.T.);
#7106=EDGE_CURVE('',#5488,#5490,#1053,.T.);
#7107=EDGE_CURVE('',#5491,#5492,#3626,.T.);
#7108=EDGE_CURVE('',#5491,#5489,#1054,.T.);
#7109=EDGE_CURVE('',#5490,#5492,#1055,.T.);
#7110=EDGE_CURVE('',#5493,#5494,#3627,.T.);
#7111=EDGE_CURVE('',#5493,#5491,#1056,.T.);
#7112=EDGE_CURVE('',#5492,#5494,#1057,.T.);
#7113=EDGE_CURVE('',#5495,#5496,#3628,.T.);
#7114=EDGE_CURVE('',#5495,#5493,#1058,.T.);
#7115=EDGE_CURVE('',#5494,#5496,#1059,.T.);
#7116=EDGE_CURVE('',#5497,#5498,#3629,.T.);
#7117=EDGE_CURVE('',#5497,#5495,#1060,.T.);
#7118=EDGE_CURVE('',#5496,#5498,#1061,.T.);
#7119=EDGE_CURVE('',#5499,#5500,#3630,.T.);
#7120=EDGE_CURVE('',#5499,#5497,#1062,.T.);
#7121=EDGE_CURVE('',#5498,#5500,#1063,.T.);
#7122=EDGE_CURVE('',#5501,#5502,#3631,.T.);
#7123=EDGE_CURVE('',#5501,#5499,#1064,.T.);
#7124=EDGE_CURVE('',#5500,#5502,#1065,.T.);
#7125=EDGE_CURVE('',#5503,#5504,#3632,.T.);
#7126=EDGE_CURVE('',#5503,#5501,#1066,.T.);
#7127=EDGE_CURVE('',#5502,#5504,#1067,.T.);
#7128=EDGE_CURVE('',#5505,#5506,#3633,.T.);
#7129=EDGE_CURVE('',#5505,#5503,#1068,.T.);
#7130=EDGE_CURVE('',#5504,#5506,#1069,.T.);
#7131=EDGE_CURVE('',#5507,#5508,#3634,.T.);
#7132=EDGE_CURVE('',#5507,#5505,#1070,.T.);
#7133=EDGE_CURVE('',#5506,#5508,#1071,.T.);
#7134=EDGE_CURVE('',#5509,#5510,#3635,.T.);
#7135=EDGE_CURVE('',#5509,#5507,#1072,.T.);
#7136=EDGE_CURVE('',#5508,#5510,#1073,.T.);
#7137=EDGE_CURVE('',#5511,#5512,#3636,.T.);
#7138=EDGE_CURVE('',#5511,#5509,#1074,.T.);
#7139=EDGE_CURVE('',#5510,#5512,#1075,.T.);
#7140=EDGE_CURVE('',#5513,#5514,#3637,.T.);
#7141=EDGE_CURVE('',#5513,#5511,#1076,.T.);
#7142=EDGE_CURVE('',#5512,#5514,#1077,.T.);
#7143=EDGE_CURVE('',#5515,#5516,#3638,.T.);
#7144=EDGE_CURVE('',#5515,#5513,#1078,.T.);
#7145=EDGE_CURVE('',#5514,#5516,#1079,.T.);
#7146=EDGE_CURVE('',#5517,#5518,#3639,.T.);
#7147=EDGE_CURVE('',#5517,#5515,#1080,.T.);
#7148=EDGE_CURVE('',#5516,#5518,#1081,.T.);
#7149=EDGE_CURVE('',#5519,#5520,#3640,.T.);
#7150=EDGE_CURVE('',#5519,#5517,#1082,.T.);
#7151=EDGE_CURVE('',#5518,#5520,#1083,.T.);
#7152=EDGE_CURVE('',#5521,#5522,#3641,.T.);
#7153=EDGE_CURVE('',#5521,#5519,#1084,.T.);
#7154=EDGE_CURVE('',#5520,#5522,#1085,.T.);
#7155=EDGE_CURVE('',#5523,#5524,#3642,.T.);
#7156=EDGE_CURVE('',#5523,#5521,#1086,.T.);
#7157=EDGE_CURVE('',#5522,#5524,#1087,.T.);
#7158=EDGE_CURVE('',#5525,#5526,#3643,.T.);
#7159=EDGE_CURVE('',#5525,#5523,#1088,.T.);
#7160=EDGE_CURVE('',#5524,#5526,#1089,.T.);
#7161=EDGE_CURVE('',#5527,#5528,#3644,.T.);
#7162=EDGE_CURVE('',#5527,#5525,#1090,.T.);
#7163=EDGE_CURVE('',#5526,#5528,#1091,.T.);
#7164=EDGE_CURVE('',#5529,#5530,#3645,.T.);
#7165=EDGE_CURVE('',#5529,#5527,#1092,.T.);
#7166=EDGE_CURVE('',#5528,#5530,#1093,.T.);
#7167=EDGE_CURVE('',#5531,#5532,#3646,.T.);
#7168=EDGE_CURVE('',#5531,#5533,#1094,.T.);
#7169=EDGE_CURVE('',#5532,#5533,#1669,.T.);
#7170=EDGE_CURVE('',#5534,#5535,#3647,.T.);
#7171=EDGE_CURVE('',#5534,#5531,#1095,.T.);
#7172=EDGE_CURVE('',#5536,#5532,#1670,.T.);
#7173=EDGE_CURVE('',#5535,#5536,#1096,.T.);
#7174=EDGE_CURVE('',#5537,#5538,#3648,.T.);
#7175=EDGE_CURVE('',#5537,#5534,#1097,.T.);
#7176=EDGE_CURVE('',#5538,#5535,#1098,.T.);
#7177=EDGE_CURVE('',#5539,#5540,#3649,.T.);
#7178=EDGE_CURVE('',#5539,#5537,#1099,.T.);
#7179=EDGE_CURVE('',#5540,#5538,#1100,.T.);
#7180=EDGE_CURVE('',#5541,#5542,#3650,.T.);
#7181=EDGE_CURVE('',#5541,#5539,#1101,.T.);
#7182=EDGE_CURVE('',#5542,#5540,#1102,.T.);
#7183=EDGE_CURVE('',#5543,#5544,#3651,.T.);
#7184=EDGE_CURVE('',#5543,#5541,#1103,.T.);
#7185=EDGE_CURVE('',#5544,#5542,#1104,.T.);
#7186=EDGE_CURVE('',#5545,#5546,#3652,.T.);
#7187=EDGE_CURVE('',#5545,#5543,#1105,.T.);
#7188=EDGE_CURVE('',#5546,#5544,#1106,.T.);
#7189=EDGE_CURVE('',#5547,#5548,#3653,.T.);
#7190=EDGE_CURVE('',#5547,#5545,#1107,.T.);
#7191=EDGE_CURVE('',#5548,#5546,#1108,.T.);
#7192=EDGE_CURVE('',#5549,#5550,#3654,.T.);
#7193=EDGE_CURVE('',#5549,#5547,#1109,.T.);
#7194=EDGE_CURVE('',#5550,#5548,#1110,.T.);
#7195=EDGE_CURVE('',#5551,#5552,#3655,.T.);
#7196=EDGE_CURVE('',#5551,#5549,#1111,.T.);
#7197=EDGE_CURVE('',#5552,#5550,#1112,.T.);
#7198=EDGE_CURVE('',#5553,#5554,#3656,.T.);
#7199=EDGE_CURVE('',#5553,#5551,#1113,.T.);
#7200=EDGE_CURVE('',#5554,#5552,#1114,.T.);
#7201=EDGE_CURVE('',#5555,#5556,#3657,.T.);
#7202=EDGE_CURVE('',#5555,#5553,#1115,.T.);
#7203=EDGE_CURVE('',#5556,#5554,#1116,.T.);
#7204=EDGE_CURVE('',#5557,#5558,#3658,.T.);
#7205=EDGE_CURVE('',#5557,#5555,#1117,.T.);
#7206=EDGE_CURVE('',#5558,#5556,#1118,.T.);
#7207=EDGE_CURVE('',#5559,#5560,#3659,.T.);
#7208=EDGE_CURVE('',#5559,#5557,#1119,.T.);
#7209=EDGE_CURVE('',#5560,#5558,#1120,.T.);
#7210=EDGE_CURVE('',#5561,#5562,#3660,.T.);
#7211=EDGE_CURVE('',#5561,#5559,#1121,.T.);
#7212=EDGE_CURVE('',#5562,#5560,#1122,.T.);
#7213=EDGE_CURVE('',#5563,#5564,#3661,.T.);
#7214=EDGE_CURVE('',#5563,#5561,#1123,.T.);
#7215=EDGE_CURVE('',#5564,#5562,#1124,.T.);
#7216=EDGE_CURVE('',#5565,#5566,#3662,.T.);
#7217=EDGE_CURVE('',#5565,#5563,#1125,.T.);
#7218=EDGE_CURVE('',#5566,#5564,#1126,.T.);
#7219=EDGE_CURVE('',#5567,#5568,#3663,.T.);
#7220=EDGE_CURVE('',#5567,#5565,#1127,.T.);
#7221=EDGE_CURVE('',#5568,#5566,#1128,.T.);
#7222=EDGE_CURVE('',#5569,#5570,#3664,.T.);
#7223=EDGE_CURVE('',#5569,#5567,#1129,.T.);
#7224=EDGE_CURVE('',#5570,#5568,#1130,.T.);
#7225=EDGE_CURVE('',#5571,#5572,#3665,.T.);
#7226=EDGE_CURVE('',#5571,#5569,#1131,.T.);
#7227=EDGE_CURVE('',#5572,#5570,#1132,.T.);
#7228=EDGE_CURVE('',#5573,#5574,#3666,.T.);
#7229=EDGE_CURVE('',#5573,#5571,#1133,.T.);
#7230=EDGE_CURVE('',#5574,#5572,#1134,.T.);
#7231=EDGE_CURVE('',#5575,#5576,#3667,.T.);
#7232=EDGE_CURVE('',#5575,#5573,#1135,.T.);
#7233=EDGE_CURVE('',#5576,#5574,#1136,.T.);
#7234=EDGE_CURVE('',#5577,#5578,#3668,.T.);
#7235=EDGE_CURVE('',#5577,#5575,#1137,.T.);
#7236=EDGE_CURVE('',#5578,#5576,#1138,.T.);
#7237=EDGE_CURVE('',#5579,#5580,#3669,.T.);
#7238=EDGE_CURVE('',#5579,#5577,#1139,.T.);
#7239=EDGE_CURVE('',#5580,#5578,#1140,.T.);
#7240=EDGE_CURVE('',#5581,#5536,#1141,.T.);
#7241=EDGE_CURVE('',#5530,#5581,#1142,.T.);
#7242=EDGE_CURVE('',#5582,#5484,#1143,.T.);
#7243=EDGE_CURVE('',#5582,#5580,#1144,.T.);
#7244=EDGE_CURVE('',#5484,#5583,#1671,.T.);
#7245=EDGE_CURVE('',#5583,#5483,#1672,.T.);
#7246=EDGE_CURVE('',#5483,#5584,#1145,.T.);
#7247=EDGE_CURVE('',#5584,#5582,#1673,.T.);
#7248=EDGE_CURVE('',#5584,#5579,#1146,.T.);
#7249=EDGE_CURVE('',#5533,#5585,#1147,.T.);
#7250=EDGE_CURVE('',#5585,#5529,#1148,.T.);
#7251=EDGE_CURVE('',#5586,#5587,#3670,.T.);
#7252=EDGE_CURVE('',#5587,#5587,#1674,.T.);
#7253=EDGE_CURVE('',#5588,#5589,#3671,.T.);
#7254=EDGE_CURVE('',#5588,#5590,#3672,.T.);
#7255=EDGE_CURVE('',#5590,#5591,#3673,.T.);
#7256=EDGE_CURVE('',#5589,#5591,#3674,.T.);
#7257=EDGE_CURVE('',#5592,#5588,#3675,.T.);
#7258=EDGE_CURVE('',#5592,#5593,#3676,.T.);
#7259=EDGE_CURVE('',#5593,#5590,#3677,.T.);
#7260=EDGE_CURVE('',#5594,#5592,#3678,.T.);
#7261=EDGE_CURVE('',#5594,#5595,#3679,.T.);
#7262=EDGE_CURVE('',#5595,#5593,#3680,.T.);
#7263=EDGE_CURVE('',#5596,#5594,#3681,.T.);
#7264=EDGE_CURVE('',#5596,#5597,#3682,.T.);
#7265=EDGE_CURVE('',#5597,#5595,#3683,.T.);
#7266=EDGE_CURVE('',#5598,#5596,#3684,.T.);
#7267=EDGE_CURVE('',#5598,#5599,#3685,.T.);
#7268=EDGE_CURVE('',#5599,#5597,#3686,.T.);
#7269=EDGE_CURVE('',#5589,#5598,#3687,.T.);
#7270=EDGE_CURVE('',#5591,#5599,#3688,.T.);
#7271=EDGE_CURVE('',#5600,#5601,#3689,.T.);
#7272=EDGE_CURVE('',#5600,#5602,#3690,.T.);
#7273=EDGE_CURVE('',#5603,#5602,#3691,.T.);
#7274=EDGE_CURVE('',#5601,#5603,#3692,.T.);
#7275=EDGE_CURVE('',#5601,#5604,#1675,.T.);
#7276=EDGE_CURVE('',#5603,#5604,#3693,.T.);
#7277=EDGE_CURVE('',#5604,#5605,#3694,.T.);
#7278=EDGE_CURVE('',#5602,#5605,#3695,.T.);
#7279=EDGE_CURVE('',#5605,#5600,#1676,.T.);
#7280=EDGE_CURVE('',#5606,#5607,#3696,.T.);
#7281=EDGE_CURVE('',#5606,#5608,#3697,.T.);
#7282=EDGE_CURVE('',#5609,#5608,#3698,.T.);
#7283=EDGE_CURVE('',#5607,#5609,#3699,.T.);
#7284=EDGE_CURVE('',#5607,#5610,#1677,.T.);
#7285=EDGE_CURVE('',#5609,#5610,#3700,.T.);
#7286=EDGE_CURVE('',#5610,#5611,#3701,.T.);
#7287=EDGE_CURVE('',#5608,#5611,#3702,.T.);
#7288=EDGE_CURVE('',#5611,#5606,#1678,.T.);
#7289=EDGE_CURVE('',#5612,#5613,#3703,.T.);
#7290=EDGE_CURVE('',#5612,#5614,#3704,.T.);
#7291=EDGE_CURVE('',#5615,#5614,#3705,.T.);
#7292=EDGE_CURVE('',#5613,#5615,#3706,.T.);
#7293=EDGE_CURVE('',#5613,#5616,#1679,.T.);
#7294=EDGE_CURVE('',#5615,#5616,#3707,.T.);
#7295=EDGE_CURVE('',#5616,#5617,#3708,.T.);
#7296=EDGE_CURVE('',#5614,#5617,#3709,.T.);
#7297=EDGE_CURVE('',#5617,#5612,#1680,.T.);
#7298=EDGE_CURVE('',#5618,#5619,#3710,.T.);
#7299=EDGE_CURVE('',#5618,#5620,#3711,.T.);
#7300=EDGE_CURVE('',#5621,#5620,#3712,.T.);
#7301=EDGE_CURVE('',#5619,#5621,#3713,.T.);
#7302=EDGE_CURVE('',#5619,#5622,#1681,.T.);
#7303=EDGE_CURVE('',#5621,#5622,#3714,.T.);
#7304=EDGE_CURVE('',#5622,#5623,#3715,.T.);
#7305=EDGE_CURVE('',#5620,#5623,#3716,.T.);
#7306=EDGE_CURVE('',#5623,#5618,#1682,.T.);
#7307=EDGE_CURVE('',#5624,#5625,#3717,.T.);
#7308=EDGE_CURVE('',#5624,#5626,#3718,.T.);
#7309=EDGE_CURVE('',#5627,#5626,#3719,.T.);
#7310=EDGE_CURVE('',#5625,#5627,#3720,.T.);
#7311=EDGE_CURVE('',#5625,#5628,#1683,.T.);
#7312=EDGE_CURVE('',#5627,#5628,#3721,.T.);
#7313=EDGE_CURVE('',#5628,#5629,#3722,.T.);
#7314=EDGE_CURVE('',#5626,#5629,#3723,.T.);
#7315=EDGE_CURVE('',#5629,#5624,#1684,.T.);
#7316=EDGE_CURVE('',#5630,#5631,#3724,.T.);
#7317=EDGE_CURVE('',#5630,#5632,#3725,.T.);
#7318=EDGE_CURVE('',#5633,#5632,#3726,.T.);
#7319=EDGE_CURVE('',#5631,#5633,#3727,.T.);
#7320=EDGE_CURVE('',#5631,#5634,#1685,.T.);
#7321=EDGE_CURVE('',#5633,#5634,#3728,.T.);
#7322=EDGE_CURVE('',#5634,#5635,#3729,.T.);
#7323=EDGE_CURVE('',#5632,#5635,#3730,.T.);
#7324=EDGE_CURVE('',#5635,#5630,#1686,.T.);
#7325=EDGE_CURVE('',#5636,#5637,#3731,.T.);
#7326=EDGE_CURVE('',#5636,#5638,#3732,.T.);
#7327=EDGE_CURVE('',#5639,#5638,#3733,.T.);
#7328=EDGE_CURVE('',#5637,#5639,#3734,.T.);
#7329=EDGE_CURVE('',#5637,#5640,#1687,.T.);
#7330=EDGE_CURVE('',#5639,#5640,#3735,.T.);
#7331=EDGE_CURVE('',#5640,#5641,#3736,.T.);
#7332=EDGE_CURVE('',#5638,#5641,#3737,.T.);
#7333=EDGE_CURVE('',#5641,#5636,#1688,.T.);
#7334=EDGE_CURVE('',#5642,#5643,#3738,.T.);
#7335=EDGE_CURVE('',#5642,#5644,#3739,.T.);
#7336=EDGE_CURVE('',#5645,#5644,#3740,.T.);
#7337=EDGE_CURVE('',#5643,#5645,#3741,.T.);
#7338=EDGE_CURVE('',#5643,#5646,#1689,.T.);
#7339=EDGE_CURVE('',#5645,#5646,#3742,.T.);
#7340=EDGE_CURVE('',#5646,#5647,#3743,.T.);
#7341=EDGE_CURVE('',#5644,#5647,#3744,.T.);
#7342=EDGE_CURVE('',#5647,#5642,#1690,.T.);
#7343=EDGE_CURVE('',#5648,#5649,#3745,.T.);
#7344=EDGE_CURVE('',#5648,#5650,#3746,.T.);
#7345=EDGE_CURVE('',#5651,#5650,#3747,.T.);
#7346=EDGE_CURVE('',#5649,#5651,#3748,.T.);
#7347=EDGE_CURVE('',#5649,#5652,#1691,.T.);
#7348=EDGE_CURVE('',#5651,#5653,#3749,.T.);
#7349=EDGE_CURVE('',#5652,#5653,#1692,.T.);
#7350=EDGE_CURVE('',#5653,#5654,#3750,.T.);
#7351=EDGE_CURVE('',#5650,#5654,#3751,.T.);
#7352=EDGE_CURVE('',#5654,#5655,#1693,.T.);
#7353=EDGE_CURVE('',#5655,#5648,#1694,.T.);
#7354=EDGE_CURVE('',#5656,#5657,#3752,.T.);
#7355=EDGE_CURVE('',#5656,#5658,#3753,.T.);
#7356=EDGE_CURVE('',#5659,#5658,#3754,.T.);
#7357=EDGE_CURVE('',#5657,#5659,#3755,.T.);
#7358=EDGE_CURVE('',#5657,#5660,#1695,.T.);
#7359=EDGE_CURVE('',#5659,#5660,#3756,.T.);
#7360=EDGE_CURVE('',#5660,#5661,#3757,.T.);
#7361=EDGE_CURVE('',#5658,#5661,#3758,.T.);
#7362=EDGE_CURVE('',#5661,#5656,#1696,.T.);
#7363=EDGE_CURVE('',#5662,#5663,#3759,.T.);
#7364=EDGE_CURVE('',#5662,#5664,#3760,.T.);
#7365=EDGE_CURVE('',#5665,#5664,#3761,.T.);
#7366=EDGE_CURVE('',#5663,#5665,#3762,.T.);
#7367=EDGE_CURVE('',#5663,#5666,#1697,.T.);
#7368=EDGE_CURVE('',#5665,#5666,#3763,.T.);
#7369=EDGE_CURVE('',#5666,#5667,#3764,.T.);
#7370=EDGE_CURVE('',#5664,#5667,#3765,.T.);
#7371=EDGE_CURVE('',#5667,#5662,#1698,.T.);
#7372=EDGE_CURVE('',#5668,#5669,#3766,.T.);
#7373=EDGE_CURVE('',#5668,#5670,#3767,.T.);
#7374=EDGE_CURVE('',#5671,#5670,#3768,.T.);
#7375=EDGE_CURVE('',#5669,#5671,#3769,.T.);
#7376=EDGE_CURVE('',#5669,#5672,#1699,.T.);
#7377=EDGE_CURVE('',#5671,#5672,#3770,.T.);
#7378=EDGE_CURVE('',#5672,#5673,#3771,.T.);
#7379=EDGE_CURVE('',#5670,#5673,#3772,.T.);
#7380=EDGE_CURVE('',#5673,#5668,#1700,.T.);
#7381=EDGE_CURVE('',#5674,#5675,#3773,.T.);
#7382=EDGE_CURVE('',#5674,#5676,#3774,.T.);
#7383=EDGE_CURVE('',#5677,#5676,#3775,.T.);
#7384=EDGE_CURVE('',#5675,#5677,#3776,.T.);
#7385=EDGE_CURVE('',#5675,#5678,#1701,.T.);
#7386=EDGE_CURVE('',#5677,#5678,#3777,.T.);
#7387=EDGE_CURVE('',#5678,#5679,#3778,.T.);
#7388=EDGE_CURVE('',#5676,#5679,#3779,.T.);
#7389=EDGE_CURVE('',#5679,#5674,#1702,.T.);
#7390=EDGE_CURVE('',#5680,#5681,#3780,.T.);
#7391=EDGE_CURVE('',#5680,#5682,#3781,.T.);
#7392=EDGE_CURVE('',#5683,#5682,#3782,.T.);
#7393=EDGE_CURVE('',#5681,#5683,#3783,.T.);
#7394=EDGE_CURVE('',#5681,#5684,#1703,.T.);
#7395=EDGE_CURVE('',#5683,#5684,#3784,.T.);
#7396=EDGE_CURVE('',#5684,#5685,#3785,.T.);
#7397=EDGE_CURVE('',#5682,#5685,#3786,.T.);
#7398=EDGE_CURVE('',#5685,#5680,#1704,.T.);
#7399=EDGE_CURVE('',#5686,#5687,#3787,.T.);
#7400=EDGE_CURVE('',#5686,#5688,#3788,.T.);
#7401=EDGE_CURVE('',#5689,#5688,#3789,.T.);
#7402=EDGE_CURVE('',#5687,#5689,#3790,.T.);
#7403=EDGE_CURVE('',#5687,#5690,#1705,.T.);
#7404=EDGE_CURVE('',#5689,#5690,#3791,.T.);
#7405=EDGE_CURVE('',#5690,#5691,#3792,.T.);
#7406=EDGE_CURVE('',#5688,#5691,#3793,.T.);
#7407=EDGE_CURVE('',#5691,#5686,#1706,.T.);
#7408=EDGE_CURVE('',#5692,#5693,#3794,.T.);
#7409=EDGE_CURVE('',#5692,#5694,#3795,.T.);
#7410=EDGE_CURVE('',#5695,#5694,#3796,.T.);
#7411=EDGE_CURVE('',#5693,#5695,#3797,.T.);
#7412=EDGE_CURVE('',#5693,#5696,#1707,.T.);
#7413=EDGE_CURVE('',#5695,#5696,#3798,.T.);
#7414=EDGE_CURVE('',#5696,#5697,#3799,.T.);
#7415=EDGE_CURVE('',#5694,#5697,#3800,.T.);
#7416=EDGE_CURVE('',#5697,#5692,#1708,.T.);
#7417=EDGE_CURVE('',#5698,#5699,#3801,.T.);
#7418=EDGE_CURVE('',#5698,#5700,#3802,.T.);
#7419=EDGE_CURVE('',#5701,#5700,#3803,.T.);
#7420=EDGE_CURVE('',#5699,#5701,#3804,.T.);
#7421=EDGE_CURVE('',#5699,#5702,#1709,.T.);
#7422=EDGE_CURVE('',#5701,#5702,#3805,.T.);
#7423=EDGE_CURVE('',#5702,#5703,#3806,.T.);
#7424=EDGE_CURVE('',#5700,#5703,#3807,.T.);
#7425=EDGE_CURVE('',#5703,#5698,#1710,.T.);
#7426=EDGE_CURVE('',#5704,#5705,#3808,.T.);
#7427=EDGE_CURVE('',#5704,#5706,#3809,.T.);
#7428=EDGE_CURVE('',#5707,#5706,#3810,.T.);
#7429=EDGE_CURVE('',#5705,#5707,#3811,.T.);
#7430=EDGE_CURVE('',#5705,#5708,#1711,.T.);
#7431=EDGE_CURVE('',#5707,#5708,#3812,.T.);
#7432=EDGE_CURVE('',#5708,#5709,#3813,.T.);
#7433=EDGE_CURVE('',#5706,#5709,#3814,.T.);
#7434=EDGE_CURVE('',#5709,#5704,#1712,.T.);
#7435=EDGE_CURVE('',#5710,#5711,#3815,.T.);
#7436=EDGE_CURVE('',#5710,#5712,#3816,.T.);
#7437=EDGE_CURVE('',#5713,#5712,#3817,.T.);
#7438=EDGE_CURVE('',#5711,#5713,#3818,.T.);
#7439=EDGE_CURVE('',#5711,#5714,#1713,.T.);
#7440=EDGE_CURVE('',#5713,#5714,#3819,.T.);
#7441=EDGE_CURVE('',#5714,#5715,#3820,.T.);
#7442=EDGE_CURVE('',#5712,#5715,#3821,.T.);
#7443=EDGE_CURVE('',#5715,#5710,#1714,.T.);
#7444=EDGE_CURVE('',#5716,#5717,#3822,.T.);
#7445=EDGE_CURVE('',#5716,#5718,#3823,.T.);
#7446=EDGE_CURVE('',#5719,#5718,#3824,.T.);
#7447=EDGE_CURVE('',#5717,#5719,#3825,.T.);
#7448=EDGE_CURVE('',#5717,#5720,#1715,.T.);
#7449=EDGE_CURVE('',#5719,#5720,#3826,.T.);
#7450=EDGE_CURVE('',#5720,#5721,#3827,.T.);
#7451=EDGE_CURVE('',#5718,#5721,#3828,.T.);
#7452=EDGE_CURVE('',#5721,#5716,#1716,.T.);
#7453=EDGE_CURVE('',#5722,#5723,#3829,.T.);
#7454=EDGE_CURVE('',#5722,#5724,#3830,.T.);
#7455=EDGE_CURVE('',#5725,#5724,#3831,.T.);
#7456=EDGE_CURVE('',#5723,#5725,#3832,.T.);
#7457=EDGE_CURVE('',#5723,#5726,#1717,.T.);
#7458=EDGE_CURVE('',#5725,#5726,#3833,.T.);
#7459=EDGE_CURVE('',#5726,#5727,#3834,.T.);
#7460=EDGE_CURVE('',#5724,#5727,#3835,.T.);
#7461=EDGE_CURVE('',#5727,#5722,#1718,.T.);
#7462=EDGE_CURVE('',#5728,#5729,#3836,.T.);
#7463=EDGE_CURVE('',#5728,#5730,#3837,.T.);
#7464=EDGE_CURVE('',#5731,#5730,#3838,.T.);
#7465=EDGE_CURVE('',#5729,#5731,#3839,.T.);
#7466=EDGE_CURVE('',#5729,#5732,#1719,.T.);
#7467=EDGE_CURVE('',#5731,#5732,#3840,.T.);
#7468=EDGE_CURVE('',#5732,#5733,#3841,.T.);
#7469=EDGE_CURVE('',#5730,#5733,#3842,.T.);
#7470=EDGE_CURVE('',#5733,#5728,#1720,.T.);
#7471=EDGE_CURVE('',#5734,#5735,#3843,.T.);
#7472=EDGE_CURVE('',#5734,#5736,#3844,.T.);
#7473=EDGE_CURVE('',#5737,#5736,#3845,.T.);
#7474=EDGE_CURVE('',#5735,#5737,#3846,.T.);
#7475=EDGE_CURVE('',#5735,#5738,#1721,.T.);
#7476=EDGE_CURVE('',#5737,#5738,#3847,.T.);
#7477=EDGE_CURVE('',#5738,#5739,#3848,.T.);
#7478=EDGE_CURVE('',#5736,#5739,#3849,.T.);
#7479=EDGE_CURVE('',#5739,#5734,#1722,.T.);
#7480=EDGE_CURVE('',#5740,#5741,#3850,.T.);
#7481=EDGE_CURVE('',#5740,#5742,#3851,.T.);
#7482=EDGE_CURVE('',#5743,#5742,#3852,.T.);
#7483=EDGE_CURVE('',#5741,#5743,#3853,.T.);
#7484=EDGE_CURVE('',#5741,#5744,#1723,.T.);
#7485=EDGE_CURVE('',#5743,#5744,#3854,.T.);
#7486=EDGE_CURVE('',#5744,#5745,#3855,.T.);
#7487=EDGE_CURVE('',#5742,#5745,#3856,.T.);
#7488=EDGE_CURVE('',#5745,#5740,#1724,.T.);
#7489=EDGE_CURVE('',#5746,#5747,#3857,.T.);
#7490=EDGE_CURVE('',#5746,#5748,#3858,.T.);
#7491=EDGE_CURVE('',#5749,#5748,#3859,.T.);
#7492=EDGE_CURVE('',#5747,#5749,#3860,.T.);
#7493=EDGE_CURVE('',#5747,#5750,#1725,.T.);
#7494=EDGE_CURVE('',#5749,#5750,#3861,.T.);
#7495=EDGE_CURVE('',#5750,#5751,#3862,.T.);
#7496=EDGE_CURVE('',#5748,#5751,#3863,.T.);
#7497=EDGE_CURVE('',#5751,#5746,#1726,.T.);
#7498=EDGE_CURVE('',#5752,#5753,#3864,.T.);
#7499=EDGE_CURVE('',#5752,#5754,#3865,.T.);
#7500=EDGE_CURVE('',#5755,#5754,#3866,.T.);
#7501=EDGE_CURVE('',#5753,#5755,#3867,.T.);
#7502=EDGE_CURVE('',#5753,#5756,#1727,.T.);
#7503=EDGE_CURVE('',#5755,#5756,#3868,.T.);
#7504=EDGE_CURVE('',#5756,#5757,#3869,.T.);
#7505=EDGE_CURVE('',#5754,#5757,#3870,.T.);
#7506=EDGE_CURVE('',#5757,#5752,#1728,.T.);
#7507=EDGE_CURVE('',#5758,#5759,#1729,.T.);
#7508=EDGE_CURVE('',#5758,#5760,#3871,.T.);
#7509=EDGE_CURVE('',#5760,#5759,#3872,.T.);
#7510=EDGE_CURVE('',#5761,#5758,#3873,.T.);
#7511=EDGE_CURVE('',#5761,#5762,#3874,.T.);
#7512=EDGE_CURVE('',#5760,#5762,#3875,.T.);
#7513=EDGE_CURVE('',#5759,#5763,#3876,.T.);
#7514=EDGE_CURVE('',#5762,#5763,#3877,.T.);
#7515=EDGE_CURVE('',#5763,#5761,#1730,.T.);
#7516=EDGE_CURVE('',#5764,#5765,#3878,.T.);
#7517=EDGE_CURVE('',#5764,#5766,#3879,.T.);
#7518=EDGE_CURVE('',#5767,#5766,#3880,.T.);
#7519=EDGE_CURVE('',#5765,#5767,#3881,.T.);
#7520=EDGE_CURVE('',#5765,#5768,#1731,.T.);
#7521=EDGE_CURVE('',#5767,#5768,#3882,.T.);
#7522=EDGE_CURVE('',#5768,#5769,#3883,.T.);
#7523=EDGE_CURVE('',#5766,#5769,#3884,.T.);
#7524=EDGE_CURVE('',#5769,#5764,#1732,.T.);
#7525=EDGE_CURVE('',#5770,#5771,#3885,.T.);
#7526=EDGE_CURVE('',#5770,#5772,#3886,.T.);
#7527=EDGE_CURVE('',#5773,#5772,#3887,.T.);
#7528=EDGE_CURVE('',#5771,#5773,#3888,.T.);
#7529=EDGE_CURVE('',#5771,#5774,#1733,.T.);
#7530=EDGE_CURVE('',#5773,#5774,#3889,.T.);
#7531=EDGE_CURVE('',#5774,#5775,#3890,.T.);
#7532=EDGE_CURVE('',#5772,#5775,#3891,.T.);
#7533=EDGE_CURVE('',#5775,#5770,#1734,.T.);
#7534=EDGE_CURVE('',#5776,#5777,#3892,.T.);
#7535=EDGE_CURVE('',#5776,#5778,#3893,.T.);
#7536=EDGE_CURVE('',#5779,#5778,#3894,.T.);
#7537=EDGE_CURVE('',#5777,#5779,#3895,.T.);
#7538=EDGE_CURVE('',#5777,#5780,#1735,.T.);
#7539=EDGE_CURVE('',#5779,#5780,#3896,.T.);
#7540=EDGE_CURVE('',#5780,#5781,#3897,.T.);
#7541=EDGE_CURVE('',#5778,#5781,#3898,.T.);
#7542=EDGE_CURVE('',#5781,#5776,#1736,.T.);
#7543=EDGE_CURVE('',#5782,#5783,#3899,.T.);
#7544=EDGE_CURVE('',#5782,#5784,#3900,.T.);
#7545=EDGE_CURVE('',#5785,#5784,#3901,.T.);
#7546=EDGE_CURVE('',#5783,#5785,#3902,.T.);
#7547=EDGE_CURVE('',#5783,#5786,#1737,.T.);
#7548=EDGE_CURVE('',#5785,#5786,#3903,.T.);
#7549=EDGE_CURVE('',#5786,#5787,#3904,.T.);
#7550=EDGE_CURVE('',#5784,#5787,#3905,.T.);
#7551=EDGE_CURVE('',#5787,#5782,#1738,.T.);
#7552=EDGE_CURVE('',#5788,#5789,#3906,.T.);
#7553=EDGE_CURVE('',#5788,#5790,#3907,.T.);
#7554=EDGE_CURVE('',#5791,#5790,#3908,.T.);
#7555=EDGE_CURVE('',#5789,#5791,#3909,.T.);
#7556=EDGE_CURVE('',#5789,#5792,#1739,.T.);
#7557=EDGE_CURVE('',#5791,#5792,#3910,.T.);
#7558=EDGE_CURVE('',#5792,#5793,#3911,.T.);
#7559=EDGE_CURVE('',#5790,#5793,#3912,.T.);
#7560=EDGE_CURVE('',#5793,#5788,#1740,.T.);
#7561=EDGE_CURVE('',#5794,#5795,#3913,.T.);
#7562=EDGE_CURVE('',#5794,#5796,#3914,.T.);
#7563=EDGE_CURVE('',#5797,#5796,#3915,.T.);
#7564=EDGE_CURVE('',#5795,#5797,#3916,.T.);
#7565=EDGE_CURVE('',#5795,#5798,#1741,.T.);
#7566=EDGE_CURVE('',#5797,#5798,#3917,.T.);
#7567=EDGE_CURVE('',#5798,#5799,#3918,.T.);
#7568=EDGE_CURVE('',#5796,#5799,#3919,.T.);
#7569=EDGE_CURVE('',#5799,#5794,#1742,.T.);
#7570=EDGE_CURVE('',#5800,#5801,#3920,.T.);
#7571=EDGE_CURVE('',#5800,#5802,#3921,.T.);
#7572=EDGE_CURVE('',#5803,#5802,#3922,.T.);
#7573=EDGE_CURVE('',#5801,#5803,#3923,.T.);
#7574=EDGE_CURVE('',#5801,#5804,#1743,.T.);
#7575=EDGE_CURVE('',#5803,#5804,#3924,.T.);
#7576=EDGE_CURVE('',#5804,#5805,#3925,.T.);
#7577=EDGE_CURVE('',#5802,#5805,#3926,.T.);
#7578=EDGE_CURVE('',#5805,#5800,#1744,.T.);
#7579=EDGE_CURVE('',#5806,#5807,#3927,.T.);
#7580=EDGE_CURVE('',#5806,#5808,#3928,.T.);
#7581=EDGE_CURVE('',#5809,#5808,#3929,.T.);
#7582=EDGE_CURVE('',#5807,#5809,#3930,.T.);
#7583=EDGE_CURVE('',#5807,#5810,#1745,.T.);
#7584=EDGE_CURVE('',#5809,#5810,#3931,.T.);
#7585=EDGE_CURVE('',#5810,#5811,#3932,.T.);
#7586=EDGE_CURVE('',#5808,#5811,#3933,.T.);
#7587=EDGE_CURVE('',#5811,#5806,#1746,.T.);
#7588=EDGE_CURVE('',#5812,#5813,#3934,.T.);
#7589=EDGE_CURVE('',#5812,#5814,#3935,.T.);
#7590=EDGE_CURVE('',#5815,#5814,#3936,.T.);
#7591=EDGE_CURVE('',#5813,#5815,#3937,.T.);
#7592=EDGE_CURVE('',#5813,#5816,#1747,.T.);
#7593=EDGE_CURVE('',#5815,#5816,#3938,.T.);
#7594=EDGE_CURVE('',#5816,#5817,#3939,.T.);
#7595=EDGE_CURVE('',#5814,#5817,#3940,.T.);
#7596=EDGE_CURVE('',#5817,#5812,#1748,.T.);
#7597=EDGE_CURVE('',#5818,#5818,#1749,.T.);
#7598=EDGE_CURVE('',#5818,#5819,#1750,.T.);
#7599=EDGE_CURVE('',#5819,#5819,#1751,.T.);
#7600=EDGE_CURVE('',#5818,#5820,#3941,.T.);
#7601=EDGE_CURVE('',#5820,#5820,#1752,.T.);
#7602=EDGE_CURVE('',#5821,#5821,#1753,.T.);
#7603=EDGE_CURVE('',#5822,#5822,#1754,.T.);
#7604=EDGE_CURVE('',#5583,#5822,#3942,.T.);
#7605=EDGE_CURVE('',#5585,#5581,#1755,.F.);
#7606=EDGE_CURVE('',#5823,#5823,#1756,.T.);
#7607=EDGE_CURVE('',#5823,#5821,#3943,.T.);
#7608=EDGE_CURVE('',#5810,#5601,#1757,.T.);
#7609=EDGE_CURVE('',#5610,#5807,#1758,.T.);
#7610=EDGE_CURVE('',#5804,#5607,#1759,.T.);
#7611=EDGE_CURVE('',#5616,#5801,#1760,.T.);
#7612=EDGE_CURVE('',#5798,#5613,#1761,.T.);
#7613=EDGE_CURVE('',#5622,#5795,#1762,.T.);
#7614=EDGE_CURVE('',#5792,#5619,#1763,.T.);
#7615=EDGE_CURVE('',#5628,#5789,#1764,.T.);
#7616=EDGE_CURVE('',#5786,#5625,#1765,.T.);
#7617=EDGE_CURVE('',#5634,#5783,#1766,.T.);
#7618=EDGE_CURVE('',#5780,#5631,#1767,.T.);
#7619=EDGE_CURVE('',#5640,#5777,#1768,.T.);
#7620=EDGE_CURVE('',#5774,#5637,#1769,.T.);
#7621=EDGE_CURVE('',#5646,#5771,#1770,.T.);
#7622=EDGE_CURVE('',#5768,#5643,#1771,.T.);
#7623=EDGE_CURVE('',#5653,#5765,#1772,.T.);
#7624=EDGE_CURVE('',#5655,#5823,#3944,.T.);
#7625=EDGE_CURVE('',#5660,#5649,#1773,.T.);
#7626=EDGE_CURVE('',#5756,#5657,#1774,.T.);
#7627=EDGE_CURVE('',#5666,#5753,#1775,.T.);
#7628=EDGE_CURVE('',#5750,#5663,#1776,.T.);
#7629=EDGE_CURVE('',#5672,#5747,#1777,.T.);
#7630=EDGE_CURVE('',#5744,#5669,#1778,.T.);
#7631=EDGE_CURVE('',#5678,#5741,#1779,.T.);
#7632=EDGE_CURVE('',#5738,#5675,#1780,.T.);
#7633=EDGE_CURVE('',#5684,#5735,#1781,.T.);
#7634=EDGE_CURVE('',#5732,#5681,#1782,.T.);
#7635=EDGE_CURVE('',#5690,#5729,#1783,.T.);
#7636=EDGE_CURVE('',#5726,#5687,#1784,.T.);
#7637=EDGE_CURVE('',#5696,#5723,#1785,.T.);
#7638=EDGE_CURVE('',#5720,#5693,#1786,.T.);
#7639=EDGE_CURVE('',#5702,#5717,#1787,.T.);
#7640=EDGE_CURVE('',#5714,#5699,#1788,.T.);
#7641=EDGE_CURVE('',#5708,#5711,#1789,.T.);
#7642=EDGE_CURVE('',#5759,#5705,#1790,.T.);
#7643=EDGE_CURVE('',#5816,#5758,#1791,.T.);
#7644=EDGE_CURVE('',#5604,#5813,#1792,.T.);
#7645=EDGE_CURVE('',#5824,#5824,#1793,.T.);
#7646=EDGE_CURVE('',#5824,#5652,#3945,.T.);
#10165=ORIENTED_EDGE('',*,*,#7094,.F.);
#10166=ORIENTED_EDGE('',*,*,#7095,.T.);
#10167=ORIENTED_EDGE('',*,*,#7096,.T.);
#10168=ORIENTED_EDGE('',*,*,#7097,.T.);
#10169=ORIENTED_EDGE('',*,*,#7098,.F.);
#10170=ORIENTED_EDGE('',*,*,#7099,.T.);
#10171=ORIENTED_EDGE('',*,*,#7094,.T.);
#10172=ORIENTED_EDGE('',*,*,#7100,.T.);
#10173=ORIENTED_EDGE('',*,*,#7101,.F.);
#10174=ORIENTED_EDGE('',*,*,#7102,.T.);
#10175=ORIENTED_EDGE('',*,*,#7098,.T.);
#10176=ORIENTED_EDGE('',*,*,#7103,.T.);
#10177=ORIENTED_EDGE('',*,*,#7104,.F.);
#10178=ORIENTED_EDGE('',*,*,#7105,.T.);
#10179=ORIENTED_EDGE('',*,*,#7101,.T.);
#10180=ORIENTED_EDGE('',*,*,#7106,.T.);
#10181=ORIENTED_EDGE('',*,*,#7107,.F.);
#10182=ORIENTED_EDGE('',*,*,#7108,.T.);
#10183=ORIENTED_EDGE('',*,*,#7104,.T.);
#10184=ORIENTED_EDGE('',*,*,#7109,.T.);
#10185=ORIENTED_EDGE('',*,*,#7110,.F.);
#10186=ORIENTED_EDGE('',*,*,#7111,.T.);
#10187=ORIENTED_EDGE('',*,*,#7107,.T.);
#10188=ORIENTED_EDGE('',*,*,#7112,.T.);
#10189=ORIENTED_EDGE('',*,*,#7113,.F.);
#10190=ORIENTED_EDGE('',*,*,#7114,.T.);
#10191=ORIENTED_EDGE('',*,*,#7110,.T.);
#10192=ORIENTED_EDGE('',*,*,#7115,.T.);
#10193=ORIENTED_EDGE('',*,*,#7116,.F.);
#10194=ORIENTED_EDGE('',*,*,#7117,.T.);
#10195=ORIENTED_EDGE('',*,*,#7113,.T.);
#10196=ORIENTED_EDGE('',*,*,#7118,.T.);
#10197=ORIENTED_EDGE('',*,*,#7119,.F.);
#10198=ORIENTED_EDGE('',*,*,#7120,.T.);
#10199=ORIENTED_EDGE('',*,*,#7116,.T.);
#10200=ORIENTED_EDGE('',*,*,#7121,.T.);
#10201=ORIENTED_EDGE('',*,*,#7122,.F.);
#10202=ORIENTED_EDGE('',*,*,#7123,.T.);
#10203=ORIENTED_EDGE('',*,*,#7119,.T.);
#10204=ORIENTED_EDGE('',*,*,#7124,.T.);
#10205=ORIENTED_EDGE('',*,*,#7125,.F.);
#10206=ORIENTED_EDGE('',*,*,#7126,.T.);
#10207=ORIENTED_EDGE('',*,*,#7122,.T.);
#10208=ORIENTED_EDGE('',*,*,#7127,.T.);
#10209=ORIENTED_EDGE('',*,*,#7128,.F.);
#10210=ORIENTED_EDGE('',*,*,#7129,.T.);
#10211=ORIENTED_EDGE('',*,*,#7125,.T.);
#10212=ORIENTED_EDGE('',*,*,#7130,.T.);
#10213=ORIENTED_EDGE('',*,*,#7131,.F.);
#10214=ORIENTED_EDGE('',*,*,#7132,.T.);
#10215=ORIENTED_EDGE('',*,*,#7128,.T.);
#10216=ORIENTED_EDGE('',*,*,#7133,.T.);
#10217=ORIENTED_EDGE('',*,*,#7134,.F.);
#10218=ORIENTED_EDGE('',*,*,#7135,.T.);
#10219=ORIENTED_EDGE('',*,*,#7131,.T.);
#10220=ORIENTED_EDGE('',*,*,#7136,.T.);
#10221=ORIENTED_EDGE('',*,*,#7137,.F.);
#10222=ORIENTED_EDGE('',*,*,#7138,.T.);
#10223=ORIENTED_EDGE('',*,*,#7134,.T.);
#10224=ORIENTED_EDGE('',*,*,#7139,.T.);
#10225=ORIENTED_EDGE('',*,*,#7140,.F.);
#10226=ORIENTED_EDGE('',*,*,#7141,.T.);
#10227=ORIENTED_EDGE('',*,*,#7137,.T.);
#10228=ORIENTED_EDGE('',*,*,#7142,.T.);
#10229=ORIENTED_EDGE('',*,*,#7143,.F.);
#10230=ORIENTED_EDGE('',*,*,#7144,.T.);
#10231=ORIENTED_EDGE('',*,*,#7140,.T.);
#10232=ORIENTED_EDGE('',*,*,#7145,.T.);
#10233=ORIENTED_EDGE('',*,*,#7146,.F.);
#10234=ORIENTED_EDGE('',*,*,#7147,.T.);
#10235=ORIENTED_EDGE('',*,*,#7143,.T.);
#10236=ORIENTED_EDGE('',*,*,#7148,.T.);
#10237=ORIENTED_EDGE('',*,*,#7149,.F.);
#10238=ORIENTED_EDGE('',*,*,#7150,.T.);
#10239=ORIENTED_EDGE('',*,*,#7146,.T.);
#10240=ORIENTED_EDGE('',*,*,#7151,.T.);
#10241=ORIENTED_EDGE('',*,*,#7152,.F.);
#10242=ORIENTED_EDGE('',*,*,#7153,.T.);
#10243=ORIENTED_EDGE('',*,*,#7149,.T.);
#10244=ORIENTED_EDGE('',*,*,#7154,.T.);
#10245=ORIENTED_EDGE('',*,*,#7155,.F.);
#10246=ORIENTED_EDGE('',*,*,#7156,.T.);
#10247=ORIENTED_EDGE('',*,*,#7152,.T.);
#10248=ORIENTED_EDGE('',*,*,#7157,.T.);
#10249=ORIENTED_EDGE('',*,*,#7158,.F.);
#10250=ORIENTED_EDGE('',*,*,#7159,.T.);
#10251=ORIENTED_EDGE('',*,*,#7155,.T.);
#10252=ORIENTED_EDGE('',*,*,#7160,.T.);
#10253=ORIENTED_EDGE('',*,*,#7161,.F.);
#10254=ORIENTED_EDGE('',*,*,#7162,.T.);
#10255=ORIENTED_EDGE('',*,*,#7158,.T.);
#10256=ORIENTED_EDGE('',*,*,#7163,.T.);
#10257=ORIENTED_EDGE('',*,*,#7164,.F.);
#10258=ORIENTED_EDGE('',*,*,#7165,.T.);
#10259=ORIENTED_EDGE('',*,*,#7161,.T.);
#10260=ORIENTED_EDGE('',*,*,#7166,.T.);
#10261=ORIENTED_EDGE('',*,*,#7167,.F.);
#10262=ORIENTED_EDGE('',*,*,#7168,.T.);
#10263=ORIENTED_EDGE('',*,*,#7169,.F.);
#10264=ORIENTED_EDGE('',*,*,#7170,.F.);
#10265=ORIENTED_EDGE('',*,*,#7171,.T.);
#10266=ORIENTED_EDGE('',*,*,#7167,.T.);
#10267=ORIENTED_EDGE('',*,*,#7172,.F.);
#10268=ORIENTED_EDGE('',*,*,#7173,.F.);
#10269=ORIENTED_EDGE('',*,*,#7174,.F.);
#10270=ORIENTED_EDGE('',*,*,#7175,.T.);
#10271=ORIENTED_EDGE('',*,*,#7170,.T.);
#10272=ORIENTED_EDGE('',*,*,#7176,.F.);
#10273=ORIENTED_EDGE('',*,*,#7177,.F.);
#10274=ORIENTED_EDGE('',*,*,#7178,.T.);
#10275=ORIENTED_EDGE('',*,*,#7174,.T.);
#10276=ORIENTED_EDGE('',*,*,#7179,.F.);
#10277=ORIENTED_EDGE('',*,*,#7180,.F.);
#10278=ORIENTED_EDGE('',*,*,#7181,.T.);
#10279=ORIENTED_EDGE('',*,*,#7177,.T.);
#10280=ORIENTED_EDGE('',*,*,#7182,.F.);
#10281=ORIENTED_EDGE('',*,*,#7183,.F.);
#10282=ORIENTED_EDGE('',*,*,#7184,.T.);
#10283=ORIENTED_EDGE('',*,*,#7180,.T.);
#10284=ORIENTED_EDGE('',*,*,#7185,.F.);
#10285=ORIENTED_EDGE('',*,*,#7186,.F.);
#10286=ORIENTED_EDGE('',*,*,#7187,.T.);
#10287=ORIENTED_EDGE('',*,*,#7183,.T.);
#10288=ORIENTED_EDGE('',*,*,#7188,.F.);
#10289=ORIENTED_EDGE('',*,*,#7189,.F.);
#10290=ORIENTED_EDGE('',*,*,#7190,.T.);
#10291=ORIENTED_EDGE('',*,*,#7186,.T.);
#10292=ORIENTED_EDGE('',*,*,#7191,.F.);
#10293=ORIENTED_EDGE('',*,*,#7192,.F.);
#10294=ORIENTED_EDGE('',*,*,#7193,.T.);
#10295=ORIENTED_EDGE('',*,*,#7189,.T.);
#10296=ORIENTED_EDGE('',*,*,#7194,.F.);
#10297=ORIENTED_EDGE('',*,*,#7195,.F.);
#10298=ORIENTED_EDGE('',*,*,#7196,.T.);
#10299=ORIENTED_EDGE('',*,*,#7192,.T.);
#10300=ORIENTED_EDGE('',*,*,#7197,.F.);
#10301=ORIENTED_EDGE('',*,*,#7198,.F.);
#10302=ORIENTED_EDGE('',*,*,#7199,.T.);
#10303=ORIENTED_EDGE('',*,*,#7195,.T.);
#10304=ORIENTED_EDGE('',*,*,#7200,.F.);
#10305=ORIENTED_EDGE('',*,*,#7201,.F.);
#10306=ORIENTED_EDGE('',*,*,#7202,.T.);
#10307=ORIENTED_EDGE('',*,*,#7198,.T.);
#10308=ORIENTED_EDGE('',*,*,#7203,.F.);
#10309=ORIENTED_EDGE('',*,*,#7204,.F.);
#10310=ORIENTED_EDGE('',*,*,#7205,.T.);
#10311=ORIENTED_EDGE('',*,*,#7201,.T.);
#10312=ORIENTED_EDGE('',*,*,#7206,.F.);
#10313=ORIENTED_EDGE('',*,*,#7207,.F.);
#10314=ORIENTED_EDGE('',*,*,#7208,.T.);
#10315=ORIENTED_EDGE('',*,*,#7204,.T.);
#10316=ORIENTED_EDGE('',*,*,#7209,.F.);
#10317=ORIENTED_EDGE('',*,*,#7210,.F.);
#10318=ORIENTED_EDGE('',*,*,#7211,.T.);
#10319=ORIENTED_EDGE('',*,*,#7207,.T.);
#10320=ORIENTED_EDGE('',*,*,#7212,.F.);
#10321=ORIENTED_EDGE('',*,*,#7213,.F.);
#10322=ORIENTED_EDGE('',*,*,#7214,.T.);
#10323=ORIENTED_EDGE('',*,*,#7210,.T.);
#10324=ORIENTED_EDGE('',*,*,#7215,.F.);
#10325=ORIENTED_EDGE('',*,*,#7216,.F.);
#10326=ORIENTED_EDGE('',*,*,#7217,.T.);
#10327=ORIENTED_EDGE('',*,*,#7213,.T.);
#10328=ORIENTED_EDGE('',*,*,#7218,.F.);
#10329=ORIENTED_EDGE('',*,*,#7219,.F.);
#10330=ORIENTED_EDGE('',*,*,#7220,.T.);
#10331=ORIENTED_EDGE('',*,*,#7216,.T.);
#10332=ORIENTED_EDGE('',*,*,#7221,.F.);
#10333=ORIENTED_EDGE('',*,*,#7222,.F.);
#10334=ORIENTED_EDGE('',*,*,#7223,.T.);
#10335=ORIENTED_EDGE('',*,*,#7219,.T.);
#10336=ORIENTED_EDGE('',*,*,#7224,.F.);
#10337=ORIENTED_EDGE('',*,*,#7225,.F.);
#10338=ORIENTED_EDGE('',*,*,#7226,.T.);
#10339=ORIENTED_EDGE('',*,*,#7222,.T.);
#10340=ORIENTED_EDGE('',*,*,#7227,.F.);
#10341=ORIENTED_EDGE('',*,*,#7228,.F.);
#10342=ORIENTED_EDGE('',*,*,#7229,.T.);
#10343=ORIENTED_EDGE('',*,*,#7225,.T.);
#10344=ORIENTED_EDGE('',*,*,#7230,.F.);
#10345=ORIENTED_EDGE('',*,*,#7231,.F.);
#10346=ORIENTED_EDGE('',*,*,#7232,.T.);
#10347=ORIENTED_EDGE('',*,*,#7228,.T.);
#10348=ORIENTED_EDGE('',*,*,#7233,.F.);
#10349=ORIENTED_EDGE('',*,*,#7234,.F.);
#10350=ORIENTED_EDGE('',*,*,#7235,.T.);
#10351=ORIENTED_EDGE('',*,*,#7231,.T.);
#10352=ORIENTED_EDGE('',*,*,#7236,.F.);
#10353=ORIENTED_EDGE('',*,*,#7237,.F.);
#10354=ORIENTED_EDGE('',*,*,#7238,.T.);
#10355=ORIENTED_EDGE('',*,*,#7234,.T.);
#10356=ORIENTED_EDGE('',*,*,#7239,.F.);
#10357=ORIENTED_EDGE('',*,*,#7240,.F.);
#10358=ORIENTED_EDGE('',*,*,#7241,.F.);
#10359=ORIENTED_EDGE('',*,*,#7166,.F.);
#10360=ORIENTED_EDGE('',*,*,#7163,.F.);
#10361=ORIENTED_EDGE('',*,*,#7160,.F.);
#10362=ORIENTED_EDGE('',*,*,#7157,.F.);
#10363=ORIENTED_EDGE('',*,*,#7154,.F.);
#10364=ORIENTED_EDGE('',*,*,#7151,.F.);
#10365=ORIENTED_EDGE('',*,*,#7148,.F.);
#10366=ORIENTED_EDGE('',*,*,#7145,.F.);
#10367=ORIENTED_EDGE('',*,*,#7142,.F.);
#10368=ORIENTED_EDGE('',*,*,#7139,.F.);
#10369=ORIENTED_EDGE('',*,*,#7136,.F.);
#10370=ORIENTED_EDGE('',*,*,#7133,.F.);
#10371=ORIENTED_EDGE('',*,*,#7130,.F.);
#10372=ORIENTED_EDGE('',*,*,#7127,.F.);
#10373=ORIENTED_EDGE('',*,*,#7124,.F.);
#10374=ORIENTED_EDGE('',*,*,#7121,.F.);
#10375=ORIENTED_EDGE('',*,*,#7118,.F.);
#10376=ORIENTED_EDGE('',*,*,#7115,.F.);
#10377=ORIENTED_EDGE('',*,*,#7112,.F.);
#10378=ORIENTED_EDGE('',*,*,#7109,.F.);
#10379=ORIENTED_EDGE('',*,*,#7106,.F.);
#10380=ORIENTED_EDGE('',*,*,#7103,.F.);
#10381=ORIENTED_EDGE('',*,*,#7100,.F.);
#10382=ORIENTED_EDGE('',*,*,#7097,.F.);
#10383=ORIENTED_EDGE('',*,*,#7242,.F.);
#10384=ORIENTED_EDGE('',*,*,#7243,.T.);
#10385=ORIENTED_EDGE('',*,*,#7239,.T.);
#10386=ORIENTED_EDGE('',*,*,#7236,.T.);
#10387=ORIENTED_EDGE('',*,*,#7233,.T.);
#10388=ORIENTED_EDGE('',*,*,#7230,.T.);
#10389=ORIENTED_EDGE('',*,*,#7227,.T.);
#10390=ORIENTED_EDGE('',*,*,#7224,.T.);
#10391=ORIENTED_EDGE('',*,*,#7221,.T.);
#10392=ORIENTED_EDGE('',*,*,#7218,.T.);
#10393=ORIENTED_EDGE('',*,*,#7215,.T.);
#10394=ORIENTED_EDGE('',*,*,#7212,.T.);
#10395=ORIENTED_EDGE('',*,*,#7209,.T.);
#10396=ORIENTED_EDGE('',*,*,#7206,.T.);
#10397=ORIENTED_EDGE('',*,*,#7203,.T.);
#10398=ORIENTED_EDGE('',*,*,#7200,.T.);
#10399=ORIENTED_EDGE('',*,*,#7197,.T.);
#10400=ORIENTED_EDGE('',*,*,#7194,.T.);
#10401=ORIENTED_EDGE('',*,*,#7191,.T.);
#10402=ORIENTED_EDGE('',*,*,#7188,.T.);
#10403=ORIENTED_EDGE('',*,*,#7185,.T.);
#10404=ORIENTED_EDGE('',*,*,#7182,.T.);
#10405=ORIENTED_EDGE('',*,*,#7179,.T.);
#10406=ORIENTED_EDGE('',*,*,#7176,.T.);
#10407=ORIENTED_EDGE('',*,*,#7173,.T.);
#10408=ORIENTED_EDGE('',*,*,#7244,.T.);
#10409=ORIENTED_EDGE('',*,*,#7245,.T.);
#10410=ORIENTED_EDGE('',*,*,#7246,.T.);
#10411=ORIENTED_EDGE('',*,*,#7247,.T.);
#10412=ORIENTED_EDGE('',*,*,#7242,.T.);
#10413=ORIENTED_EDGE('',*,*,#7237,.T.);
#10414=ORIENTED_EDGE('',*,*,#7243,.F.);
#10415=ORIENTED_EDGE('',*,*,#7247,.F.);
#10416=ORIENTED_EDGE('',*,*,#7248,.T.);
#10417=ORIENTED_EDGE('',*,*,#7249,.F.);
#10418=ORIENTED_EDGE('',*,*,#7168,.F.);
#10419=ORIENTED_EDGE('',*,*,#7171,.F.);
#10420=ORIENTED_EDGE('',*,*,#7175,.F.);
#10421=ORIENTED_EDGE('',*,*,#7178,.F.);
#10422=ORIENTED_EDGE('',*,*,#7181,.F.);
#10423=ORIENTED_EDGE('',*,*,#7184,.F.);
#10424=ORIENTED_EDGE('',*,*,#7187,.F.);
#10425=ORIENTED_EDGE('',*,*,#7190,.F.);
#10426=ORIENTED_EDGE('',*,*,#7193,.F.);
#10427=ORIENTED_EDGE('',*,*,#7196,.F.);
#10428=ORIENTED_EDGE('',*,*,#7199,.F.);
#10429=ORIENTED_EDGE('',*,*,#7202,.F.);
#10430=ORIENTED_EDGE('',*,*,#7205,.F.);
#10431=ORIENTED_EDGE('',*,*,#7208,.F.);
#10432=ORIENTED_EDGE('',*,*,#7211,.F.);
#10433=ORIENTED_EDGE('',*,*,#7214,.F.);
#10434=ORIENTED_EDGE('',*,*,#7217,.F.);
#10435=ORIENTED_EDGE('',*,*,#7220,.F.);
#10436=ORIENTED_EDGE('',*,*,#7223,.F.);
#10437=ORIENTED_EDGE('',*,*,#7226,.F.);
#10438=ORIENTED_EDGE('',*,*,#7229,.F.);
#10439=ORIENTED_EDGE('',*,*,#7232,.F.);
#10440=ORIENTED_EDGE('',*,*,#7235,.F.);
#10441=ORIENTED_EDGE('',*,*,#7238,.F.);
#10442=ORIENTED_EDGE('',*,*,#7248,.F.);
#10443=ORIENTED_EDGE('',*,*,#7246,.F.);
#10444=ORIENTED_EDGE('',*,*,#7095,.F.);
#10445=ORIENTED_EDGE('',*,*,#7099,.F.);
#10446=ORIENTED_EDGE('',*,*,#7102,.F.);
#10447=ORIENTED_EDGE('',*,*,#7105,.F.);
#10448=ORIENTED_EDGE('',*,*,#7108,.F.);
#10449=ORIENTED_EDGE('',*,*,#7111,.F.);
#10450=ORIENTED_EDGE('',*,*,#7114,.F.);
#10451=ORIENTED_EDGE('',*,*,#7117,.F.);
#10452=ORIENTED_EDGE('',*,*,#7120,.F.);
#10453=ORIENTED_EDGE('',*,*,#7123,.F.);
#10454=ORIENTED_EDGE('',*,*,#7126,.F.);
#10455=ORIENTED_EDGE('',*,*,#7129,.F.);
#10456=ORIENTED_EDGE('',*,*,#7132,.F.);
#10457=ORIENTED_EDGE('',*,*,#7135,.F.);
#10458=ORIENTED_EDGE('',*,*,#7138,.F.);
#10459=ORIENTED_EDGE('',*,*,#7141,.F.);
#10460=ORIENTED_EDGE('',*,*,#7144,.F.);
#10461=ORIENTED_EDGE('',*,*,#7147,.F.);
#10462=ORIENTED_EDGE('',*,*,#7150,.F.);
#10463=ORIENTED_EDGE('',*,*,#7153,.F.);
#10464=ORIENTED_EDGE('',*,*,#7156,.F.);
#10465=ORIENTED_EDGE('',*,*,#7159,.F.);
#10466=ORIENTED_EDGE('',*,*,#7162,.F.);
#10467=ORIENTED_EDGE('',*,*,#7165,.F.);
#10468=ORIENTED_EDGE('',*,*,#7250,.F.);
#10469=ORIENTED_EDGE('',*,*,#7251,.T.);
#10470=ORIENTED_EDGE('',*,*,#7252,.F.);
#10471=ORIENTED_EDGE('',*,*,#7251,.F.);
#10472=ORIENTED_EDGE('',*,*,#7253,.F.);
#10473=ORIENTED_EDGE('',*,*,#7254,.T.);
#10474=ORIENTED_EDGE('',*,*,#7255,.T.);
#10475=ORIENTED_EDGE('',*,*,#7256,.F.);
#10476=ORIENTED_EDGE('',*,*,#7257,.F.);
#10477=ORIENTED_EDGE('',*,*,#7258,.T.);
#10478=ORIENTED_EDGE('',*,*,#7259,.T.);
#10479=ORIENTED_EDGE('',*,*,#7254,.F.);
#10480=ORIENTED_EDGE('',*,*,#7260,.F.);
#10481=ORIENTED_EDGE('',*,*,#7261,.T.);
#10482=ORIENTED_EDGE('',*,*,#7262,.T.);
#10483=ORIENTED_EDGE('',*,*,#7258,.F.);
#10484=ORIENTED_EDGE('',*,*,#7263,.F.);
#10485=ORIENTED_EDGE('',*,*,#7264,.T.);
#10486=ORIENTED_EDGE('',*,*,#7265,.T.);
#10487=ORIENTED_EDGE('',*,*,#7261,.F.);
#10488=ORIENTED_EDGE('',*,*,#7266,.F.);
#10489=ORIENTED_EDGE('',*,*,#7267,.T.);
#10490=ORIENTED_EDGE('',*,*,#7268,.T.);
#10491=ORIENTED_EDGE('',*,*,#7264,.F.);
#10492=ORIENTED_EDGE('',*,*,#7269,.F.);
#10493=ORIENTED_EDGE('',*,*,#7256,.T.);
#10494=ORIENTED_EDGE('',*,*,#7270,.T.);
#10495=ORIENTED_EDGE('',*,*,#7267,.F.);
#10496=ORIENTED_EDGE('',*,*,#7270,.F.);
#10497=ORIENTED_EDGE('',*,*,#7255,.F.);
#10498=ORIENTED_EDGE('',*,*,#7259,.F.);
#10499=ORIENTED_EDGE('',*,*,#7262,.F.);
#10500=ORIENTED_EDGE('',*,*,#7265,.F.);
#10501=ORIENTED_EDGE('',*,*,#7268,.F.);
#10502=ORIENTED_EDGE('',*,*,#7252,.T.);
#10503=ORIENTED_EDGE('',*,*,#7271,.F.);
#10504=ORIENTED_EDGE('',*,*,#7272,.T.);
#10505=ORIENTED_EDGE('',*,*,#7273,.F.);
#10506=ORIENTED_EDGE('',*,*,#7274,.F.);
#10507=ORIENTED_EDGE('',*,*,#7275,.F.);
#10508=ORIENTED_EDGE('',*,*,#7274,.T.);
#10509=ORIENTED_EDGE('',*,*,#7276,.T.);
#10510=ORIENTED_EDGE('',*,*,#7277,.F.);
#10511=ORIENTED_EDGE('',*,*,#7276,.F.);
#10512=ORIENTED_EDGE('',*,*,#7273,.T.);
#10513=ORIENTED_EDGE('',*,*,#7278,.T.);
#10514=ORIENTED_EDGE('',*,*,#7279,.F.);
#10515=ORIENTED_EDGE('',*,*,#7278,.F.);
#10516=ORIENTED_EDGE('',*,*,#7272,.F.);
#10517=ORIENTED_EDGE('',*,*,#7280,.F.);
#10518=ORIENTED_EDGE('',*,*,#7281,.T.);
#10519=ORIENTED_EDGE('',*,*,#7282,.F.);
#10520=ORIENTED_EDGE('',*,*,#7283,.F.);
#10521=ORIENTED_EDGE('',*,*,#7284,.F.);
#10522=ORIENTED_EDGE('',*,*,#7283,.T.);
#10523=ORIENTED_EDGE('',*,*,#7285,.T.);
#10524=ORIENTED_EDGE('',*,*,#7286,.F.);
#10525=ORIENTED_EDGE('',*,*,#7285,.F.);
#10526=ORIENTED_EDGE('',*,*,#7282,.T.);
#10527=ORIENTED_EDGE('',*,*,#7287,.T.);
#10528=ORIENTED_EDGE('',*,*,#7288,.F.);
#10529=ORIENTED_EDGE('',*,*,#7287,.F.);
#10530=ORIENTED_EDGE('',*,*,#7281,.F.);
#10531=ORIENTED_EDGE('',*,*,#7289,.F.);
#10532=ORIENTED_EDGE('',*,*,#7290,.T.);
#10533=ORIENTED_EDGE('',*,*,#7291,.F.);
#10534=ORIENTED_EDGE('',*,*,#7292,.F.);
#10535=ORIENTED_EDGE('',*,*,#7293,.F.);
#10536=ORIENTED_EDGE('',*,*,#7292,.T.);
#10537=ORIENTED_EDGE('',*,*,#7294,.T.);
#10538=ORIENTED_EDGE('',*,*,#7295,.F.);
#10539=ORIENTED_EDGE('',*,*,#7294,.F.);
#10540=ORIENTED_EDGE('',*,*,#7291,.T.);
#10541=ORIENTED_EDGE('',*,*,#7296,.T.);
#10542=ORIENTED_EDGE('',*,*,#7297,.F.);
#10543=ORIENTED_EDGE('',*,*,#7296,.F.);
#10544=ORIENTED_EDGE('',*,*,#7290,.F.);
#10545=ORIENTED_EDGE('',*,*,#7298,.F.);
#10546=ORIENTED_EDGE('',*,*,#7299,.T.);
#10547=ORIENTED_EDGE('',*,*,#7300,.F.);
#10548=ORIENTED_EDGE('',*,*,#7301,.F.);
#10549=ORIENTED_EDGE('',*,*,#7302,.F.);
#10550=ORIENTED_EDGE('',*,*,#7301,.T.);
#10551=ORIENTED_EDGE('',*,*,#7303,.T.);
#10552=ORIENTED_EDGE('',*,*,#7304,.F.);
#10553=ORIENTED_EDGE('',*,*,#7303,.F.);
#10554=ORIENTED_EDGE('',*,*,#7300,.T.);
#10555=ORIENTED_EDGE('',*,*,#7305,.T.);
#10556=ORIENTED_EDGE('',*,*,#7306,.F.);
#10557=ORIENTED_EDGE('',*,*,#7305,.F.);
#10558=ORIENTED_EDGE('',*,*,#7299,.F.);
#10559=ORIENTED_EDGE('',*,*,#7307,.F.);
#10560=ORIENTED_EDGE('',*,*,#7308,.T.);
#10561=ORIENTED_EDGE('',*,*,#7309,.F.);
#10562=ORIENTED_EDGE('',*,*,#7310,.F.);
#10563=ORIENTED_EDGE('',*,*,#7311,.F.);
#10564=ORIENTED_EDGE('',*,*,#7310,.T.);
#10565=ORIENTED_EDGE('',*,*,#7312,.T.);
#10566=ORIENTED_EDGE('',*,*,#7313,.F.);
#10567=ORIENTED_EDGE('',*,*,#7312,.F.);
#10568=ORIENTED_EDGE('',*,*,#7309,.T.);
#10569=ORIENTED_EDGE('',*,*,#7314,.T.);
#10570=ORIENTED_EDGE('',*,*,#7315,.F.);
#10571=ORIENTED_EDGE('',*,*,#7314,.F.);
#10572=ORIENTED_EDGE('',*,*,#7308,.F.);
#10573=ORIENTED_EDGE('',*,*,#7316,.F.);
#10574=ORIENTED_EDGE('',*,*,#7317,.T.);
#10575=ORIENTED_EDGE('',*,*,#7318,.F.);
#10576=ORIENTED_EDGE('',*,*,#7319,.F.);
#10577=ORIENTED_EDGE('',*,*,#7320,.F.);
#10578=ORIENTED_EDGE('',*,*,#7319,.T.);
#10579=ORIENTED_EDGE('',*,*,#7321,.T.);
#10580=ORIENTED_EDGE('',*,*,#7322,.F.);
#10581=ORIENTED_EDGE('',*,*,#7321,.F.);
#10582=ORIENTED_EDGE('',*,*,#7318,.T.);
#10583=ORIENTED_EDGE('',*,*,#7323,.T.);
#10584=ORIENTED_EDGE('',*,*,#7324,.F.);
#10585=ORIENTED_EDGE('',*,*,#7323,.F.);
#10586=ORIENTED_EDGE('',*,*,#7317,.F.);
#10587=ORIENTED_EDGE('',*,*,#7325,.F.);
#10588=ORIENTED_EDGE('',*,*,#7326,.T.);
#10589=ORIENTED_EDGE('',*,*,#7327,.F.);
#10590=ORIENTED_EDGE('',*,*,#7328,.F.);
#10591=ORIENTED_EDGE('',*,*,#7329,.F.);
#10592=ORIENTED_EDGE('',*,*,#7328,.T.);
#10593=ORIENTED_EDGE('',*,*,#7330,.T.);
#10594=ORIENTED_EDGE('',*,*,#7331,.F.);
#10595=ORIENTED_EDGE('',*,*,#7330,.F.);
#10596=ORIENTED_EDGE('',*,*,#7327,.T.);
#10597=ORIENTED_EDGE('',*,*,#7332,.T.);
#10598=ORIENTED_EDGE('',*,*,#7333,.F.);
#10599=ORIENTED_EDGE('',*,*,#7332,.F.);
#10600=ORIENTED_EDGE('',*,*,#7326,.F.);
#10601=ORIENTED_EDGE('',*,*,#7334,.F.);
#10602=ORIENTED_EDGE('',*,*,#7335,.T.);
#10603=ORIENTED_EDGE('',*,*,#7336,.F.);
#10604=ORIENTED_EDGE('',*,*,#7337,.F.);
#10605=ORIENTED_EDGE('',*,*,#7338,.F.);
#10606=ORIENTED_EDGE('',*,*,#7337,.T.);
#10607=ORIENTED_EDGE('',*,*,#7339,.T.);
#10608=ORIENTED_EDGE('',*,*,#7340,.F.);
#10609=ORIENTED_EDGE('',*,*,#7339,.F.);
#10610=ORIENTED_EDGE('',*,*,#7336,.T.);
#10611=ORIENTED_EDGE('',*,*,#7341,.T.);
#10612=ORIENTED_EDGE('',*,*,#7342,.F.);
#10613=ORIENTED_EDGE('',*,*,#7341,.F.);
#10614=ORIENTED_EDGE('',*,*,#7335,.F.);
#10615=ORIENTED_EDGE('',*,*,#7343,.F.);
#10616=ORIENTED_EDGE('',*,*,#7344,.T.);
#10617=ORIENTED_EDGE('',*,*,#7345,.F.);
#10618=ORIENTED_EDGE('',*,*,#7346,.F.);
#10619=ORIENTED_EDGE('',*,*,#7347,.F.);
#10620=ORIENTED_EDGE('',*,*,#7346,.T.);
#10621=ORIENTED_EDGE('',*,*,#7348,.T.);
#10622=ORIENTED_EDGE('',*,*,#7349,.F.);
#10623=ORIENTED_EDGE('',*,*,#7350,.F.);
#10624=ORIENTED_EDGE('',*,*,#7348,.F.);
#10625=ORIENTED_EDGE('',*,*,#7345,.T.);
#10626=ORIENTED_EDGE('',*,*,#7351,.T.);
#10627=ORIENTED_EDGE('',*,*,#7352,.F.);
#10628=ORIENTED_EDGE('',*,*,#7351,.F.);
#10629=ORIENTED_EDGE('',*,*,#7344,.F.);
#10630=ORIENTED_EDGE('',*,*,#7353,.F.);
#10631=ORIENTED_EDGE('',*,*,#7354,.F.);
#10632=ORIENTED_EDGE('',*,*,#7355,.T.);
#10633=ORIENTED_EDGE('',*,*,#7356,.F.);
#10634=ORIENTED_EDGE('',*,*,#7357,.F.);
#10635=ORIENTED_EDGE('',*,*,#7358,.F.);
#10636=ORIENTED_EDGE('',*,*,#7357,.T.);
#10637=ORIENTED_EDGE('',*,*,#7359,.T.);
#10638=ORIENTED_EDGE('',*,*,#7360,.F.);
#10639=ORIENTED_EDGE('',*,*,#7359,.F.);
#10640=ORIENTED_EDGE('',*,*,#7356,.T.);
#10641=ORIENTED_EDGE('',*,*,#7361,.T.);
#10642=ORIENTED_EDGE('',*,*,#7362,.F.);
#10643=ORIENTED_EDGE('',*,*,#7361,.F.);
#10644=ORIENTED_EDGE('',*,*,#7355,.F.);
#10645=ORIENTED_EDGE('',*,*,#7363,.F.);
#10646=ORIENTED_EDGE('',*,*,#7364,.T.);
#10647=ORIENTED_EDGE('',*,*,#7365,.F.);
#10648=ORIENTED_EDGE('',*,*,#7366,.F.);
#10649=ORIENTED_EDGE('',*,*,#7367,.F.);
#10650=ORIENTED_EDGE('',*,*,#7366,.T.);
#10651=ORIENTED_EDGE('',*,*,#7368,.T.);
#10652=ORIENTED_EDGE('',*,*,#7369,.F.);
#10653=ORIENTED_EDGE('',*,*,#7368,.F.);
#10654=ORIENTED_EDGE('',*,*,#7365,.T.);
#10655=ORIENTED_EDGE('',*,*,#7370,.T.);
#10656=ORIENTED_EDGE('',*,*,#7371,.F.);
#10657=ORIENTED_EDGE('',*,*,#7370,.F.);
#10658=ORIENTED_EDGE('',*,*,#7364,.F.);
#10659=ORIENTED_EDGE('',*,*,#7372,.F.);
#10660=ORIENTED_EDGE('',*,*,#7373,.T.);
#10661=ORIENTED_EDGE('',*,*,#7374,.F.);
#10662=ORIENTED_EDGE('',*,*,#7375,.F.);
#10663=ORIENTED_EDGE('',*,*,#7376,.F.);
#10664=ORIENTED_EDGE('',*,*,#7375,.T.);
#10665=ORIENTED_EDGE('',*,*,#7377,.T.);
#10666=ORIENTED_EDGE('',*,*,#7378,.F.);
#10667=ORIENTED_EDGE('',*,*,#7377,.F.);
#10668=ORIENTED_EDGE('',*,*,#7374,.T.);
#10669=ORIENTED_EDGE('',*,*,#7379,.T.);
#10670=ORIENTED_EDGE('',*,*,#7380,.F.);
#10671=ORIENTED_EDGE('',*,*,#7379,.F.);
#10672=ORIENTED_EDGE('',*,*,#7373,.F.);
#10673=ORIENTED_EDGE('',*,*,#7381,.F.);
#10674=ORIENTED_EDGE('',*,*,#7382,.T.);
#10675=ORIENTED_EDGE('',*,*,#7383,.F.);
#10676=ORIENTED_EDGE('',*,*,#7384,.F.);
#10677=ORIENTED_EDGE('',*,*,#7385,.F.);
#10678=ORIENTED_EDGE('',*,*,#7384,.T.);
#10679=ORIENTED_EDGE('',*,*,#7386,.T.);
#10680=ORIENTED_EDGE('',*,*,#7387,.F.);
#10681=ORIENTED_EDGE('',*,*,#7386,.F.);
#10682=ORIENTED_EDGE('',*,*,#7383,.T.);
#10683=ORIENTED_EDGE('',*,*,#7388,.T.);
#10684=ORIENTED_EDGE('',*,*,#7389,.F.);
#10685=ORIENTED_EDGE('',*,*,#7388,.F.);
#10686=ORIENTED_EDGE('',*,*,#7382,.F.);
#10687=ORIENTED_EDGE('',*,*,#7390,.F.);
#10688=ORIENTED_EDGE('',*,*,#7391,.T.);
#10689=ORIENTED_EDGE('',*,*,#7392,.F.);
#10690=ORIENTED_EDGE('',*,*,#7393,.F.);
#10691=ORIENTED_EDGE('',*,*,#7394,.F.);
#10692=ORIENTED_EDGE('',*,*,#7393,.T.);
#10693=ORIENTED_EDGE('',*,*,#7395,.T.);
#10694=ORIENTED_EDGE('',*,*,#7396,.F.);
#10695=ORIENTED_EDGE('',*,*,#7395,.F.);
#10696=ORIENTED_EDGE('',*,*,#7392,.T.);
#10697=ORIENTED_EDGE('',*,*,#7397,.T.);
#10698=ORIENTED_EDGE('',*,*,#7398,.F.);
#10699=ORIENTED_EDGE('',*,*,#7397,.F.);
#10700=ORIENTED_EDGE('',*,*,#7391,.F.);
#10701=ORIENTED_EDGE('',*,*,#7399,.F.);
#10702=ORIENTED_EDGE('',*,*,#7400,.T.);
#10703=ORIENTED_EDGE('',*,*,#7401,.F.);
#10704=ORIENTED_EDGE('',*,*,#7402,.F.);
#10705=ORIENTED_EDGE('',*,*,#7403,.F.);
#10706=ORIENTED_EDGE('',*,*,#7402,.T.);
#10707=ORIENTED_EDGE('',*,*,#7404,.T.);
#10708=ORIENTED_EDGE('',*,*,#7405,.F.);
#10709=ORIENTED_EDGE('',*,*,#7404,.F.);
#10710=ORIENTED_EDGE('',*,*,#7401,.T.);
#10711=ORIENTED_EDGE('',*,*,#7406,.T.);
#10712=ORIENTED_EDGE('',*,*,#7407,.F.);
#10713=ORIENTED_EDGE('',*,*,#7406,.F.);
#10714=ORIENTED_EDGE('',*,*,#7400,.F.);
#10715=ORIENTED_EDGE('',*,*,#7408,.F.);
#10716=ORIENTED_EDGE('',*,*,#7409,.T.);
#10717=ORIENTED_EDGE('',*,*,#7410,.F.);
#10718=ORIENTED_EDGE('',*,*,#7411,.F.);
#10719=ORIENTED_EDGE('',*,*,#7412,.F.);
#10720=ORIENTED_EDGE('',*,*,#7411,.T.);
#10721=ORIENTED_EDGE('',*,*,#7413,.T.);
#10722=ORIENTED_EDGE('',*,*,#7414,.F.);
#10723=ORIENTED_EDGE('',*,*,#7413,.F.);
#10724=ORIENTED_EDGE('',*,*,#7410,.T.);
#10725=ORIENTED_EDGE('',*,*,#7415,.T.);
#10726=ORIENTED_EDGE('',*,*,#7416,.F.);
#10727=ORIENTED_EDGE('',*,*,#7415,.F.);
#10728=ORIENTED_EDGE('',*,*,#7409,.F.);
#10729=ORIENTED_EDGE('',*,*,#7417,.F.);
#10730=ORIENTED_EDGE('',*,*,#7418,.T.);
#10731=ORIENTED_EDGE('',*,*,#7419,.F.);
#10732=ORIENTED_EDGE('',*,*,#7420,.F.);
#10733=ORIENTED_EDGE('',*,*,#7421,.F.);
#10734=ORIENTED_EDGE('',*,*,#7420,.T.);
#10735=ORIENTED_EDGE('',*,*,#7422,.T.);
#10736=ORIENTED_EDGE('',*,*,#7423,.F.);
#10737=ORIENTED_EDGE('',*,*,#7422,.F.);
#10738=ORIENTED_EDGE('',*,*,#7419,.T.);
#10739=ORIENTED_EDGE('',*,*,#7424,.T.);
#10740=ORIENTED_EDGE('',*,*,#7425,.F.);
#10741=ORIENTED_EDGE('',*,*,#7424,.F.);
#10742=ORIENTED_EDGE('',*,*,#7418,.F.);
#10743=ORIENTED_EDGE('',*,*,#7426,.F.);
#10744=ORIENTED_EDGE('',*,*,#7427,.T.);
#10745=ORIENTED_EDGE('',*,*,#7428,.F.);
#10746=ORIENTED_EDGE('',*,*,#7429,.F.);
#10747=ORIENTED_EDGE('',*,*,#7430,.F.);
#10748=ORIENTED_EDGE('',*,*,#7429,.T.);
#10749=ORIENTED_EDGE('',*,*,#7431,.T.);
#10750=ORIENTED_EDGE('',*,*,#7432,.F.);
#10751=ORIENTED_EDGE('',*,*,#7431,.F.);
#10752=ORIENTED_EDGE('',*,*,#7428,.T.);
#10753=ORIENTED_EDGE('',*,*,#7433,.T.);
#10754=ORIENTED_EDGE('',*,*,#7434,.F.);
#10755=ORIENTED_EDGE('',*,*,#7433,.F.);
#10756=ORIENTED_EDGE('',*,*,#7427,.F.);
#10757=ORIENTED_EDGE('',*,*,#7435,.F.);
#10758=ORIENTED_EDGE('',*,*,#7436,.T.);
#10759=ORIENTED_EDGE('',*,*,#7437,.F.);
#10760=ORIENTED_EDGE('',*,*,#7438,.F.);
#10761=ORIENTED_EDGE('',*,*,#7439,.F.);
#10762=ORIENTED_EDGE('',*,*,#7438,.T.);
#10763=ORIENTED_EDGE('',*,*,#7440,.T.);
#10764=ORIENTED_EDGE('',*,*,#7441,.F.);
#10765=ORIENTED_EDGE('',*,*,#7440,.F.);
#10766=ORIENTED_EDGE('',*,*,#7437,.T.);
#10767=ORIENTED_EDGE('',*,*,#7442,.T.);
#10768=ORIENTED_EDGE('',*,*,#7443,.F.);
#10769=ORIENTED_EDGE('',*,*,#7442,.F.);
#10770=ORIENTED_EDGE('',*,*,#7436,.F.);
#10771=ORIENTED_EDGE('',*,*,#7444,.F.);
#10772=ORIENTED_EDGE('',*,*,#7445,.T.);
#10773=ORIENTED_EDGE('',*,*,#7446,.F.);
#10774=ORIENTED_EDGE('',*,*,#7447,.F.);
#10775=ORIENTED_EDGE('',*,*,#7448,.F.);
#10776=ORIENTED_EDGE('',*,*,#7447,.T.);
#10777=ORIENTED_EDGE('',*,*,#7449,.T.);
#10778=ORIENTED_EDGE('',*,*,#7450,.F.);
#10779=ORIENTED_EDGE('',*,*,#7449,.F.);
#10780=ORIENTED_EDGE('',*,*,#7446,.T.);
#10781=ORIENTED_EDGE('',*,*,#7451,.T.);
#10782=ORIENTED_EDGE('',*,*,#7452,.F.);
#10783=ORIENTED_EDGE('',*,*,#7451,.F.);
#10784=ORIENTED_EDGE('',*,*,#7445,.F.);
#10785=ORIENTED_EDGE('',*,*,#7453,.F.);
#10786=ORIENTED_EDGE('',*,*,#7454,.T.);
#10787=ORIENTED_EDGE('',*,*,#7455,.F.);
#10788=ORIENTED_EDGE('',*,*,#7456,.F.);
#10789=ORIENTED_EDGE('',*,*,#7457,.F.);
#10790=ORIENTED_EDGE('',*,*,#7456,.T.);
#10791=ORIENTED_EDGE('',*,*,#7458,.T.);
#10792=ORIENTED_EDGE('',*,*,#7459,.F.);
#10793=ORIENTED_EDGE('',*,*,#7458,.F.);
#10794=ORIENTED_EDGE('',*,*,#7455,.T.);
#10795=ORIENTED_EDGE('',*,*,#7460,.T.);
#10796=ORIENTED_EDGE('',*,*,#7461,.F.);
#10797=ORIENTED_EDGE('',*,*,#7460,.F.);
#10798=ORIENTED_EDGE('',*,*,#7454,.F.);
#10799=ORIENTED_EDGE('',*,*,#7462,.F.);
#10800=ORIENTED_EDGE('',*,*,#7463,.T.);
#10801=ORIENTED_EDGE('',*,*,#7464,.F.);
#10802=ORIENTED_EDGE('',*,*,#7465,.F.);
#10803=ORIENTED_EDGE('',*,*,#7466,.F.);
#10804=ORIENTED_EDGE('',*,*,#7465,.T.);
#10805=ORIENTED_EDGE('',*,*,#7467,.T.);
#10806=ORIENTED_EDGE('',*,*,#7468,.F.);
#10807=ORIENTED_EDGE('',*,*,#7467,.F.);
#10808=ORIENTED_EDGE('',*,*,#7464,.T.);
#10809=ORIENTED_EDGE('',*,*,#7469,.T.);
#10810=ORIENTED_EDGE('',*,*,#7470,.F.);
#10811=ORIENTED_EDGE('',*,*,#7469,.F.);
#10812=ORIENTED_EDGE('',*,*,#7463,.F.);
#10813=ORIENTED_EDGE('',*,*,#7471,.F.);
#10814=ORIENTED_EDGE('',*,*,#7472,.T.);
#10815=ORIENTED_EDGE('',*,*,#7473,.F.);
#10816=ORIENTED_EDGE('',*,*,#7474,.F.);
#10817=ORIENTED_EDGE('',*,*,#7475,.F.);
#10818=ORIENTED_EDGE('',*,*,#7474,.T.);
#10819=ORIENTED_EDGE('',*,*,#7476,.T.);
#10820=ORIENTED_EDGE('',*,*,#7477,.F.);
#10821=ORIENTED_EDGE('',*,*,#7476,.F.);
#10822=ORIENTED_EDGE('',*,*,#7473,.T.);
#10823=ORIENTED_EDGE('',*,*,#7478,.T.);
#10824=ORIENTED_EDGE('',*,*,#7479,.F.);
#10825=ORIENTED_EDGE('',*,*,#7478,.F.);
#10826=ORIENTED_EDGE('',*,*,#7472,.F.);
#10827=ORIENTED_EDGE('',*,*,#7480,.F.);
#10828=ORIENTED_EDGE('',*,*,#7481,.T.);
#10829=ORIENTED_EDGE('',*,*,#7482,.F.);
#10830=ORIENTED_EDGE('',*,*,#7483,.F.);
#10831=ORIENTED_EDGE('',*,*,#7484,.F.);
#10832=ORIENTED_EDGE('',*,*,#7483,.T.);
#10833=ORIENTED_EDGE('',*,*,#7485,.T.);
#10834=ORIENTED_EDGE('',*,*,#7486,.F.);
#10835=ORIENTED_EDGE('',*,*,#7485,.F.);
#10836=ORIENTED_EDGE('',*,*,#7482,.T.);
#10837=ORIENTED_EDGE('',*,*,#7487,.T.);
#10838=ORIENTED_EDGE('',*,*,#7488,.F.);
#10839=ORIENTED_EDGE('',*,*,#7487,.F.);
#10840=ORIENTED_EDGE('',*,*,#7481,.F.);
#10841=ORIENTED_EDGE('',*,*,#7489,.F.);
#10842=ORIENTED_EDGE('',*,*,#7490,.T.);
#10843=ORIENTED_EDGE('',*,*,#7491,.F.);
#10844=ORIENTED_EDGE('',*,*,#7492,.F.);
#10845=ORIENTED_EDGE('',*,*,#7493,.F.);
#10846=ORIENTED_EDGE('',*,*,#7492,.T.);
#10847=ORIENTED_EDGE('',*,*,#7494,.T.);
#10848=ORIENTED_EDGE('',*,*,#7495,.F.);
#10849=ORIENTED_EDGE('',*,*,#7494,.F.);
#10850=ORIENTED_EDGE('',*,*,#7491,.T.);
#10851=ORIENTED_EDGE('',*,*,#7496,.T.);
#10852=ORIENTED_EDGE('',*,*,#7497,.F.);
#10853=ORIENTED_EDGE('',*,*,#7496,.F.);
#10854=ORIENTED_EDGE('',*,*,#7490,.F.);
#10855=ORIENTED_EDGE('',*,*,#7498,.F.);
#10856=ORIENTED_EDGE('',*,*,#7499,.T.);
#10857=ORIENTED_EDGE('',*,*,#7500,.F.);
#10858=ORIENTED_EDGE('',*,*,#7501,.F.);
#10859=ORIENTED_EDGE('',*,*,#7502,.F.);
#10860=ORIENTED_EDGE('',*,*,#7501,.T.);
#10861=ORIENTED_EDGE('',*,*,#7503,.T.);
#10862=ORIENTED_EDGE('',*,*,#7504,.F.);
#10863=ORIENTED_EDGE('',*,*,#7503,.F.);
#10864=ORIENTED_EDGE('',*,*,#7500,.T.);
#10865=ORIENTED_EDGE('',*,*,#7505,.T.);
#10866=ORIENTED_EDGE('',*,*,#7506,.F.);
#10867=ORIENTED_EDGE('',*,*,#7505,.F.);
#10868=ORIENTED_EDGE('',*,*,#7499,.F.);
#10869=ORIENTED_EDGE('',*,*,#7507,.F.);
#10870=ORIENTED_EDGE('',*,*,#7508,.T.);
#10871=ORIENTED_EDGE('',*,*,#7509,.T.);
#10872=ORIENTED_EDGE('',*,*,#7510,.F.);
#10873=ORIENTED_EDGE('',*,*,#7511,.T.);
#10874=ORIENTED_EDGE('',*,*,#7512,.F.);
#10875=ORIENTED_EDGE('',*,*,#7508,.F.);
#10876=ORIENTED_EDGE('',*,*,#7513,.F.);
#10877=ORIENTED_EDGE('',*,*,#7509,.F.);
#10878=ORIENTED_EDGE('',*,*,#7512,.T.);
#10879=ORIENTED_EDGE('',*,*,#7514,.T.);
#10880=ORIENTED_EDGE('',*,*,#7515,.F.);
#10881=ORIENTED_EDGE('',*,*,#7514,.F.);
#10882=ORIENTED_EDGE('',*,*,#7511,.F.);
#10883=ORIENTED_EDGE('',*,*,#7516,.F.);
#10884=ORIENTED_EDGE('',*,*,#7517,.T.);
#10885=ORIENTED_EDGE('',*,*,#7518,.F.);
#10886=ORIENTED_EDGE('',*,*,#7519,.F.);
#10887=ORIENTED_EDGE('',*,*,#7520,.F.);
#10888=ORIENTED_EDGE('',*,*,#7519,.T.);
#10889=ORIENTED_EDGE('',*,*,#7521,.T.);
#10890=ORIENTED_EDGE('',*,*,#7522,.F.);
#10891=ORIENTED_EDGE('',*,*,#7521,.F.);
#10892=ORIENTED_EDGE('',*,*,#7518,.T.);
#10893=ORIENTED_EDGE('',*,*,#7523,.T.);
#10894=ORIENTED_EDGE('',*,*,#7524,.F.);
#10895=ORIENTED_EDGE('',*,*,#7523,.F.);
#10896=ORIENTED_EDGE('',*,*,#7517,.F.);
#10897=ORIENTED_EDGE('',*,*,#7525,.F.);
#10898=ORIENTED_EDGE('',*,*,#7526,.T.);
#10899=ORIENTED_EDGE('',*,*,#7527,.F.);
#10900=ORIENTED_EDGE('',*,*,#7528,.F.);
#10901=ORIENTED_EDGE('',*,*,#7529,.F.);
#10902=ORIENTED_EDGE('',*,*,#7528,.T.);
#10903=ORIENTED_EDGE('',*,*,#7530,.T.);
#10904=ORIENTED_EDGE('',*,*,#7531,.F.);
#10905=ORIENTED_EDGE('',*,*,#7530,.F.);
#10906=ORIENTED_EDGE('',*,*,#7527,.T.);
#10907=ORIENTED_EDGE('',*,*,#7532,.T.);
#10908=ORIENTED_EDGE('',*,*,#7533,.F.);
#10909=ORIENTED_EDGE('',*,*,#7532,.F.);
#10910=ORIENTED_EDGE('',*,*,#7526,.F.);
#10911=ORIENTED_EDGE('',*,*,#7534,.F.);
#10912=ORIENTED_EDGE('',*,*,#7535,.T.);
#10913=ORIENTED_EDGE('',*,*,#7536,.F.);
#10914=ORIENTED_EDGE('',*,*,#7537,.F.);
#10915=ORIENTED_EDGE('',*,*,#7538,.F.);
#10916=ORIENTED_EDGE('',*,*,#7537,.T.);
#10917=ORIENTED_EDGE('',*,*,#7539,.T.);
#10918=ORIENTED_EDGE('',*,*,#7540,.F.);
#10919=ORIENTED_EDGE('',*,*,#7539,.F.);
#10920=ORIENTED_EDGE('',*,*,#7536,.T.);
#10921=ORIENTED_EDGE('',*,*,#7541,.T.);
#10922=ORIENTED_EDGE('',*,*,#7542,.F.);
#10923=ORIENTED_EDGE('',*,*,#7541,.F.);
#10924=ORIENTED_EDGE('',*,*,#7535,.F.);
#10925=ORIENTED_EDGE('',*,*,#7543,.F.);
#10926=ORIENTED_EDGE('',*,*,#7544,.T.);
#10927=ORIENTED_EDGE('',*,*,#7545,.F.);
#10928=ORIENTED_EDGE('',*,*,#7546,.F.);
#10929=ORIENTED_EDGE('',*,*,#7547,.F.);
#10930=ORIENTED_EDGE('',*,*,#7546,.T.);
#10931=ORIENTED_EDGE('',*,*,#7548,.T.);
#10932=ORIENTED_EDGE('',*,*,#7549,.F.);
#10933=ORIENTED_EDGE('',*,*,#7548,.F.);
#10934=ORIENTED_EDGE('',*,*,#7545,.T.);
#10935=ORIENTED_EDGE('',*,*,#7550,.T.);
#10936=ORIENTED_EDGE('',*,*,#7551,.F.);
#10937=ORIENTED_EDGE('',*,*,#7550,.F.);
#10938=ORIENTED_EDGE('',*,*,#7544,.F.);
#10939=ORIENTED_EDGE('',*,*,#7552,.F.);
#10940=ORIENTED_EDGE('',*,*,#7553,.T.);
#10941=ORIENTED_EDGE('',*,*,#7554,.F.);
#10942=ORIENTED_EDGE('',*,*,#7555,.F.);
#10943=ORIENTED_EDGE('',*,*,#7556,.F.);
#10944=ORIENTED_EDGE('',*,*,#7555,.T.);
#10945=ORIENTED_EDGE('',*,*,#7557,.T.);
#10946=ORIENTED_EDGE('',*,*,#7558,.F.);
#10947=ORIENTED_EDGE('',*,*,#7557,.F.);
#10948=ORIENTED_EDGE('',*,*,#7554,.T.);
#10949=ORIENTED_EDGE('',*,*,#7559,.T.);
#10950=ORIENTED_EDGE('',*,*,#7560,.F.);
#10951=ORIENTED_EDGE('',*,*,#7559,.F.);
#10952=ORIENTED_EDGE('',*,*,#7553,.F.);
#10953=ORIENTED_EDGE('',*,*,#7561,.F.);
#10954=ORIENTED_EDGE('',*,*,#7562,.T.);
#10955=ORIENTED_EDGE('',*,*,#7563,.F.);
#10956=ORIENTED_EDGE('',*,*,#7564,.F.);
#10957=ORIENTED_EDGE('',*,*,#7565,.F.);
#10958=ORIENTED_EDGE('',*,*,#7564,.T.);
#10959=ORIENTED_EDGE('',*,*,#7566,.T.);
#10960=ORIENTED_EDGE('',*,*,#7567,.F.);
#10961=ORIENTED_EDGE('',*,*,#7566,.F.);
#10962=ORIENTED_EDGE('',*,*,#7563,.T.);
#10963=ORIENTED_EDGE('',*,*,#7568,.T.);
#10964=ORIENTED_EDGE('',*,*,#7569,.F.);
#10965=ORIENTED_EDGE('',*,*,#7568,.F.);
#10966=ORIENTED_EDGE('',*,*,#7562,.F.);
#10967=ORIENTED_EDGE('',*,*,#7570,.F.);
#10968=ORIENTED_EDGE('',*,*,#7571,.T.);
#10969=ORIENTED_EDGE('',*,*,#7572,.F.);
#10970=ORIENTED_EDGE('',*,*,#7573,.F.);
#10971=ORIENTED_EDGE('',*,*,#7574,.F.);
#10972=ORIENTED_EDGE('',*,*,#7573,.T.);
#10973=ORIENTED_EDGE('',*,*,#7575,.T.);
#10974=ORIENTED_EDGE('',*,*,#7576,.F.);
#10975=ORIENTED_EDGE('',*,*,#7575,.F.);
#10976=ORIENTED_EDGE('',*,*,#7572,.T.);
#10977=ORIENTED_EDGE('',*,*,#7577,.T.);
#10978=ORIENTED_EDGE('',*,*,#7578,.F.);
#10979=ORIENTED_EDGE('',*,*,#7577,.F.);
#10980=ORIENTED_EDGE('',*,*,#7571,.F.);
#10981=ORIENTED_EDGE('',*,*,#7579,.F.);
#10982=ORIENTED_EDGE('',*,*,#7580,.T.);
#10983=ORIENTED_EDGE('',*,*,#7581,.F.);
#10984=ORIENTED_EDGE('',*,*,#7582,.F.);
#10985=ORIENTED_EDGE('',*,*,#7583,.F.);
#10986=ORIENTED_EDGE('',*,*,#7582,.T.);
#10987=ORIENTED_EDGE('',*,*,#7584,.T.);
#10988=ORIENTED_EDGE('',*,*,#7585,.F.);
#10989=ORIENTED_EDGE('',*,*,#7584,.F.);
#10990=ORIENTED_EDGE('',*,*,#7581,.T.);
#10991=ORIENTED_EDGE('',*,*,#7586,.T.);
#10992=ORIENTED_EDGE('',*,*,#7587,.F.);
#10993=ORIENTED_EDGE('',*,*,#7586,.F.);
#10994=ORIENTED_EDGE('',*,*,#7580,.F.);
#10995=ORIENTED_EDGE('',*,*,#7588,.F.);
#10996=ORIENTED_EDGE('',*,*,#7589,.T.);
#10997=ORIENTED_EDGE('',*,*,#7590,.F.);
#10998=ORIENTED_EDGE('',*,*,#7591,.F.);
#10999=ORIENTED_EDGE('',*,*,#7592,.F.);
#11000=ORIENTED_EDGE('',*,*,#7591,.T.);
#11001=ORIENTED_EDGE('',*,*,#7593,.T.);
#11002=ORIENTED_EDGE('',*,*,#7594,.F.);
#11003=ORIENTED_EDGE('',*,*,#7593,.F.);
#11004=ORIENTED_EDGE('',*,*,#7590,.T.);
#11005=ORIENTED_EDGE('',*,*,#7595,.T.);
#11006=ORIENTED_EDGE('',*,*,#7596,.F.);
#11007=ORIENTED_EDGE('',*,*,#7595,.F.);
#11008=ORIENTED_EDGE('',*,*,#7589,.F.);
#11009=ORIENTED_EDGE('',*,*,#7597,.T.);
#11010=ORIENTED_EDGE('',*,*,#7598,.T.);
#11011=ORIENTED_EDGE('',*,*,#7599,.T.);
#11012=ORIENTED_EDGE('',*,*,#7598,.F.);
#11013=ORIENTED_EDGE('',*,*,#7597,.F.);
#11014=ORIENTED_EDGE('',*,*,#7600,.T.);
#11015=ORIENTED_EDGE('',*,*,#7601,.T.);
#11016=ORIENTED_EDGE('',*,*,#7600,.F.);
#11017=ORIENTED_EDGE('',*,*,#7602,.F.);
#11018=ORIENTED_EDGE('',*,*,#7599,.F.);
#11019=ORIENTED_EDGE('',*,*,#7603,.F.);
#11020=ORIENTED_EDGE('',*,*,#7244,.F.);
#11021=ORIENTED_EDGE('',*,*,#7096,.F.);
#11022=ORIENTED_EDGE('',*,*,#7245,.F.);
#11023=ORIENTED_EDGE('',*,*,#7604,.T.);
#11024=ORIENTED_EDGE('',*,*,#7603,.T.);
#11025=ORIENTED_EDGE('',*,*,#7604,.F.);
#11026=ORIENTED_EDGE('',*,*,#7164,.T.);
#11027=ORIENTED_EDGE('',*,*,#7241,.T.);
#11028=ORIENTED_EDGE('',*,*,#7605,.F.);
#11029=ORIENTED_EDGE('',*,*,#7250,.T.);
#11030=ORIENTED_EDGE('',*,*,#7601,.F.);
#11031=ORIENTED_EDGE('',*,*,#7605,.T.);
#11032=ORIENTED_EDGE('',*,*,#7240,.T.);
#11033=ORIENTED_EDGE('',*,*,#7172,.T.);
#11034=ORIENTED_EDGE('',*,*,#7169,.T.);
#11035=ORIENTED_EDGE('',*,*,#7249,.T.);
#11036=ORIENTED_EDGE('',*,*,#7606,.F.);
#11037=ORIENTED_EDGE('',*,*,#7607,.T.);
#11038=ORIENTED_EDGE('',*,*,#7602,.T.);
#11039=ORIENTED_EDGE('',*,*,#7607,.F.);
#11040=ORIENTED_EDGE('',*,*,#7271,.T.);
#11041=ORIENTED_EDGE('',*,*,#7608,.F.);
#11042=ORIENTED_EDGE('',*,*,#7585,.T.);
#11043=ORIENTED_EDGE('',*,*,#7587,.T.);
#11044=ORIENTED_EDGE('',*,*,#7579,.T.);
#11045=ORIENTED_EDGE('',*,*,#7609,.F.);
#11046=ORIENTED_EDGE('',*,*,#7286,.T.);
#11047=ORIENTED_EDGE('',*,*,#7288,.T.);
#11048=ORIENTED_EDGE('',*,*,#7280,.T.);
#11049=ORIENTED_EDGE('',*,*,#7610,.F.);
#11050=ORIENTED_EDGE('',*,*,#7576,.T.);
#11051=ORIENTED_EDGE('',*,*,#7578,.T.);
#11052=ORIENTED_EDGE('',*,*,#7570,.T.);
#11053=ORIENTED_EDGE('',*,*,#7611,.F.);
#11054=ORIENTED_EDGE('',*,*,#7295,.T.);
#11055=ORIENTED_EDGE('',*,*,#7297,.T.);
#11056=ORIENTED_EDGE('',*,*,#7289,.T.);
#11057=ORIENTED_EDGE('',*,*,#7612,.F.);
#11058=ORIENTED_EDGE('',*,*,#7567,.T.);
#11059=ORIENTED_EDGE('',*,*,#7569,.T.);
#11060=ORIENTED_EDGE('',*,*,#7561,.T.);
#11061=ORIENTED_EDGE('',*,*,#7613,.F.);
#11062=ORIENTED_EDGE('',*,*,#7304,.T.);
#11063=ORIENTED_EDGE('',*,*,#7306,.T.);
#11064=ORIENTED_EDGE('',*,*,#7298,.T.);
#11065=ORIENTED_EDGE('',*,*,#7614,.F.);
#11066=ORIENTED_EDGE('',*,*,#7558,.T.);
#11067=ORIENTED_EDGE('',*,*,#7560,.T.);
#11068=ORIENTED_EDGE('',*,*,#7552,.T.);
#11069=ORIENTED_EDGE('',*,*,#7615,.F.);
#11070=ORIENTED_EDGE('',*,*,#7313,.T.);
#11071=ORIENTED_EDGE('',*,*,#7315,.T.);
#11072=ORIENTED_EDGE('',*,*,#7307,.T.);
#11073=ORIENTED_EDGE('',*,*,#7616,.F.);
#11074=ORIENTED_EDGE('',*,*,#7549,.T.);
#11075=ORIENTED_EDGE('',*,*,#7551,.T.);
#11076=ORIENTED_EDGE('',*,*,#7543,.T.);
#11077=ORIENTED_EDGE('',*,*,#7617,.F.);
#11078=ORIENTED_EDGE('',*,*,#7322,.T.);
#11079=ORIENTED_EDGE('',*,*,#7324,.T.);
#11080=ORIENTED_EDGE('',*,*,#7316,.T.);
#11081=ORIENTED_EDGE('',*,*,#7618,.F.);
#11082=ORIENTED_EDGE('',*,*,#7540,.T.);
#11083=ORIENTED_EDGE('',*,*,#7542,.T.);
#11084=ORIENTED_EDGE('',*,*,#7534,.T.);
#11085=ORIENTED_EDGE('',*,*,#7619,.F.);
#11086=ORIENTED_EDGE('',*,*,#7331,.T.);
#11087=ORIENTED_EDGE('',*,*,#7333,.T.);
#11088=ORIENTED_EDGE('',*,*,#7325,.T.);
#11089=ORIENTED_EDGE('',*,*,#7620,.F.);
#11090=ORIENTED_EDGE('',*,*,#7531,.T.);
#11091=ORIENTED_EDGE('',*,*,#7533,.T.);
#11092=ORIENTED_EDGE('',*,*,#7525,.T.);
#11093=ORIENTED_EDGE('',*,*,#7621,.F.);
#11094=ORIENTED_EDGE('',*,*,#7340,.T.);
#11095=ORIENTED_EDGE('',*,*,#7342,.T.);
#11096=ORIENTED_EDGE('',*,*,#7334,.T.);
#11097=ORIENTED_EDGE('',*,*,#7622,.F.);
#11098=ORIENTED_EDGE('',*,*,#7522,.T.);
#11099=ORIENTED_EDGE('',*,*,#7524,.T.);
#11100=ORIENTED_EDGE('',*,*,#7516,.T.);
#11101=ORIENTED_EDGE('',*,*,#7623,.F.);
#11102=ORIENTED_EDGE('',*,*,#7350,.T.);
#11103=ORIENTED_EDGE('',*,*,#7352,.T.);
#11104=ORIENTED_EDGE('',*,*,#7624,.T.);
#11105=ORIENTED_EDGE('',*,*,#7606,.T.);
#11106=ORIENTED_EDGE('',*,*,#7624,.F.);
#11107=ORIENTED_EDGE('',*,*,#7353,.T.);
#11108=ORIENTED_EDGE('',*,*,#7343,.T.);
#11109=ORIENTED_EDGE('',*,*,#7625,.F.);
#11110=ORIENTED_EDGE('',*,*,#7360,.T.);
#11111=ORIENTED_EDGE('',*,*,#7362,.T.);
#11112=ORIENTED_EDGE('',*,*,#7354,.T.);
#11113=ORIENTED_EDGE('',*,*,#7626,.F.);
#11114=ORIENTED_EDGE('',*,*,#7504,.T.);
#11115=ORIENTED_EDGE('',*,*,#7506,.T.);
#11116=ORIENTED_EDGE('',*,*,#7498,.T.);
#11117=ORIENTED_EDGE('',*,*,#7627,.F.);
#11118=ORIENTED_EDGE('',*,*,#7369,.T.);
#11119=ORIENTED_EDGE('',*,*,#7371,.T.);
#11120=ORIENTED_EDGE('',*,*,#7363,.T.);
#11121=ORIENTED_EDGE('',*,*,#7628,.F.);
#11122=ORIENTED_EDGE('',*,*,#7495,.T.);
#11123=ORIENTED_EDGE('',*,*,#7497,.T.);
#11124=ORIENTED_EDGE('',*,*,#7489,.T.);
#11125=ORIENTED_EDGE('',*,*,#7629,.F.);
#11126=ORIENTED_EDGE('',*,*,#7378,.T.);
#11127=ORIENTED_EDGE('',*,*,#7380,.T.);
#11128=ORIENTED_EDGE('',*,*,#7372,.T.);
#11129=ORIENTED_EDGE('',*,*,#7630,.F.);
#11130=ORIENTED_EDGE('',*,*,#7486,.T.);
#11131=ORIENTED_EDGE('',*,*,#7488,.T.);
#11132=ORIENTED_EDGE('',*,*,#7480,.T.);
#11133=ORIENTED_EDGE('',*,*,#7631,.F.);
#11134=ORIENTED_EDGE('',*,*,#7387,.T.);
#11135=ORIENTED_EDGE('',*,*,#7389,.T.);
#11136=ORIENTED_EDGE('',*,*,#7381,.T.);
#11137=ORIENTED_EDGE('',*,*,#7632,.F.);
#11138=ORIENTED_EDGE('',*,*,#7477,.T.);
#11139=ORIENTED_EDGE('',*,*,#7479,.T.);
#11140=ORIENTED_EDGE('',*,*,#7471,.T.);
#11141=ORIENTED_EDGE('',*,*,#7633,.F.);
#11142=ORIENTED_EDGE('',*,*,#7396,.T.);
#11143=ORIENTED_EDGE('',*,*,#7398,.T.);
#11144=ORIENTED_EDGE('',*,*,#7390,.T.);
#11145=ORIENTED_EDGE('',*,*,#7634,.F.);
#11146=ORIENTED_EDGE('',*,*,#7468,.T.);
#11147=ORIENTED_EDGE('',*,*,#7470,.T.);
#11148=ORIENTED_EDGE('',*,*,#7462,.T.);
#11149=ORIENTED_EDGE('',*,*,#7635,.F.);
#11150=ORIENTED_EDGE('',*,*,#7405,.T.);
#11151=ORIENTED_EDGE('',*,*,#7407,.T.);
#11152=ORIENTED_EDGE('',*,*,#7399,.T.);
#11153=ORIENTED_EDGE('',*,*,#7636,.F.);
#11154=ORIENTED_EDGE('',*,*,#7459,.T.);
#11155=ORIENTED_EDGE('',*,*,#7461,.T.);
#11156=ORIENTED_EDGE('',*,*,#7453,.T.);
#11157=ORIENTED_EDGE('',*,*,#7637,.F.);
#11158=ORIENTED_EDGE('',*,*,#7414,.T.);
#11159=ORIENTED_EDGE('',*,*,#7416,.T.);
#11160=ORIENTED_EDGE('',*,*,#7408,.T.);
#11161=ORIENTED_EDGE('',*,*,#7638,.F.);
#11162=ORIENTED_EDGE('',*,*,#7450,.T.);
#11163=ORIENTED_EDGE('',*,*,#7452,.T.);
#11164=ORIENTED_EDGE('',*,*,#7444,.T.);
#11165=ORIENTED_EDGE('',*,*,#7639,.F.);
#11166=ORIENTED_EDGE('',*,*,#7423,.T.);
#11167=ORIENTED_EDGE('',*,*,#7425,.T.);
#11168=ORIENTED_EDGE('',*,*,#7417,.T.);
#11169=ORIENTED_EDGE('',*,*,#7640,.F.);
#11170=ORIENTED_EDGE('',*,*,#7441,.T.);
#11171=ORIENTED_EDGE('',*,*,#7443,.T.);
#11172=ORIENTED_EDGE('',*,*,#7435,.T.);
#11173=ORIENTED_EDGE('',*,*,#7641,.F.);
#11174=ORIENTED_EDGE('',*,*,#7432,.T.);
#11175=ORIENTED_EDGE('',*,*,#7434,.T.);
#11176=ORIENTED_EDGE('',*,*,#7426,.T.);
#11177=ORIENTED_EDGE('',*,*,#7642,.F.);
#11178=ORIENTED_EDGE('',*,*,#7513,.T.);
#11179=ORIENTED_EDGE('',*,*,#7515,.T.);
#11180=ORIENTED_EDGE('',*,*,#7510,.T.);
#11181=ORIENTED_EDGE('',*,*,#7643,.F.);
#11182=ORIENTED_EDGE('',*,*,#7594,.T.);
#11183=ORIENTED_EDGE('',*,*,#7596,.T.);
#11184=ORIENTED_EDGE('',*,*,#7588,.T.);
#11185=ORIENTED_EDGE('',*,*,#7644,.F.);
#11186=ORIENTED_EDGE('',*,*,#7277,.T.);
#11187=ORIENTED_EDGE('',*,*,#7279,.T.);
#11188=ORIENTED_EDGE('',*,*,#7645,.F.);
#11189=ORIENTED_EDGE('',*,*,#7646,.T.);
#11190=ORIENTED_EDGE('',*,*,#7349,.T.);
#11191=ORIENTED_EDGE('',*,*,#7623,.T.);
#11192=ORIENTED_EDGE('',*,*,#7520,.T.);
#11193=ORIENTED_EDGE('',*,*,#7622,.T.);
#11194=ORIENTED_EDGE('',*,*,#7338,.T.);
#11195=ORIENTED_EDGE('',*,*,#7621,.T.);
#11196=ORIENTED_EDGE('',*,*,#7529,.T.);
#11197=ORIENTED_EDGE('',*,*,#7620,.T.);
#11198=ORIENTED_EDGE('',*,*,#7329,.T.);
#11199=ORIENTED_EDGE('',*,*,#7619,.T.);
#11200=ORIENTED_EDGE('',*,*,#7538,.T.);
#11201=ORIENTED_EDGE('',*,*,#7618,.T.);
#11202=ORIENTED_EDGE('',*,*,#7320,.T.);
#11203=ORIENTED_EDGE('',*,*,#7617,.T.);
#11204=ORIENTED_EDGE('',*,*,#7547,.T.);
#11205=ORIENTED_EDGE('',*,*,#7616,.T.);
#11206=ORIENTED_EDGE('',*,*,#7311,.T.);
#11207=ORIENTED_EDGE('',*,*,#7615,.T.);
#11208=ORIENTED_EDGE('',*,*,#7556,.T.);
#11209=ORIENTED_EDGE('',*,*,#7614,.T.);
#11210=ORIENTED_EDGE('',*,*,#7302,.T.);
#11211=ORIENTED_EDGE('',*,*,#7613,.T.);
#11212=ORIENTED_EDGE('',*,*,#7565,.T.);
#11213=ORIENTED_EDGE('',*,*,#7612,.T.);
#11214=ORIENTED_EDGE('',*,*,#7293,.T.);
#11215=ORIENTED_EDGE('',*,*,#7611,.T.);
#11216=ORIENTED_EDGE('',*,*,#7574,.T.);
#11217=ORIENTED_EDGE('',*,*,#7610,.T.);
#11218=ORIENTED_EDGE('',*,*,#7284,.T.);
#11219=ORIENTED_EDGE('',*,*,#7609,.T.);
#11220=ORIENTED_EDGE('',*,*,#7583,.T.);
#11221=ORIENTED_EDGE('',*,*,#7608,.T.);
#11222=ORIENTED_EDGE('',*,*,#7275,.T.);
#11223=ORIENTED_EDGE('',*,*,#7644,.T.);
#11224=ORIENTED_EDGE('',*,*,#7592,.T.);
#11225=ORIENTED_EDGE('',*,*,#7643,.T.);
#11226=ORIENTED_EDGE('',*,*,#7507,.T.);
#11227=ORIENTED_EDGE('',*,*,#7642,.T.);
#11228=ORIENTED_EDGE('',*,*,#7430,.T.);
#11229=ORIENTED_EDGE('',*,*,#7641,.T.);
#11230=ORIENTED_EDGE('',*,*,#7439,.T.);
#11231=ORIENTED_EDGE('',*,*,#7640,.T.);
#11232=ORIENTED_EDGE('',*,*,#7421,.T.);
#11233=ORIENTED_EDGE('',*,*,#7639,.T.);
#11234=ORIENTED_EDGE('',*,*,#7448,.T.);
#11235=ORIENTED_EDGE('',*,*,#7638,.T.);
#11236=ORIENTED_EDGE('',*,*,#7412,.T.);
#11237=ORIENTED_EDGE('',*,*,#7637,.T.);
#11238=ORIENTED_EDGE('',*,*,#7457,.T.);
#11239=ORIENTED_EDGE('',*,*,#7636,.T.);
#11240=ORIENTED_EDGE('',*,*,#7403,.T.);
#11241=ORIENTED_EDGE('',*,*,#7635,.T.);
#11242=ORIENTED_EDGE('',*,*,#7466,.T.);
#11243=ORIENTED_EDGE('',*,*,#7634,.T.);
#11244=ORIENTED_EDGE('',*,*,#7394,.T.);
#11245=ORIENTED_EDGE('',*,*,#7633,.T.);
#11246=ORIENTED_EDGE('',*,*,#7475,.T.);
#11247=ORIENTED_EDGE('',*,*,#7632,.T.);
#11248=ORIENTED_EDGE('',*,*,#7385,.T.);
#11249=ORIENTED_EDGE('',*,*,#7631,.T.);
#11250=ORIENTED_EDGE('',*,*,#7484,.T.);
#11251=ORIENTED_EDGE('',*,*,#7630,.T.);
#11252=ORIENTED_EDGE('',*,*,#7376,.T.);
#11253=ORIENTED_EDGE('',*,*,#7629,.T.);
#11254=ORIENTED_EDGE('',*,*,#7493,.T.);
#11255=ORIENTED_EDGE('',*,*,#7628,.T.);
#11256=ORIENTED_EDGE('',*,*,#7367,.T.);
#11257=ORIENTED_EDGE('',*,*,#7627,.T.);
#11258=ORIENTED_EDGE('',*,*,#7502,.T.);
#11259=ORIENTED_EDGE('',*,*,#7626,.T.);
#11260=ORIENTED_EDGE('',*,*,#7358,.T.);
#11261=ORIENTED_EDGE('',*,*,#7625,.T.);
#11262=ORIENTED_EDGE('',*,*,#7347,.T.);
#11263=ORIENTED_EDGE('',*,*,#7646,.F.);
#11264=ORIENTED_EDGE('',*,*,#7645,.T.);
#11265=ORIENTED_EDGE('',*,*,#7253,.T.);
#11266=ORIENTED_EDGE('',*,*,#7269,.T.);
#11267=ORIENTED_EDGE('',*,*,#7266,.T.);
#11268=ORIENTED_EDGE('',*,*,#7263,.T.);
#11269=ORIENTED_EDGE('',*,*,#7260,.T.);
#11270=ORIENTED_EDGE('',*,*,#7257,.T.);
#11608=PLANE('',#13227);
#11609=PLANE('',#13234);
#11610=PLANE('',#13235);
#11611=PLANE('',#13236);
#11612=PLANE('',#13237);
#11613=PLANE('',#13238);
#11614=PLANE('',#13239);
#11615=PLANE('',#13240);
#11616=PLANE('',#13241);
#11617=PLANE('',#13242);
#11618=PLANE('',#13244);
#11619=PLANE('',#13245);
#11620=PLANE('',#13247);
#11621=PLANE('',#13248);
#11622=PLANE('',#13250);
#11623=PLANE('',#13251);
#11624=PLANE('',#13253);
#11625=PLANE('',#13254);
#11626=PLANE('',#13256);
#11627=PLANE('',#13257);
#11628=PLANE('',#13259);
#11629=PLANE('',#13260);
#11630=PLANE('',#13262);
#11631=PLANE('',#13263);
#11632=PLANE('',#13265);
#11633=PLANE('',#13266);
#11634=PLANE('',#13268);
#11635=PLANE('',#13269);
#11636=PLANE('',#13271);
#11637=PLANE('',#13272);
#11638=PLANE('',#13274);
#11639=PLANE('',#13275);
#11640=PLANE('',#13277);
#11641=PLANE('',#13278);
#11642=PLANE('',#13280);
#11643=PLANE('',#13281);
#11644=PLANE('',#13283);
#11645=PLANE('',#13284);
#11646=PLANE('',#13286);
#11647=PLANE('',#13287);
#11648=PLANE('',#13289);
#11649=PLANE('',#13290);
#11650=PLANE('',#13293);
#11651=PLANE('',#13294);
#11652=PLANE('',#13297);
#11653=PLANE('',#13298);
#11654=PLANE('',#13300);
#11655=PLANE('',#13301);
#11656=PLANE('',#13303);
#11657=PLANE('',#13304);
#11658=PLANE('',#13306);
#11659=PLANE('',#13307);
#11660=PLANE('',#13309);
#11661=PLANE('',#13310);
#11662=PLANE('',#13312);
#11663=PLANE('',#13313);
#11664=PLANE('',#13315);
#11665=PLANE('',#13316);
#11666=PLANE('',#13318);
#11667=PLANE('',#13319);
#11668=PLANE('',#13321);
#11669=PLANE('',#13322);
#11670=PLANE('',#13324);
#11671=PLANE('',#13325);
#11672=PLANE('',#13327);
#11673=PLANE('',#13328);
#11674=PLANE('',#13330);
#11675=PLANE('',#13331);
#11676=PLANE('',#13333);
#11677=PLANE('',#13334);
#11678=PLANE('',#13336);
#11679=PLANE('',#13337);
#11680=PLANE('',#13339);
#11681=PLANE('',#13340);
#11682=PLANE('',#13342);
#11683=PLANE('',#13343);
#11684=PLANE('',#13345);
#11685=PLANE('',#13346);
#11686=PLANE('',#13348);
#11687=PLANE('',#13349);
#11688=PLANE('',#13351);
#11689=PLANE('',#13352);
#11690=PLANE('',#13354);
#11691=PLANE('',#13355);
#11692=PLANE('',#13357);
#11693=PLANE('',#13358);
#11694=PLANE('',#13360);
#11695=PLANE('',#13361);
#11696=PLANE('',#13363);
#11697=PLANE('',#13364);
#11698=PLANE('',#13366);
#11699=PLANE('',#13367);
#11700=PLANE('',#13369);
#11701=PLANE('',#13370);
#11702=PLANE('',#13372);
#11703=PLANE('',#13373);
#11704=PLANE('',#13375);
#11705=PLANE('',#13376);
#11706=PLANE('',#13378);
#11707=PLANE('',#13379);
#11708=PLANE('',#13381);
#11709=PLANE('',#13382);
#11710=PLANE('',#13384);
#11711=PLANE('',#13385);
#11712=PLANE('',#13387);
#11713=PLANE('',#13388);
#11714=PLANE('',#13390);
#11715=PLANE('',#13391);
#11716=PLANE('',#13393);
#11717=PLANE('',#13394);
#11718=PLANE('',#13396);
#11719=PLANE('',#13397);
#11720=PLANE('',#13399);
#11721=PLANE('',#13401);
#11722=PLANE('',#13402);
#11723=PLANE('',#13403);
#11724=PLANE('',#13405);
#11725=PLANE('',#13406);
#11726=PLANE('',#13408);
#11727=PLANE('',#13409);
#11728=PLANE('',#13411);
#11729=PLANE('',#13412);
#11730=PLANE('',#13414);
#11731=PLANE('',#13415);
#11732=PLANE('',#13417);
#11733=PLANE('',#13418);
#11734=PLANE('',#13420);
#11735=PLANE('',#13421);
#11736=PLANE('',#13423);
#11737=PLANE('',#13424);
#11738=PLANE('',#13426);
#11739=PLANE('',#13427);
#11740=PLANE('',#13429);
#11741=PLANE('',#13430);
#11742=PLANE('',#13432);
#11743=PLANE('',#13433);
#11744=PLANE('',#13435);
#11745=PLANE('',#13436);
#11746=PLANE('',#13438);
#11747=PLANE('',#13439);
#11748=PLANE('',#13441);
#11749=PLANE('',#13442);
#11750=PLANE('',#13444);
#11751=PLANE('',#13445);
#11752=PLANE('',#13447);
#11753=PLANE('',#13448);
#11754=PLANE('',#13450);
#11755=PLANE('',#13451);
#11756=PLANE('',#13453);
#11757=PLANE('',#13454);
#11758=PLANE('',#13456);
#11759=PLANE('',#13457);
#11760=PLANE('',#13465);
#11761=PLANE('',#13467);
#11762=PLANE('',#13472);
#11763=PLANE('',#13514);
#12218=ADVANCED_FACE('',(#2251),#307,.T.);
#12219=ADVANCED_FACE('',(#2252),#308,.T.);
#12220=ADVANCED_FACE('',(#2253),#309,.T.);
#12221=ADVANCED_FACE('',(#2254),#310,.T.);
#12222=ADVANCED_FACE('',(#2255),#311,.T.);
#12223=ADVANCED_FACE('',(#2256),#312,.T.);
#12224=ADVANCED_FACE('',(#2257),#313,.T.);
#12225=ADVANCED_FACE('',(#2258),#314,.T.);
#12226=ADVANCED_FACE('',(#2259),#315,.T.);
#12227=ADVANCED_FACE('',(#2260),#316,.T.);
#12228=ADVANCED_FACE('',(#2261),#317,.T.);
#12229=ADVANCED_FACE('',(#2262),#318,.T.);
#12230=ADVANCED_FACE('',(#2263),#319,.T.);
#12231=ADVANCED_FACE('',(#2264),#320,.T.);
#12232=ADVANCED_FACE('',(#2265),#321,.T.);
#12233=ADVANCED_FACE('',(#2266),#322,.T.);
#12234=ADVANCED_FACE('',(#2267),#323,.T.);
#12235=ADVANCED_FACE('',(#2268),#324,.T.);
#12236=ADVANCED_FACE('',(#2269),#325,.T.);
#12237=ADVANCED_FACE('',(#2270),#326,.T.);
#12238=ADVANCED_FACE('',(#2271),#327,.T.);
#12239=ADVANCED_FACE('',(#2272),#328,.T.);
#12240=ADVANCED_FACE('',(#2273),#329,.T.);
#12241=ADVANCED_FACE('',(#2274),#330,.T.);
#12242=ADVANCED_FACE('',(#2275),#331,.T.);
#12243=ADVANCED_FACE('',(#2276),#332,.T.);
#12244=ADVANCED_FACE('',(#2277),#333,.T.);
#12245=ADVANCED_FACE('',(#2278),#334,.T.);
#12246=ADVANCED_FACE('',(#2279),#335,.T.);
#12247=ADVANCED_FACE('',(#2280),#336,.T.);
#12248=ADVANCED_FACE('',(#2281),#337,.T.);
#12249=ADVANCED_FACE('',(#2282),#338,.T.);
#12250=ADVANCED_FACE('',(#2283),#339,.T.);
#12251=ADVANCED_FACE('',(#2284),#340,.T.);
#12252=ADVANCED_FACE('',(#2285),#341,.T.);
#12253=ADVANCED_FACE('',(#2286),#342,.T.);
#12254=ADVANCED_FACE('',(#2287),#343,.T.);
#12255=ADVANCED_FACE('',(#2288),#344,.T.);
#12256=ADVANCED_FACE('',(#2289),#345,.T.);
#12257=ADVANCED_FACE('',(#2290),#346,.T.);
#12258=ADVANCED_FACE('',(#2291),#347,.T.);
#12259=ADVANCED_FACE('',(#2292),#348,.T.);
#12260=ADVANCED_FACE('',(#2293),#349,.T.);
#12261=ADVANCED_FACE('',(#2294),#350,.T.);
#12262=ADVANCED_FACE('',(#2295),#351,.T.);
#12263=ADVANCED_FACE('',(#2296),#352,.T.);
#12264=ADVANCED_FACE('',(#2297),#353,.T.);
#12265=ADVANCED_FACE('',(#2298),#354,.T.);
#12266=ADVANCED_FACE('',(#2299),#1332,.F.);
#12267=ADVANCED_FACE('',(#2300),#11608,.T.);
#12268=ADVANCED_FACE('',(#2301),#355,.T.);
#12269=ADVANCED_FACE('',(#2302),#1333,.F.);
#12270=ADVANCED_FACE('',(#2303),#437,.F.);
#12271=ADVANCED_FACE('',(#2304),#11609,.F.);
#12272=ADVANCED_FACE('',(#2305),#11610,.F.);
#12273=ADVANCED_FACE('',(#2306),#11611,.F.);
#12274=ADVANCED_FACE('',(#2307),#11612,.F.);
#12275=ADVANCED_FACE('',(#2308),#11613,.F.);
#12276=ADVANCED_FACE('',(#2309),#11614,.F.);
#12277=ADVANCED_FACE('',(#2310,#1397),#11615,.F.);
#12278=ADVANCED_FACE('',(#2311),#11616,.F.);
#12279=ADVANCED_FACE('',(#2312),#11617,.F.);
#12280=ADVANCED_FACE('',(#2313),#11618,.F.);
#12281=ADVANCED_FACE('',(#2314),#11619,.F.);
#12282=ADVANCED_FACE('',(#2315),#11620,.F.);
#12283=ADVANCED_FACE('',(#2316),#11621,.F.);
#12284=ADVANCED_FACE('',(#2317),#11622,.F.);
#12285=ADVANCED_FACE('',(#2318),#11623,.F.);
#12286=ADVANCED_FACE('',(#2319),#11624,.F.);
#12287=ADVANCED_FACE('',(#2320),#11625,.F.);
#12288=ADVANCED_FACE('',(#2321),#11626,.F.);
#12289=ADVANCED_FACE('',(#2322),#11627,.F.);
#12290=ADVANCED_FACE('',(#2323),#11628,.F.);
#12291=ADVANCED_FACE('',(#2324),#11629,.F.);
#12292=ADVANCED_FACE('',(#2325),#11630,.F.);
#12293=ADVANCED_FACE('',(#2326),#11631,.F.);
#12294=ADVANCED_FACE('',(#2327),#11632,.F.);
#12295=ADVANCED_FACE('',(#2328),#11633,.F.);
#12296=ADVANCED_FACE('',(#2329),#11634,.F.);
#12297=ADVANCED_FACE('',(#2330),#11635,.F.);
#12298=ADVANCED_FACE('',(#2331),#11636,.F.);
#12299=ADVANCED_FACE('',(#2332),#11637,.F.);
#12300=ADVANCED_FACE('',(#2333),#11638,.F.);
#12301=ADVANCED_FACE('',(#2334),#11639,.F.);
#12302=ADVANCED_FACE('',(#2335),#11640,.F.);
#12303=ADVANCED_FACE('',(#2336),#11641,.F.);
#12304=ADVANCED_FACE('',(#2337),#11642,.F.);
#12305=ADVANCED_FACE('',(#2338),#11643,.F.);
#12306=ADVANCED_FACE('',(#2339),#11644,.F.);
#12307=ADVANCED_FACE('',(#2340),#11645,.F.);
#12308=ADVANCED_FACE('',(#2341),#11646,.F.);
#12309=ADVANCED_FACE('',(#2342),#11647,.F.);
#12310=ADVANCED_FACE('',(#2343),#11648,.F.);
#12311=ADVANCED_FACE('',(#2344),#11649,.F.);
#12312=ADVANCED_FACE('',(#2345),#11650,.F.);
#12313=ADVANCED_FACE('',(#2346),#11651,.F.);
#12314=ADVANCED_FACE('',(#2347),#11652,.F.);
#12315=ADVANCED_FACE('',(#2348),#11653,.F.);
#12316=ADVANCED_FACE('',(#2349),#11654,.F.);
#12317=ADVANCED_FACE('',(#2350),#11655,.F.);
#12318=ADVANCED_FACE('',(#2351),#11656,.F.);
#12319=ADVANCED_FACE('',(#2352),#11657,.F.);
#12320=ADVANCED_FACE('',(#2353),#11658,.F.);
#12321=ADVANCED_FACE('',(#2354),#11659,.F.);
#12322=ADVANCED_FACE('',(#2355),#11660,.F.);
#12323=ADVANCED_FACE('',(#2356),#11661,.F.);
#12324=ADVANCED_FACE('',(#2357),#11662,.F.);
#12325=ADVANCED_FACE('',(#2358),#11663,.F.);
#12326=ADVANCED_FACE('',(#2359),#11664,.F.);
#12327=ADVANCED_FACE('',(#2360),#11665,.F.);
#12328=ADVANCED_FACE('',(#2361),#11666,.F.);
#12329=ADVANCED_FACE('',(#2362),#11667,.F.);
#12330=ADVANCED_FACE('',(#2363),#11668,.F.);
#12331=ADVANCED_FACE('',(#2364),#11669,.F.);
#12332=ADVANCED_FACE('',(#2365),#11670,.F.);
#12333=ADVANCED_FACE('',(#2366),#11671,.F.);
#12334=ADVANCED_FACE('',(#2367),#11672,.F.);
#12335=ADVANCED_FACE('',(#2368),#11673,.F.);
#12336=ADVANCED_FACE('',(#2369),#11674,.F.);
#12337=ADVANCED_FACE('',(#2370),#11675,.F.);
#12338=ADVANCED_FACE('',(#2371),#11676,.F.);
#12339=ADVANCED_FACE('',(#2372),#11677,.F.);
#12340=ADVANCED_FACE('',(#2373),#11678,.F.);
#12341=ADVANCED_FACE('',(#2374),#11679,.F.);
#12342=ADVANCED_FACE('',(#2375),#11680,.F.);
#12343=ADVANCED_FACE('',(#2376),#11681,.F.);
#12344=ADVANCED_FACE('',(#2377),#11682,.F.);
#12345=ADVANCED_FACE('',(#2378),#11683,.F.);
#12346=ADVANCED_FACE('',(#2379),#11684,.F.);
#12347=ADVANCED_FACE('',(#2380),#11685,.F.);
#12348=ADVANCED_FACE('',(#2381),#11686,.F.);
#12349=ADVANCED_FACE('',(#2382),#11687,.F.);
#12350=ADVANCED_FACE('',(#2383),#11688,.F.);
#12351=ADVANCED_FACE('',(#2384),#11689,.F.);
#12352=ADVANCED_FACE('',(#2385),#11690,.F.);
#12353=ADVANCED_FACE('',(#2386),#11691,.F.);
#12354=ADVANCED_FACE('',(#2387),#11692,.F.);
#12355=ADVANCED_FACE('',(#2388),#11693,.F.);
#12356=ADVANCED_FACE('',(#2389),#11694,.F.);
#12357=ADVANCED_FACE('',(#2390),#11695,.F.);
#12358=ADVANCED_FACE('',(#2391),#11696,.F.);
#12359=ADVANCED_FACE('',(#2392),#11697,.F.);
#12360=ADVANCED_FACE('',(#2393),#11698,.F.);
#12361=ADVANCED_FACE('',(#2394),#11699,.F.);
#12362=ADVANCED_FACE('',(#2395),#11700,.F.);
#12363=ADVANCED_FACE('',(#2396),#11701,.F.);
#12364=ADVANCED_FACE('',(#2397),#11702,.F.);
#12365=ADVANCED_FACE('',(#2398),#11703,.F.);
#12366=ADVANCED_FACE('',(#2399),#11704,.F.);
#12367=ADVANCED_FACE('',(#2400),#11705,.F.);
#12368=ADVANCED_FACE('',(#2401),#11706,.F.);
#12369=ADVANCED_FACE('',(#2402),#11707,.F.);
#12370=ADVANCED_FACE('',(#2403),#11708,.F.);
#12371=ADVANCED_FACE('',(#2404),#11709,.F.);
#12372=ADVANCED_FACE('',(#2405),#11710,.F.);
#12373=ADVANCED_FACE('',(#2406),#11711,.F.);
#12374=ADVANCED_FACE('',(#2407),#11712,.F.);
#12375=ADVANCED_FACE('',(#2408),#11713,.F.);
#12376=ADVANCED_FACE('',(#2409),#11714,.F.);
#12377=ADVANCED_FACE('',(#2410),#11715,.F.);
#12378=ADVANCED_FACE('',(#2411),#11716,.F.);
#12379=ADVANCED_FACE('',(#2412),#11717,.F.);
#12380=ADVANCED_FACE('',(#2413),#11718,.F.);
#12381=ADVANCED_FACE('',(#2414),#11719,.F.);
#12382=ADVANCED_FACE('',(#2415),#11720,.F.);
#12383=ADVANCED_FACE('',(#2416),#11721,.F.);
#12384=ADVANCED_FACE('',(#2417),#11722,.F.);
#12385=ADVANCED_FACE('',(#2418),#11723,.F.);
#12386=ADVANCED_FACE('',(#2419),#11724,.F.);
#12387=ADVANCED_FACE('',(#2420),#11725,.F.);
#12388=ADVANCED_FACE('',(#2421),#11726,.F.);
#12389=ADVANCED_FACE('',(#2422),#11727,.F.);
#12390=ADVANCED_FACE('',(#2423),#11728,.F.);
#12391=ADVANCED_FACE('',(#2424),#11729,.F.);
#12392=ADVANCED_FACE('',(#2425),#11730,.F.);
#12393=ADVANCED_FACE('',(#2426),#11731,.F.);
#12394=ADVANCED_FACE('',(#2427),#11732,.F.);
#12395=ADVANCED_FACE('',(#2428),#11733,.F.);
#12396=ADVANCED_FACE('',(#2429),#11734,.F.);
#12397=ADVANCED_FACE('',(#2430),#11735,.F.);
#12398=ADVANCED_FACE('',(#2431),#11736,.F.);
#12399=ADVANCED_FACE('',(#2432),#11737,.F.);
#12400=ADVANCED_FACE('',(#2433),#11738,.F.);
#12401=ADVANCED_FACE('',(#2434),#11739,.F.);
#12402=ADVANCED_FACE('',(#2435),#11740,.F.);
#12403=ADVANCED_FACE('',(#2436),#11741,.F.);
#12404=ADVANCED_FACE('',(#2437),#11742,.F.);
#12405=ADVANCED_FACE('',(#2438),#11743,.F.);
#12406=ADVANCED_FACE('',(#2439),#11744,.F.);
#12407=ADVANCED_FACE('',(#2440),#11745,.F.);
#12408=ADVANCED_FACE('',(#2441),#11746,.F.);
#12409=ADVANCED_FACE('',(#2442),#11747,.F.);
#12410=ADVANCED_FACE('',(#2443),#11748,.F.);
#12411=ADVANCED_FACE('',(#2444),#11749,.F.);
#12412=ADVANCED_FACE('',(#2445),#11750,.F.);
#12413=ADVANCED_FACE('',(#2446),#11751,.F.);
#12414=ADVANCED_FACE('',(#2447),#11752,.F.);
#12415=ADVANCED_FACE('',(#2448),#11753,.F.);
#12416=ADVANCED_FACE('',(#2449),#11754,.F.);
#12417=ADVANCED_FACE('',(#2450),#11755,.F.);
#12418=ADVANCED_FACE('',(#2451),#11756,.F.);
#12419=ADVANCED_FACE('',(#2452),#11757,.F.);
#12420=ADVANCED_FACE('',(#2453),#11758,.F.);
#12421=ADVANCED_FACE('',(#2454),#11759,.F.);
#12422=ADVANCED_FACE('',(#2455),#245,.F.);
#12423=ADVANCED_FACE('',(#2456),#356,.T.);
#12424=ADVANCED_FACE('',(#2457,#1398),#11760,.T.);
#12425=ADVANCED_FACE('',(#2458),#11761,.T.);
#12426=ADVANCED_FACE('',(#2459),#438,.T.);
#12427=ADVANCED_FACE('',(#2460),#357,.T.);
#12428=ADVANCED_FACE('',(#2461,#1399),#11762,.F.);
#12429=ADVANCED_FACE('',(#2462),#439,.T.);
#12430=ADVANCED_FACE('',(#2463),#358,.T.);
#12431=ADVANCED_FACE('',(#2464),#440,.T.);
#12432=ADVANCED_FACE('',(#2465,#1400),#11763,.T.);
#12488=CLOSED_SHELL('',(#12218,#12219,#12220,#12221,#12222,#12223,#12224,
#12225,#12226,#12227,#12228,#12229,#12230,#12231,#12232,#12233,#12234,#12235,
#12236,#12237,#12238,#12239,#12240,#12241,#12242,#12243,#12244,#12245,#12246,
#12247,#12248,#12249,#12250,#12251,#12252,#12253,#12254,#12255,#12256,#12257,
#12258,#12259,#12260,#12261,#12262,#12263,#12264,#12265,#12266,#12267,#12268,
#12269,#12270,#12271,#12272,#12273,#12274,#12275,#12276,#12277,#12278,#12279,
#12280,#12281,#12282,#12283,#12284,#12285,#12286,#12287,#12288,#12289,#12290,
#12291,#12292,#12293,#12294,#12295,#12296,#12297,#12298,#12299,#12300,#12301,
#12302,#12303,#12304,#12305,#12306,#12307,#12308,#12309,#12310,#12311,#12312,
#12313,#12314,#12315,#12316,#12317,#12318,#12319,#12320,#12321,#12322,#12323,
#12324,#12325,#12326,#12327,#12328,#12329,#12330,#12331,#12332,#12333,#12334,
#12335,#12336,#12337,#12338,#12339,#12340,#12341,#12342,#12343,#12344,#12345,
#12346,#12347,#12348,#12349,#12350,#12351,#12352,#12353,#12354,#12355,#12356,
#12357,#12358,#12359,#12360,#12361,#12362,#12363,#12364,#12365,#12366,#12367,
#12368,#12369,#12370,#12371,#12372,#12373,#12374,#12375,#12376,#12377,#12378,
#12379,#12380,#12381,#12382,#12383,#12384,#12385,#12386,#12387,#12388,#12389,
#12390,#12391,#12392,#12393,#12394,#12395,#12396,#12397,#12398,#12399,#12400,
#12401,#12402,#12403,#12404,#12405,#12406,#12407,#12408,#12409,#12410,#12411,
#12412,#12413,#12414,#12415,#12416,#12417,#12418,#12419,#12420,#12421,#12422,
#12423,#12424,#12425,#12426,#12427,#12428,#12429,#12430,#12431,#12432));
#13175=AXIS2_PLACEMENT_3D('',#26908,#15094,#15095);
#13176=AXIS2_PLACEMENT_3D('',#26909,#15096,#15097);
#13177=AXIS2_PLACEMENT_3D('',#26925,#15099,#15100);
#13178=AXIS2_PLACEMENT_3D('',#26933,#15101,#15102);
#13179=AXIS2_PLACEMENT_3D('',#26981,#15104,#15105);
#13180=AXIS2_PLACEMENT_3D('',#27029,#15107,#15108);
#13181=AXIS2_PLACEMENT_3D('',#27080,#15110,#15111);
#13182=AXIS2_PLACEMENT_3D('',#27131,#15113,#15114);
#13183=AXIS2_PLACEMENT_3D('',#27179,#15116,#15117);
#13184=AXIS2_PLACEMENT_3D('',#27227,#15119,#15120);
#13185=AXIS2_PLACEMENT_3D('',#27281,#15122,#15123);
#13186=AXIS2_PLACEMENT_3D('',#27329,#15125,#15126);
#13187=AXIS2_PLACEMENT_3D('',#27377,#15128,#15129);
#13188=AXIS2_PLACEMENT_3D('',#27431,#15131,#15132);
#13189=AXIS2_PLACEMENT_3D('',#27479,#15134,#15135);
#13190=AXIS2_PLACEMENT_3D('',#27527,#15137,#15138);
#13191=AXIS2_PLACEMENT_3D('',#27575,#15140,#15141);
#13192=AXIS2_PLACEMENT_3D('',#27629,#15143,#15144);
#13193=AXIS2_PLACEMENT_3D('',#27677,#15146,#15147);
#13194=AXIS2_PLACEMENT_3D('',#27725,#15149,#15150);
#13195=AXIS2_PLACEMENT_3D('',#27779,#15152,#15153);
#13196=AXIS2_PLACEMENT_3D('',#27827,#15155,#15156);
#13197=AXIS2_PLACEMENT_3D('',#27875,#15158,#15159);
#13198=AXIS2_PLACEMENT_3D('',#27926,#15161,#15162);
#13199=AXIS2_PLACEMENT_3D('',#27974,#15164,#15165);
#13200=AXIS2_PLACEMENT_3D('',#28022,#15167,#15168);
#13201=AXIS2_PLACEMENT_3D('',#28070,#15170,#15171);
#13202=AXIS2_PLACEMENT_3D('',#28079,#15173,#15174);
#13203=AXIS2_PLACEMENT_3D('',#28080,#15175,#15176);
#13204=AXIS2_PLACEMENT_3D('',#28095,#15178,#15179);
#13205=AXIS2_PLACEMENT_3D('',#28105,#15180,#15181);
#13206=AXIS2_PLACEMENT_3D('',#28129,#15183,#15184);
#13207=AXIS2_PLACEMENT_3D('',#28153,#15186,#15187);
#13208=AXIS2_PLACEMENT_3D('',#28178,#15189,#15190);
#13209=AXIS2_PLACEMENT_3D('',#28203,#15192,#15193);
#13210=AXIS2_PLACEMENT_3D('',#28227,#15195,#15196);
#13211=AXIS2_PLACEMENT_3D('',#28252,#15198,#15199);
#13212=AXIS2_PLACEMENT_3D('',#28277,#15201,#15202);
#13213=AXIS2_PLACEMENT_3D('',#28301,#15204,#15205);
#13214=AXIS2_PLACEMENT_3D('',#28326,#15207,#15208);
#13215=AXIS2_PLACEMENT_3D('',#28351,#15210,#15211);
#13216=AXIS2_PLACEMENT_3D('',#28375,#15213,#15214);
#13217=AXIS2_PLACEMENT_3D('',#28399,#15216,#15217);
#13218=AXIS2_PLACEMENT_3D('',#28424,#15219,#15220);
#13219=AXIS2_PLACEMENT_3D('',#28449,#15222,#15223);
#13220=AXIS2_PLACEMENT_3D('',#28473,#15225,#15226);
#13221=AXIS2_PLACEMENT_3D('',#28498,#15228,#15229);
#13222=AXIS2_PLACEMENT_3D('',#28523,#15231,#15232);
#13223=AXIS2_PLACEMENT_3D('',#28547,#15234,#15235);
#13224=AXIS2_PLACEMENT_3D('',#28572,#15237,#15238);
#13225=AXIS2_PLACEMENT_3D('',#28596,#15240,#15241);
#13226=AXIS2_PLACEMENT_3D('',#28621,#15243,#15244);
#13227=AXIS2_PLACEMENT_3D('',#29398,#15246,#15247);
#13228=AXIS2_PLACEMENT_3D('',#29400,#15248,#15249);
#13229=AXIS2_PLACEMENT_3D('',#29401,#15250,#15251);
#13230=AXIS2_PLACEMENT_3D('',#29461,#15252,#15253);
#13231=AXIS2_PLACEMENT_3D('',#29462,#15254,#15255);
#13232=AXIS2_PLACEMENT_3D('',#30153,#15256,#15257);
#13233=AXIS2_PLACEMENT_3D('',#30157,#15259,#15260);
#13234=AXIS2_PLACEMENT_3D('',#30158,#15261,#15262);
#13235=AXIS2_PLACEMENT_3D('',#30167,#15267,#15268);
#13236=AXIS2_PLACEMENT_3D('',#30173,#15272,#15273);
#13237=AXIS2_PLACEMENT_3D('',#30179,#15277,#15278);
#13238=AXIS2_PLACEMENT_3D('',#30185,#15282,#15283);
#13239=AXIS2_PLACEMENT_3D('',#30191,#15287,#15288);
#13240=AXIS2_PLACEMENT_3D('',#30194,#15291,#15292);
#13241=AXIS2_PLACEMENT_3D('',#30195,#15293,#15294);
#13242=AXIS2_PLACEMENT_3D('',#30204,#15299,#15300);
#13243=AXIS2_PLACEMENT_3D('',#30206,#15301,#15302);
#13244=AXIS2_PLACEMENT_3D('',#30208,#15304,#15305);
#13245=AXIS2_PLACEMENT_3D('',#30212,#15308,#15309);
#13246=AXIS2_PLACEMENT_3D('',#30213,#15310,#15311);
#13247=AXIS2_PLACEMENT_3D('',#30214,#15312,#15313);
#13248=AXIS2_PLACEMENT_3D('',#30223,#15318,#15319);
#13249=AXIS2_PLACEMENT_3D('',#30225,#15320,#15321);
#13250=AXIS2_PLACEMENT_3D('',#30227,#15323,#15324);
#13251=AXIS2_PLACEMENT_3D('',#30231,#15327,#15328);
#13252=AXIS2_PLACEMENT_3D('',#30232,#15329,#15330);
#13253=AXIS2_PLACEMENT_3D('',#30233,#15331,#15332);
#13254=AXIS2_PLACEMENT_3D('',#30242,#15337,#15338);
#13255=AXIS2_PLACEMENT_3D('',#30244,#15339,#15340);
#13256=AXIS2_PLACEMENT_3D('',#30246,#15342,#15343);
#13257=AXIS2_PLACEMENT_3D('',#30250,#15346,#15347);
#13258=AXIS2_PLACEMENT_3D('',#30251,#15348,#15349);
#13259=AXIS2_PLACEMENT_3D('',#30252,#15350,#15351);
#13260=AXIS2_PLACEMENT_3D('',#30261,#15356,#15357);
#13261=AXIS2_PLACEMENT_3D('',#30263,#15358,#15359);
#13262=AXIS2_PLACEMENT_3D('',#30265,#15361,#15362);
#13263=AXIS2_PLACEMENT_3D('',#30269,#15365,#15366);
#13264=AXIS2_PLACEMENT_3D('',#30270,#15367,#15368);
#13265=AXIS2_PLACEMENT_3D('',#30271,#15369,#15370);
#13266=AXIS2_PLACEMENT_3D('',#30280,#15375,#15376);
#13267=AXIS2_PLACEMENT_3D('',#30282,#15377,#15378);
#13268=AXIS2_PLACEMENT_3D('',#30284,#15380,#15381);
#13269=AXIS2_PLACEMENT_3D('',#30288,#15384,#15385);
#13270=AXIS2_PLACEMENT_3D('',#30289,#15386,#15387);
#13271=AXIS2_PLACEMENT_3D('',#30290,#15388,#15389);
#13272=AXIS2_PLACEMENT_3D('',#30299,#15394,#15395);
#13273=AXIS2_PLACEMENT_3D('',#30301,#15396,#15397);
#13274=AXIS2_PLACEMENT_3D('',#30303,#15399,#15400);
#13275=AXIS2_PLACEMENT_3D('',#30307,#15403,#15404);
#13276=AXIS2_PLACEMENT_3D('',#30308,#15405,#15406);
#13277=AXIS2_PLACEMENT_3D('',#30309,#15407,#15408);
#13278=AXIS2_PLACEMENT_3D('',#30318,#15413,#15414);
#13279=AXIS2_PLACEMENT_3D('',#30320,#15415,#15416);
#13280=AXIS2_PLACEMENT_3D('',#30322,#15418,#15419);
#13281=AXIS2_PLACEMENT_3D('',#30326,#15422,#15423);
#13282=AXIS2_PLACEMENT_3D('',#30327,#15424,#15425);
#13283=AXIS2_PLACEMENT_3D('',#30328,#15426,#15427);
#13284=AXIS2_PLACEMENT_3D('',#30337,#15432,#15433);
#13285=AXIS2_PLACEMENT_3D('',#30339,#15434,#15435);
#13286=AXIS2_PLACEMENT_3D('',#30341,#15437,#15438);
#13287=AXIS2_PLACEMENT_3D('',#30345,#15441,#15442);
#13288=AXIS2_PLACEMENT_3D('',#30346,#15443,#15444);
#13289=AXIS2_PLACEMENT_3D('',#30347,#15445,#15446);
#13290=AXIS2_PLACEMENT_3D('',#30356,#15451,#15452);
#13291=AXIS2_PLACEMENT_3D('',#30358,#15453,#15454);
#13292=AXIS2_PLACEMENT_3D('',#30361,#15456,#15457);
#13293=AXIS2_PLACEMENT_3D('',#30362,#15458,#15459);
#13294=AXIS2_PLACEMENT_3D('',#30366,#15462,#15463);
#13295=AXIS2_PLACEMENT_3D('',#30368,#15464,#15465);
#13296=AXIS2_PLACEMENT_3D('',#30369,#15466,#15467);
#13297=AXIS2_PLACEMENT_3D('',#30370,#15468,#15469);
#13298=AXIS2_PLACEMENT_3D('',#30379,#15474,#15475);
#13299=AXIS2_PLACEMENT_3D('',#30381,#15476,#15477);
#13300=AXIS2_PLACEMENT_3D('',#30383,#15479,#15480);
#13301=AXIS2_PLACEMENT_3D('',#30387,#15483,#15484);
#13302=AXIS2_PLACEMENT_3D('',#30388,#15485,#15486);
#13303=AXIS2_PLACEMENT_3D('',#30389,#15487,#15488);
#13304=AXIS2_PLACEMENT_3D('',#30398,#15493,#15494);
#13305=AXIS2_PLACEMENT_3D('',#30400,#15495,#15496);
#13306=AXIS2_PLACEMENT_3D('',#30402,#15498,#15499);
#13307=AXIS2_PLACEMENT_3D('',#30406,#15502,#15503);
#13308=AXIS2_PLACEMENT_3D('',#30407,#15504,#15505);
#13309=AXIS2_PLACEMENT_3D('',#30408,#15506,#15507);
#13310=AXIS2_PLACEMENT_3D('',#30417,#15512,#15513);
#13311=AXIS2_PLACEMENT_3D('',#30419,#15514,#15515);
#13312=AXIS2_PLACEMENT_3D('',#30421,#15517,#15518);
#13313=AXIS2_PLACEMENT_3D('',#30425,#15521,#15522);
#13314=AXIS2_PLACEMENT_3D('',#30426,#15523,#15524);
#13315=AXIS2_PLACEMENT_3D('',#30427,#15525,#15526);
#13316=AXIS2_PLACEMENT_3D('',#30436,#15531,#15532);
#13317=AXIS2_PLACEMENT_3D('',#30438,#15533,#15534);
#13318=AXIS2_PLACEMENT_3D('',#30440,#15536,#15537);
#13319=AXIS2_PLACEMENT_3D('',#30444,#15540,#15541);
#13320=AXIS2_PLACEMENT_3D('',#30445,#15542,#15543);
#13321=AXIS2_PLACEMENT_3D('',#30446,#15544,#15545);
#13322=AXIS2_PLACEMENT_3D('',#30455,#15550,#15551);
#13323=AXIS2_PLACEMENT_3D('',#30457,#15552,#15553);
#13324=AXIS2_PLACEMENT_3D('',#30459,#15555,#15556);
#13325=AXIS2_PLACEMENT_3D('',#30463,#15559,#15560);
#13326=AXIS2_PLACEMENT_3D('',#30464,#15561,#15562);
#13327=AXIS2_PLACEMENT_3D('',#30465,#15563,#15564);
#13328=AXIS2_PLACEMENT_3D('',#30474,#15569,#15570);
#13329=AXIS2_PLACEMENT_3D('',#30476,#15571,#15572);
#13330=AXIS2_PLACEMENT_3D('',#30478,#15574,#15575);
#13331=AXIS2_PLACEMENT_3D('',#30482,#15578,#15579);
#13332=AXIS2_PLACEMENT_3D('',#30483,#15580,#15581);
#13333=AXIS2_PLACEMENT_3D('',#30484,#15582,#15583);
#13334=AXIS2_PLACEMENT_3D('',#30493,#15588,#15589);
#13335=AXIS2_PLACEMENT_3D('',#30495,#15590,#15591);
#13336=AXIS2_PLACEMENT_3D('',#30497,#15593,#15594);
#13337=AXIS2_PLACEMENT_3D('',#30501,#15597,#15598);
#13338=AXIS2_PLACEMENT_3D('',#30502,#15599,#15600);
#13339=AXIS2_PLACEMENT_3D('',#30503,#15601,#15602);
#13340=AXIS2_PLACEMENT_3D('',#30512,#15607,#15608);
#13341=AXIS2_PLACEMENT_3D('',#30514,#15609,#15610);
#13342=AXIS2_PLACEMENT_3D('',#30516,#15612,#15613);
#13343=AXIS2_PLACEMENT_3D('',#30520,#15616,#15617);
#13344=AXIS2_PLACEMENT_3D('',#30521,#15618,#15619);
#13345=AXIS2_PLACEMENT_3D('',#30522,#15620,#15621);
#13346=AXIS2_PLACEMENT_3D('',#30531,#15626,#15627);
#13347=AXIS2_PLACEMENT_3D('',#30533,#15628,#15629);
#13348=AXIS2_PLACEMENT_3D('',#30535,#15631,#15632);
#13349=AXIS2_PLACEMENT_3D('',#30539,#15635,#15636);
#13350=AXIS2_PLACEMENT_3D('',#30540,#15637,#15638);
#13351=AXIS2_PLACEMENT_3D('',#30541,#15639,#15640);
#13352=AXIS2_PLACEMENT_3D('',#30550,#15645,#15646);
#13353=AXIS2_PLACEMENT_3D('',#30552,#15647,#15648);
#13354=AXIS2_PLACEMENT_3D('',#30554,#15650,#15651);
#13355=AXIS2_PLACEMENT_3D('',#30558,#15654,#15655);
#13356=AXIS2_PLACEMENT_3D('',#30559,#15656,#15657);
#13357=AXIS2_PLACEMENT_3D('',#30560,#15658,#15659);
#13358=AXIS2_PLACEMENT_3D('',#30569,#15664,#15665);
#13359=AXIS2_PLACEMENT_3D('',#30571,#15666,#15667);
#13360=AXIS2_PLACEMENT_3D('',#30573,#15669,#15670);
#13361=AXIS2_PLACEMENT_3D('',#30577,#15673,#15674);
#13362=AXIS2_PLACEMENT_3D('',#30578,#15675,#15676);
#13363=AXIS2_PLACEMENT_3D('',#30579,#15677,#15678);
#13364=AXIS2_PLACEMENT_3D('',#30588,#15683,#15684);
#13365=AXIS2_PLACEMENT_3D('',#30590,#15685,#15686);
#13366=AXIS2_PLACEMENT_3D('',#30592,#15688,#15689);
#13367=AXIS2_PLACEMENT_3D('',#30596,#15692,#15693);
#13368=AXIS2_PLACEMENT_3D('',#30597,#15694,#15695);
#13369=AXIS2_PLACEMENT_3D('',#30598,#15696,#15697);
#13370=AXIS2_PLACEMENT_3D('',#30607,#15702,#15703);
#13371=AXIS2_PLACEMENT_3D('',#30609,#15704,#15705);
#13372=AXIS2_PLACEMENT_3D('',#30611,#15707,#15708);
#13373=AXIS2_PLACEMENT_3D('',#30615,#15711,#15712);
#13374=AXIS2_PLACEMENT_3D('',#30616,#15713,#15714);
#13375=AXIS2_PLACEMENT_3D('',#30617,#15715,#15716);
#13376=AXIS2_PLACEMENT_3D('',#30626,#15721,#15722);
#13377=AXIS2_PLACEMENT_3D('',#30628,#15723,#15724);
#13378=AXIS2_PLACEMENT_3D('',#30630,#15726,#15727);
#13379=AXIS2_PLACEMENT_3D('',#30634,#15730,#15731);
#13380=AXIS2_PLACEMENT_3D('',#30635,#15732,#15733);
#13381=AXIS2_PLACEMENT_3D('',#30636,#15734,#15735);
#13382=AXIS2_PLACEMENT_3D('',#30645,#15740,#15741);
#13383=AXIS2_PLACEMENT_3D('',#30647,#15742,#15743);
#13384=AXIS2_PLACEMENT_3D('',#30649,#15745,#15746);
#13385=AXIS2_PLACEMENT_3D('',#30653,#15749,#15750);
#13386=AXIS2_PLACEMENT_3D('',#30654,#15751,#15752);
#13387=AXIS2_PLACEMENT_3D('',#30655,#15753,#15754);
#13388=AXIS2_PLACEMENT_3D('',#30664,#15759,#15760);
#13389=AXIS2_PLACEMENT_3D('',#30666,#15761,#15762);
#13390=AXIS2_PLACEMENT_3D('',#30668,#15764,#15765);
#13391=AXIS2_PLACEMENT_3D('',#30672,#15768,#15769);
#13392=AXIS2_PLACEMENT_3D('',#30673,#15770,#15771);
#13393=AXIS2_PLACEMENT_3D('',#30674,#15772,#15773);
#13394=AXIS2_PLACEMENT_3D('',#30683,#15778,#15779);
#13395=AXIS2_PLACEMENT_3D('',#30685,#15780,#15781);
#13396=AXIS2_PLACEMENT_3D('',#30687,#15783,#15784);
#13397=AXIS2_PLACEMENT_3D('',#30691,#15787,#15788);
#13398=AXIS2_PLACEMENT_3D('',#30692,#15789,#15790);
#13399=AXIS2_PLACEMENT_3D('',#30693,#15791,#15792);
#13400=AXIS2_PLACEMENT_3D('',#30696,#15793,#15794);
#13401=AXIS2_PLACEMENT_3D('',#30700,#15797,#15798);
#13402=AXIS2_PLACEMENT_3D('',#30706,#15802,#15803);
#13403=AXIS2_PLACEMENT_3D('',#30710,#15806,#15807);
#13404=AXIS2_PLACEMENT_3D('',#30711,#15808,#15809);
#13405=AXIS2_PLACEMENT_3D('',#30712,#15810,#15811);
#13406=AXIS2_PLACEMENT_3D('',#30721,#15816,#15817);
#13407=AXIS2_PLACEMENT_3D('',#30723,#15818,#15819);
#13408=AXIS2_PLACEMENT_3D('',#30725,#15821,#15822);
#13409=AXIS2_PLACEMENT_3D('',#30729,#15825,#15826);
#13410=AXIS2_PLACEMENT_3D('',#30730,#15827,#15828);
#13411=AXIS2_PLACEMENT_3D('',#30731,#15829,#15830);
#13412=AXIS2_PLACEMENT_3D('',#30740,#15835,#15836);
#13413=AXIS2_PLACEMENT_3D('',#30742,#15837,#15838);
#13414=AXIS2_PLACEMENT_3D('',#30744,#15840,#15841);
#13415=AXIS2_PLACEMENT_3D('',#30748,#15844,#15845);
#13416=AXIS2_PLACEMENT_3D('',#30749,#15846,#15847);
#13417=AXIS2_PLACEMENT_3D('',#30750,#15848,#15849);
#13418=AXIS2_PLACEMENT_3D('',#30759,#15854,#15855);
#13419=AXIS2_PLACEMENT_3D('',#30761,#15856,#15857);
#13420=AXIS2_PLACEMENT_3D('',#30763,#15859,#15860);
#13421=AXIS2_PLACEMENT_3D('',#30767,#15863,#15864);
#13422=AXIS2_PLACEMENT_3D('',#30768,#15865,#15866);
#13423=AXIS2_PLACEMENT_3D('',#30769,#15867,#15868);
#13424=AXIS2_PLACEMENT_3D('',#30778,#15873,#15874);
#13425=AXIS2_PLACEMENT_3D('',#30780,#15875,#15876);
#13426=AXIS2_PLACEMENT_3D('',#30782,#15878,#15879);
#13427=AXIS2_PLACEMENT_3D('',#30786,#15882,#15883);
#13428=AXIS2_PLACEMENT_3D('',#30787,#15884,#15885);
#13429=AXIS2_PLACEMENT_3D('',#30788,#15886,#15887);
#13430=AXIS2_PLACEMENT_3D('',#30797,#15892,#15893);
#13431=AXIS2_PLACEMENT_3D('',#30799,#15894,#15895);
#13432=AXIS2_PLACEMENT_3D('',#30801,#15897,#15898);
#13433=AXIS2_PLACEMENT_3D('',#30805,#15901,#15902);
#13434=AXIS2_PLACEMENT_3D('',#30806,#15903,#15904);
#13435=AXIS2_PLACEMENT_3D('',#30807,#15905,#15906);
#13436=AXIS2_PLACEMENT_3D('',#30816,#15911,#15912);
#13437=AXIS2_PLACEMENT_3D('',#30818,#15913,#15914);
#13438=AXIS2_PLACEMENT_3D('',#30820,#15916,#15917);
#13439=AXIS2_PLACEMENT_3D('',#30824,#15920,#15921);
#13440=AXIS2_PLACEMENT_3D('',#30825,#15922,#15923);
#13441=AXIS2_PLACEMENT_3D('',#30826,#15924,#15925);
#13442=AXIS2_PLACEMENT_3D('',#30835,#15930,#15931);
#13443=AXIS2_PLACEMENT_3D('',#30837,#15932,#15933);
#13444=AXIS2_PLACEMENT_3D('',#30839,#15935,#15936);
#13445=AXIS2_PLACEMENT_3D('',#30843,#15939,#15940);
#13446=AXIS2_PLACEMENT_3D('',#30844,#15941,#15942);
#13447=AXIS2_PLACEMENT_3D('',#30845,#15943,#15944);
#13448=AXIS2_PLACEMENT_3D('',#30854,#15949,#15950);
#13449=AXIS2_PLACEMENT_3D('',#30856,#15951,#15952);
#13450=AXIS2_PLACEMENT_3D('',#30858,#15954,#15955);
#13451=AXIS2_PLACEMENT_3D('',#30862,#15958,#15959);
#13452=AXIS2_PLACEMENT_3D('',#30863,#15960,#15961);
#13453=AXIS2_PLACEMENT_3D('',#30864,#15962,#15963);
#13454=AXIS2_PLACEMENT_3D('',#30873,#15968,#15969);
#13455=AXIS2_PLACEMENT_3D('',#30875,#15970,#15971);
#13456=AXIS2_PLACEMENT_3D('',#30877,#15973,#15974);
#13457=AXIS2_PLACEMENT_3D('',#30881,#15977,#15978);
#13458=AXIS2_PLACEMENT_3D('',#30882,#15979,#15980);
#13459=AXIS2_PLACEMENT_3D('',#30883,#15981,#15982);
#13460=AXIS2_PLACEMENT_3D('',#30885,#15983,#15984);
#13461=AXIS2_PLACEMENT_3D('',#30887,#15985,#15986);
#13462=AXIS2_PLACEMENT_3D('',#30888,#15987,#15988);
#13463=AXIS2_PLACEMENT_3D('',#30889,#15989,#15990);
#13464=AXIS2_PLACEMENT_3D('',#30892,#15992,#15993);
#13465=AXIS2_PLACEMENT_3D('',#30893,#15994,#15995);
#13466=AXIS2_PLACEMENT_3D('',#30895,#15996,#15997);
#13467=AXIS2_PLACEMENT_3D('',#30896,#15998,#15999);
#13468=AXIS2_PLACEMENT_3D('',#30898,#16000,#16001);
#13469=AXIS2_PLACEMENT_3D('',#30899,#16002,#16003);
#13470=AXIS2_PLACEMENT_3D('',#30901,#16005,#16006);
#13471=AXIS2_PLACEMENT_3D('',#30902,#16007,#16008);
#13472=AXIS2_PLACEMENT_3D('',#30903,#16009,#16010);
#13473=AXIS2_PLACEMENT_3D('',#30904,#16011,#16012);
#13474=AXIS2_PLACEMENT_3D('',#30906,#16013,#16014);
#13475=AXIS2_PLACEMENT_3D('',#30908,#16016,#16017);
#13476=AXIS2_PLACEMENT_3D('',#30909,#16018,#16019);
#13477=AXIS2_PLACEMENT_3D('',#30910,#16020,#16021);
#13478=AXIS2_PLACEMENT_3D('',#30911,#16022,#16023);
#13479=AXIS2_PLACEMENT_3D('',#30912,#16024,#16025);
#13480=AXIS2_PLACEMENT_3D('',#30913,#16026,#16027);
#13481=AXIS2_PLACEMENT_3D('',#30914,#16028,#16029);
#13482=AXIS2_PLACEMENT_3D('',#30915,#16030,#16031);
#13483=AXIS2_PLACEMENT_3D('',#30916,#16032,#16033);
#13484=AXIS2_PLACEMENT_3D('',#30917,#16034,#16035);
#13485=AXIS2_PLACEMENT_3D('',#30918,#16036,#16037);
#13486=AXIS2_PLACEMENT_3D('',#30919,#16038,#16039);
#13487=AXIS2_PLACEMENT_3D('',#30920,#16040,#16041);
#13488=AXIS2_PLACEMENT_3D('',#30921,#16042,#16043);
#13489=AXIS2_PLACEMENT_3D('',#30922,#16044,#16045);
#13490=AXIS2_PLACEMENT_3D('',#30923,#16046,#16047);
#13491=AXIS2_PLACEMENT_3D('',#30924,#16048,#16049);
#13492=AXIS2_PLACEMENT_3D('',#30926,#16051,#16052);
#13493=AXIS2_PLACEMENT_3D('',#30927,#16053,#16054);
#13494=AXIS2_PLACEMENT_3D('',#30928,#16055,#16056);
#13495=AXIS2_PLACEMENT_3D('',#30929,#16057,#16058);
#13496=AXIS2_PLACEMENT_3D('',#30930,#16059,#16060);
#13497=AXIS2_PLACEMENT_3D('',#30931,#16061,#16062);
#13498=AXIS2_PLACEMENT_3D('',#30932,#16063,#16064);
#13499=AXIS2_PLACEMENT_3D('',#30933,#16065,#16066);
#13500=AXIS2_PLACEMENT_3D('',#30934,#16067,#16068);
#13501=AXIS2_PLACEMENT_3D('',#30935,#16069,#16070);
#13502=AXIS2_PLACEMENT_3D('',#30936,#16071,#16072);
#13503=AXIS2_PLACEMENT_3D('',#30937,#16073,#16074);
#13504=AXIS2_PLACEMENT_3D('',#30938,#16075,#16076);
#13505=AXIS2_PLACEMENT_3D('',#30939,#16077,#16078);
#13506=AXIS2_PLACEMENT_3D('',#30940,#16079,#16080);
#13507=AXIS2_PLACEMENT_3D('',#30941,#16081,#16082);
#13508=AXIS2_PLACEMENT_3D('',#30942,#16083,#16084);
#13509=AXIS2_PLACEMENT_3D('',#30943,#16085,#16086);
#13510=AXIS2_PLACEMENT_3D('',#30944,#16087,#16088);
#13511=AXIS2_PLACEMENT_3D('',#30945,#16089,#16090);
#13512=AXIS2_PLACEMENT_3D('',#30946,#16091,#16092);
#13513=AXIS2_PLACEMENT_3D('',#30948,#16093,#16094);
#13514=AXIS2_PLACEMENT_3D('',#30950,#16096,#16097);
#15094=DIRECTION('axis',(0.,0.,1.));
#15095=DIRECTION('refdir',(1.,0.,0.));
#15096=DIRECTION('center_axis',(0.,0.,1.));
#15097=DIRECTION('ref_axis',(1.,0.,0.));
#15098=DIRECTION('',(0.,0.,-1.));
#15099=DIRECTION('center_axis',(0.,0.,1.));
#15100=DIRECTION('ref_axis',(1.,0.,0.));
#15101=DIRECTION('center_axis',(0.,0.,1.));
#15102=DIRECTION('ref_axis',(1.,0.,0.));
#15103=DIRECTION('',(0.,0.,-1.));
#15104=DIRECTION('center_axis',(0.,0.,1.));
#15105=DIRECTION('ref_axis',(1.,0.,0.));
#15106=DIRECTION('',(0.,0.,-1.));
#15107=DIRECTION('center_axis',(0.,0.,1.));
#15108=DIRECTION('ref_axis',(1.,0.,0.));
#15109=DIRECTION('',(0.,0.,-1.));
#15110=DIRECTION('center_axis',(0.,0.,1.));
#15111=DIRECTION('ref_axis',(1.,0.,0.));
#15112=DIRECTION('',(0.,0.,-1.));
#15113=DIRECTION('center_axis',(0.,0.,1.));
#15114=DIRECTION('ref_axis',(1.,0.,0.));
#15115=DIRECTION('',(0.,0.,-1.));
#15116=DIRECTION('center_axis',(0.,0.,1.));
#15117=DIRECTION('ref_axis',(1.,0.,0.));
#15118=DIRECTION('',(0.,0.,-1.));
#15119=DIRECTION('center_axis',(0.,0.,1.));
#15120=DIRECTION('ref_axis',(1.,0.,0.));
#15121=DIRECTION('',(0.,0.,-1.));
#15122=DIRECTION('center_axis',(0.,0.,1.));
#15123=DIRECTION('ref_axis',(1.,0.,0.));
#15124=DIRECTION('',(0.,0.,-1.));
#15125=DIRECTION('center_axis',(0.,0.,1.));
#15126=DIRECTION('ref_axis',(1.,0.,0.));
#15127=DIRECTION('',(0.,0.,-1.));
#15128=DIRECTION('center_axis',(0.,0.,1.));
#15129=DIRECTION('ref_axis',(1.,0.,0.));
#15130=DIRECTION('',(0.,0.,-1.));
#15131=DIRECTION('center_axis',(0.,0.,1.));
#15132=DIRECTION('ref_axis',(1.,0.,0.));
#15133=DIRECTION('',(0.,0.,-1.));
#15134=DIRECTION('center_axis',(0.,0.,1.));
#15135=DIRECTION('ref_axis',(1.,0.,0.));
#15136=DIRECTION('',(0.,0.,-1.));
#15137=DIRECTION('center_axis',(0.,0.,1.));
#15138=DIRECTION('ref_axis',(1.,0.,0.));
#15139=DIRECTION('',(0.,0.,-1.));
#15140=DIRECTION('center_axis',(0.,0.,1.));
#15141=DIRECTION('ref_axis',(1.,0.,0.));
#15142=DIRECTION('',(0.,0.,-1.));
#15143=DIRECTION('center_axis',(0.,0.,1.));
#15144=DIRECTION('ref_axis',(1.,0.,0.));
#15145=DIRECTION('',(0.,0.,-1.));
#15146=DIRECTION('center_axis',(0.,0.,1.));
#15147=DIRECTION('ref_axis',(1.,0.,0.));
#15148=DIRECTION('',(0.,0.,-1.));
#15149=DIRECTION('center_axis',(0.,0.,1.));
#15150=DIRECTION('ref_axis',(1.,0.,0.));
#15151=DIRECTION('',(0.,0.,-1.));
#15152=DIRECTION('center_axis',(0.,0.,1.));
#15153=DIRECTION('ref_axis',(1.,0.,0.));
#15154=DIRECTION('',(0.,0.,-1.));
#15155=DIRECTION('center_axis',(0.,0.,1.));
#15156=DIRECTION('ref_axis',(1.,0.,0.));
#15157=DIRECTION('',(0.,0.,-1.));
#15158=DIRECTION('center_axis',(0.,0.,1.));
#15159=DIRECTION('ref_axis',(1.,0.,0.));
#15160=DIRECTION('',(0.,0.,-1.));
#15161=DIRECTION('center_axis',(0.,0.,1.));
#15162=DIRECTION('ref_axis',(1.,0.,0.));
#15163=DIRECTION('',(0.,0.,-1.));
#15164=DIRECTION('center_axis',(0.,0.,1.));
#15165=DIRECTION('ref_axis',(1.,0.,0.));
#15166=DIRECTION('',(0.,0.,-1.));
#15167=DIRECTION('center_axis',(0.,0.,1.));
#15168=DIRECTION('ref_axis',(1.,0.,0.));
#15169=DIRECTION('',(0.,0.,-1.));
#15170=DIRECTION('center_axis',(0.,0.,1.));
#15171=DIRECTION('ref_axis',(1.,-8.50999688392278E-15,0.));
#15172=DIRECTION('',(0.,0.,1.));
#15173=DIRECTION('center_axis',(0.,0.,1.));
#15174=DIRECTION('ref_axis',(1.,-8.50999688392278E-15,0.));
#15175=DIRECTION('center_axis',(0.,0.,1.));
#15176=DIRECTION('ref_axis',(1.,-8.50999688392278E-15,0.));
#15177=DIRECTION('',(0.,0.,1.));
#15178=DIRECTION('center_axis',(0.,0.,1.));
#15179=DIRECTION('ref_axis',(1.,-8.50999688392278E-15,0.));
#15180=DIRECTION('center_axis',(0.,0.,1.));
#15181=DIRECTION('ref_axis',(1.,-8.50999688392278E-15,0.));
#15182=DIRECTION('',(0.,0.,1.));
#15183=DIRECTION('center_axis',(0.,0.,1.));
#15184=DIRECTION('ref_axis',(1.,-8.50999688392278E-15,0.));
#15185=DIRECTION('',(0.,0.,1.));
#15186=DIRECTION('center_axis',(0.,0.,1.));
#15187=DIRECTION('ref_axis',(1.,-8.50999688392278E-15,0.));
#15188=DIRECTION('',(0.,0.,1.));
#15189=DIRECTION('center_axis',(0.,0.,1.));
#15190=DIRECTION('ref_axis',(1.,-8.50999688392278E-15,0.));
#15191=DIRECTION('',(0.,0.,1.));
#15192=DIRECTION('center_axis',(0.,0.,1.));
#15193=DIRECTION('ref_axis',(1.,-8.50999688392278E-15,0.));
#15194=DIRECTION('',(0.,0.,1.));
#15195=DIRECTION('center_axis',(0.,0.,1.));
#15196=DIRECTION('ref_axis',(1.,-8.50999688392278E-15,0.));
#15197=DIRECTION('',(0.,0.,1.));
#15198=DIRECTION('center_axis',(0.,0.,1.));
#15199=DIRECTION('ref_axis',(1.,-8.50999688392278E-15,0.));
#15200=DIRECTION('',(0.,0.,1.));
#15201=DIRECTION('center_axis',(0.,0.,1.));
#15202=DIRECTION('ref_axis',(1.,-8.50999688392278E-15,0.));
#15203=DIRECTION('',(0.,0.,1.));
#15204=DIRECTION('center_axis',(0.,0.,1.));
#15205=DIRECTION('ref_axis',(1.,-8.50999688392278E-15,0.));
#15206=DIRECTION('',(0.,0.,1.));
#15207=DIRECTION('center_axis',(0.,0.,1.));
#15208=DIRECTION('ref_axis',(1.,-8.50999688392278E-15,0.));
#15209=DIRECTION('',(0.,0.,1.));
#15210=DIRECTION('center_axis',(0.,0.,1.));
#15211=DIRECTION('ref_axis',(1.,-8.50999688392278E-15,0.));
#15212=DIRECTION('',(0.,0.,1.));
#15213=DIRECTION('center_axis',(0.,0.,1.));
#15214=DIRECTION('ref_axis',(1.,-8.50999688392278E-15,0.));
#15215=DIRECTION('',(0.,0.,1.));
#15216=DIRECTION('center_axis',(0.,0.,1.));
#15217=DIRECTION('ref_axis',(1.,-8.50999688392278E-15,0.));
#15218=DIRECTION('',(0.,0.,1.));
#15219=DIRECTION('center_axis',(0.,0.,1.));
#15220=DIRECTION('ref_axis',(1.,-8.50999688392278E-15,0.));
#15221=DIRECTION('',(0.,0.,1.));
#15222=DIRECTION('center_axis',(0.,0.,1.));
#15223=DIRECTION('ref_axis',(1.,-8.50999688392278E-15,0.));
#15224=DIRECTION('',(0.,0.,1.));
#15225=DIRECTION('center_axis',(0.,0.,1.));
#15226=DIRECTION('ref_axis',(1.,-8.50999688392278E-15,0.));
#15227=DIRECTION('',(0.,0.,1.));
#15228=DIRECTION('center_axis',(0.,0.,1.));
#15229=DIRECTION('ref_axis',(1.,-8.50999688392278E-15,0.));
#15230=DIRECTION('',(0.,0.,1.));
#15231=DIRECTION('center_axis',(0.,0.,1.));
#15232=DIRECTION('ref_axis',(1.,-8.50999688392278E-15,0.));
#15233=DIRECTION('',(0.,0.,1.));
#15234=DIRECTION('center_axis',(0.,0.,1.));
#15235=DIRECTION('ref_axis',(1.,-8.50999688392278E-15,0.));
#15236=DIRECTION('',(0.,0.,1.));
#15237=DIRECTION('center_axis',(0.,0.,1.));
#15238=DIRECTION('ref_axis',(1.,-8.50999688392278E-15,0.));
#15239=DIRECTION('',(0.,0.,1.));
#15240=DIRECTION('center_axis',(0.,0.,1.));
#15241=DIRECTION('ref_axis',(1.,-8.50999688392278E-15,0.));
#15242=DIRECTION('',(0.,0.,1.));
#15243=DIRECTION('center_axis',(0.,0.,1.));
#15244=DIRECTION('ref_axis',(1.,-8.50999688392278E-15,0.));
#15245=DIRECTION('',(0.,0.,1.));
#15246=DIRECTION('center_axis',(0.,0.,1.));
#15247=DIRECTION('ref_axis',(1.,0.,0.));
#15248=DIRECTION('center_axis',(0.,0.,1.));
#15249=DIRECTION('ref_axis',(1.,0.,0.));
#15250=DIRECTION('center_axis',(0.,0.,1.));
#15251=DIRECTION('ref_axis',(1.,0.,0.));
#15252=DIRECTION('center_axis',(0.,0.,-1.));
#15253=DIRECTION('ref_axis',(1.,-8.50999688392278E-15,0.));
#15254=DIRECTION('center_axis',(0.,0.,1.));
#15255=DIRECTION('ref_axis',(1.,-8.50999688392278E-15,0.));
#15256=DIRECTION('center_axis',(0.,0.,1.));
#15257=DIRECTION('ref_axis',(1.,0.,0.));
#15258=DIRECTION('',(-0.857492925712544,-1.05012596676537E-16,0.514495755427526));
#15259=DIRECTION('center_axis',(0.,0.,-1.));
#15260=DIRECTION('ref_axis',(1.,0.,0.));
#15261=DIRECTION('center_axis',(0.866025403784439,0.5,0.));
#15262=DIRECTION('ref_axis',(0.5,-0.866025403784439,0.));
#15263=DIRECTION('',(0.5,-0.866025403784439,0.));
#15264=DIRECTION('',(0.,0.,-1.));
#15265=DIRECTION('',(0.5,-0.866025403784439,0.));
#15266=DIRECTION('',(0.,0.,-1.));
#15267=DIRECTION('center_axis',(1.92296268638356E-16,1.,0.));
#15268=DIRECTION('ref_axis',(1.,-1.92296268638356E-16,0.));
#15269=DIRECTION('',(1.,-1.92296268638356E-16,0.));
#15270=DIRECTION('',(0.,0.,-1.));
#15271=DIRECTION('',(1.,-1.92296268638356E-16,0.));
#15272=DIRECTION('center_axis',(-0.866025403784438,0.5,0.));
#15273=DIRECTION('ref_axis',(0.5,0.866025403784438,0.));
#15274=DIRECTION('',(0.5,0.866025403784438,0.));
#15275=DIRECTION('',(0.,0.,-1.));
#15276=DIRECTION('',(0.5,0.866025403784438,0.));
#15277=DIRECTION('center_axis',(-0.866025403784439,-0.5,0.));
#15278=DIRECTION('ref_axis',(-0.5,0.866025403784439,0.));
#15279=DIRECTION('',(-0.5,0.866025403784439,0.));
#15280=DIRECTION('',(0.,0.,-1.));
#15281=DIRECTION('',(-0.5,0.866025403784439,0.));
#15282=DIRECTION('center_axis',(-1.92296268638356E-16,-1.,0.));
#15283=DIRECTION('ref_axis',(-1.,1.92296268638356E-16,0.));
#15284=DIRECTION('',(-1.,1.92296268638356E-16,0.));
#15285=DIRECTION('',(0.,0.,-1.));
#15286=DIRECTION('',(-1.,1.92296268638356E-16,0.));
#15287=DIRECTION('center_axis',(0.866025403784439,-0.5,0.));
#15288=DIRECTION('ref_axis',(-0.5,-0.866025403784439,0.));
#15289=DIRECTION('',(-0.5,-0.866025403784439,0.));
#15290=DIRECTION('',(-0.5,-0.866025403784439,0.));
#15291=DIRECTION('center_axis',(0.,0.,-1.));
#15292=DIRECTION('ref_axis',(-1.,0.,0.));
#15293=DIRECTION('center_axis',(-0.713210659190727,-0.700949752561999,0.));
#15294=DIRECTION('ref_axis',(-0.700949752561999,0.713210659190727,0.));
#15295=DIRECTION('',(0.,0.,1.));
#15296=DIRECTION('',(-0.700949752561999,0.713210659190727,0.));
#15297=DIRECTION('',(0.,0.,-1.));
#15298=DIRECTION('',(-0.700949752561999,0.713210659190727,0.));
#15299=DIRECTION('center_axis',(0.,0.,1.));
#15300=DIRECTION('ref_axis',(1.,0.,0.));
#15301=DIRECTION('center_axis',(0.,0.,1.));
#15302=DIRECTION('ref_axis',(1.,0.,0.));
#15303=DIRECTION('',(0.995401637679912,0.0957892462865752,0.));
#15304=DIRECTION('center_axis',(-0.0957892462865752,0.995401637679912,0.));
#15305=DIRECTION('ref_axis',(0.995401637679912,0.0957892462865752,0.));
#15306=DIRECTION('',(0.,0.,-1.));
#15307=DIRECTION('',(0.995401637679912,0.0957892462865752,0.));
#15308=DIRECTION('center_axis',(0.,0.,-1.));
#15309=DIRECTION('ref_axis',(-1.,0.,0.));
#15310=DIRECTION('center_axis',(0.,0.,-1.));
#15311=DIRECTION('ref_axis',(1.,0.,0.));
#15312=DIRECTION('center_axis',(-0.909937728342724,-0.414744898146418,0.));
#15313=DIRECTION('ref_axis',(-0.414744898146418,0.909937728342724,0.));
#15314=DIRECTION('',(0.,0.,1.));
#15315=DIRECTION('',(-0.414744898146418,0.909937728342724,0.));
#15316=DIRECTION('',(0.,0.,-1.));
#15317=DIRECTION('',(-0.414744898146418,0.909937728342724,0.));
#15318=DIRECTION('center_axis',(0.,0.,1.));
#15319=DIRECTION('ref_axis',(1.,0.,0.));
#15320=DIRECTION('center_axis',(0.,0.,1.));
#15321=DIRECTION('ref_axis',(1.,0.,0.));
#15322=DIRECTION('',(0.968133425390015,-0.250434962899744,0.));
#15323=DIRECTION('center_axis',(0.250434962899744,0.968133425390015,0.));
#15324=DIRECTION('ref_axis',(0.968133425390015,-0.250434962899744,0.));
#15325=DIRECTION('',(0.,0.,-1.));
#15326=DIRECTION('',(0.968133425390015,-0.250434962899744,0.));
#15327=DIRECTION('center_axis',(0.,0.,-1.));
#15328=DIRECTION('ref_axis',(-1.,0.,0.));
#15329=DIRECTION('center_axis',(0.,0.,-1.));
#15330=DIRECTION('ref_axis',(1.,0.,0.));
#15331=DIRECTION('center_axis',(-0.996912878205979,-0.0785156880315736,
0.));
#15332=DIRECTION('ref_axis',(-0.0785156880315736,0.996912878205979,0.));
#15333=DIRECTION('',(0.,0.,1.));
#15334=DIRECTION('',(-0.0785156880315736,0.996912878205979,0.));
#15335=DIRECTION('',(0.,0.,-1.));
#15336=DIRECTION('',(-0.0785156880315736,0.996912878205979,0.));
#15337=DIRECTION('center_axis',(0.,0.,1.));
#15338=DIRECTION('ref_axis',(1.,0.,0.));
#15339=DIRECTION('center_axis',(0.,0.,1.));
#15340=DIRECTION('ref_axis',(1.,0.,0.));
#15341=DIRECTION('',(0.824094033870449,-0.566453019533952,0.));
#15342=DIRECTION('center_axis',(0.566453019533952,0.824094033870449,0.));
#15343=DIRECTION('ref_axis',(0.824094033870449,-0.566453019533952,0.));
#15344=DIRECTION('',(0.,0.,-1.));
#15345=DIRECTION('',(0.824094033870449,-0.566453019533952,0.));
#15346=DIRECTION('center_axis',(0.,0.,-1.));
#15347=DIRECTION('ref_axis',(-1.,0.,0.));
#15348=DIRECTION('center_axis',(0.,0.,-1.));
#15349=DIRECTION('ref_axis',(1.,0.,0.));
#15350=DIRECTION('center_axis',(-0.963645622090473,0.26718367282801,0.));
#15351=DIRECTION('ref_axis',(0.26718367282801,0.963645622090473,0.));
#15352=DIRECTION('',(0.,0.,1.));
#15353=DIRECTION('',(0.26718367282801,0.963645622090473,0.));
#15354=DIRECTION('',(0.,0.,-1.));
#15355=DIRECTION('',(0.26718367282801,0.963645622090473,0.));
#15356=DIRECTION('center_axis',(0.,0.,1.));
#15357=DIRECTION('ref_axis',(1.,0.,0.));
#15358=DIRECTION('center_axis',(0.,0.,1.));
#15359=DIRECTION('ref_axis',(1.,0.,0.));
#15360=DIRECTION('',(0.580656739533499,-0.814148482056146,0.));
#15361=DIRECTION('center_axis',(0.814148482056146,0.580656739533499,0.));
#15362=DIRECTION('ref_axis',(0.580656739533499,-0.814148482056146,0.));
#15363=DIRECTION('',(0.,0.,-1.));
#15364=DIRECTION('',(0.580656739533499,-0.814148482056146,0.));
#15365=DIRECTION('center_axis',(0.,0.,-1.));
#15366=DIRECTION('ref_axis',(-1.,0.,0.));
#15367=DIRECTION('center_axis',(0.,0.,-1.));
#15368=DIRECTION('ref_axis',(1.,0.,0.));
#15369=DIRECTION('center_axis',(-0.814148482056146,0.580656739533499,0.));
#15370=DIRECTION('ref_axis',(0.580656739533499,0.814148482056146,0.));
#15371=DIRECTION('',(0.,0.,1.));
#15372=DIRECTION('',(0.580656739533499,0.814148482056146,0.));
#15373=DIRECTION('',(0.,0.,-1.));
#15374=DIRECTION('',(0.580656739533499,0.814148482056146,0.));
#15375=DIRECTION('center_axis',(0.,0.,1.));
#15376=DIRECTION('ref_axis',(1.,0.,0.));
#15377=DIRECTION('center_axis',(0.,0.,1.));
#15378=DIRECTION('ref_axis',(1.,0.,0.));
#15379=DIRECTION('',(0.267183672828016,-0.963645622090472,0.));
#15380=DIRECTION('center_axis',(0.963645622090472,0.267183672828016,0.));
#15381=DIRECTION('ref_axis',(0.267183672828016,-0.963645622090472,0.));
#15382=DIRECTION('',(0.,0.,-1.));
#15383=DIRECTION('',(0.267183672828016,-0.963645622090472,0.));
#15384=DIRECTION('center_axis',(0.,0.,-1.));
#15385=DIRECTION('ref_axis',(-1.,0.,0.));
#15386=DIRECTION('center_axis',(0.,0.,-1.));
#15387=DIRECTION('ref_axis',(1.,0.,0.));
#15388=DIRECTION('center_axis',(-0.56645301953395,0.82409403387045,0.));
#15389=DIRECTION('ref_axis',(0.82409403387045,0.56645301953395,0.));
#15390=DIRECTION('',(0.,0.,1.));
#15391=DIRECTION('',(0.82409403387045,0.56645301953395,0.));
#15392=DIRECTION('',(0.,0.,-1.));
#15393=DIRECTION('',(0.82409403387045,0.56645301953395,0.));
#15394=DIRECTION('center_axis',(0.,0.,1.));
#15395=DIRECTION('ref_axis',(1.,0.,0.));
#15396=DIRECTION('center_axis',(0.,0.,1.));
#15397=DIRECTION('ref_axis',(1.,0.,0.));
#15398=DIRECTION('',(-0.0785156880315734,-0.996912878205979,0.));
#15399=DIRECTION('center_axis',(0.996912878205979,-0.0785156880315734,0.));
#15400=DIRECTION('ref_axis',(-0.0785156880315734,-0.996912878205979,0.));
#15401=DIRECTION('',(0.,0.,-1.));
#15402=DIRECTION('',(-0.0785156880315734,-0.996912878205979,0.));
#15403=DIRECTION('center_axis',(0.,0.,-1.));
#15404=DIRECTION('ref_axis',(-1.,0.,0.));
#15405=DIRECTION('center_axis',(0.,0.,-1.));
#15406=DIRECTION('ref_axis',(1.,0.,0.));
#15407=DIRECTION('center_axis',(-0.250434962899748,0.968133425390014,0.));
#15408=DIRECTION('ref_axis',(0.968133425390014,0.250434962899748,0.));
#15409=DIRECTION('',(0.,0.,1.));
#15410=DIRECTION('',(0.968133425390014,0.250434962899748,0.));
#15411=DIRECTION('',(0.,0.,-1.));
#15412=DIRECTION('',(0.968133425390014,0.250434962899748,0.));
#15413=DIRECTION('center_axis',(0.,0.,1.));
#15414=DIRECTION('ref_axis',(1.,0.,0.));
#15415=DIRECTION('center_axis',(0.,0.,1.));
#15416=DIRECTION('ref_axis',(1.,0.,0.));
#15417=DIRECTION('',(-0.414744898146415,-0.909937728342726,0.));
#15418=DIRECTION('center_axis',(0.909937728342726,-0.414744898146415,0.));
#15419=DIRECTION('ref_axis',(-0.414744898146415,-0.909937728342726,0.));
#15420=DIRECTION('',(0.,0.,-1.));
#15421=DIRECTION('',(-0.414744898146415,-0.909937728342726,0.));
#15422=DIRECTION('center_axis',(0.,0.,-1.));
#15423=DIRECTION('ref_axis',(-1.,0.,0.));
#15424=DIRECTION('center_axis',(0.,0.,-1.));
#15425=DIRECTION('ref_axis',(1.,0.,0.));
#15426=DIRECTION('center_axis',(0.0957892462865784,0.995401637679911,0.));
#15427=DIRECTION('ref_axis',(0.995401637679911,-0.0957892462865784,0.));
#15428=DIRECTION('',(0.,0.,1.));
#15429=DIRECTION('',(0.995401637679911,-0.0957892462865784,0.));
#15430=DIRECTION('',(0.,0.,-1.));
#15431=DIRECTION('',(0.995401637679911,-0.0957892462865784,0.));
#15432=DIRECTION('center_axis',(0.,0.,1.));
#15433=DIRECTION('ref_axis',(1.,0.,0.));
#15434=DIRECTION('center_axis',(0.,0.,1.));
#15435=DIRECTION('ref_axis',(1.,0.,0.));
#15436=DIRECTION('',(-0.700949752562001,-0.713210659190726,0.));
#15437=DIRECTION('center_axis',(0.713210659190726,-0.700949752562001,0.));
#15438=DIRECTION('ref_axis',(-0.700949752562001,-0.713210659190726,0.));
#15439=DIRECTION('',(0.,0.,-1.));
#15440=DIRECTION('',(-0.700949752562001,-0.713210659190726,0.));
#15441=DIRECTION('center_axis',(0.,0.,-1.));
#15442=DIRECTION('ref_axis',(-1.,0.,0.));
#15443=DIRECTION('center_axis',(0.,0.,-1.));
#15444=DIRECTION('ref_axis',(1.,0.,0.));
#15445=DIRECTION('center_axis',(0.43045985867203,0.902609721902028,0.));
#15446=DIRECTION('ref_axis',(0.902609721902028,-0.43045985867203,0.));
#15447=DIRECTION('',(0.,0.,1.));
#15448=DIRECTION('',(0.902609721902028,-0.43045985867203,0.));
#15449=DIRECTION('',(0.,0.,-1.));
#15450=DIRECTION('',(0.902609721902028,-0.43045985867203,0.));
#15451=DIRECTION('center_axis',(0.,0.,1.));
#15452=DIRECTION('ref_axis',(1.,0.,0.));
#15453=DIRECTION('center_axis',(0.,0.,1.));
#15454=DIRECTION('ref_axis',(1.,0.,0.));
#15455=DIRECTION('',(-0.902609721902028,-0.43045985867203,0.));
#15456=DIRECTION('center_axis',(0.,0.,1.));
#15457=DIRECTION('ref_axis',(1.,0.,0.));
#15458=DIRECTION('center_axis',(0.43045985867203,-0.902609721902028,0.));
#15459=DIRECTION('ref_axis',(-0.902609721902028,-0.43045985867203,0.));
#15460=DIRECTION('',(0.,0.,-1.));
#15461=DIRECTION('',(-0.902609721902028,-0.43045985867203,0.));
#15462=DIRECTION('center_axis',(0.,0.,-1.));
#15463=DIRECTION('ref_axis',(-1.,0.,0.));
#15464=DIRECTION('center_axis',(0.,0.,-1.));
#15465=DIRECTION('ref_axis',(1.,0.,0.));
#15466=DIRECTION('center_axis',(0.,0.,-1.));
#15467=DIRECTION('ref_axis',(1.,0.,0.));
#15468=DIRECTION('center_axis',(0.580656739533499,0.814148482056146,0.));
#15469=DIRECTION('ref_axis',(0.814148482056146,-0.580656739533499,0.));
#15470=DIRECTION('',(0.,0.,1.));
#15471=DIRECTION('',(0.814148482056146,-0.580656739533499,0.));
#15472=DIRECTION('',(0.,0.,-1.));
#15473=DIRECTION('',(0.814148482056146,-0.580656739533499,0.));
#15474=DIRECTION('center_axis',(0.,0.,1.));
#15475=DIRECTION('ref_axis',(1.,0.,0.));
#15476=DIRECTION('center_axis',(0.,0.,1.));
#15477=DIRECTION('ref_axis',(1.,0.,0.));
#15478=DIRECTION('',(-0.963645622090472,-0.267183672828013,0.));
#15479=DIRECTION('center_axis',(0.267183672828013,-0.963645622090472,0.));
#15480=DIRECTION('ref_axis',(-0.963645622090472,-0.267183672828013,0.));
#15481=DIRECTION('',(0.,0.,-1.));
#15482=DIRECTION('',(-0.963645622090472,-0.267183672828013,0.));
#15483=DIRECTION('center_axis',(0.,0.,-1.));
#15484=DIRECTION('ref_axis',(-1.,0.,0.));
#15485=DIRECTION('center_axis',(0.,0.,-1.));
#15486=DIRECTION('ref_axis',(1.,0.,0.));
#15487=DIRECTION('center_axis',(0.824094033870453,0.566453019533945,0.));
#15488=DIRECTION('ref_axis',(0.566453019533945,-0.824094033870453,0.));
#15489=DIRECTION('',(0.,0.,1.));
#15490=DIRECTION('',(0.566453019533945,-0.824094033870453,0.));
#15491=DIRECTION('',(0.,0.,-1.));
#15492=DIRECTION('',(0.566453019533945,-0.824094033870453,0.));
#15493=DIRECTION('center_axis',(0.,0.,1.));
#15494=DIRECTION('ref_axis',(1.,0.,0.));
#15495=DIRECTION('center_axis',(0.,0.,1.));
#15496=DIRECTION('ref_axis',(1.,0.,0.));
#15497=DIRECTION('',(-0.996912878205979,0.078515688031577,0.));
#15498=DIRECTION('center_axis',(-0.078515688031577,-0.996912878205979,0.));
#15499=DIRECTION('ref_axis',(-0.996912878205979,0.078515688031577,0.));
#15500=DIRECTION('',(0.,0.,-1.));
#15501=DIRECTION('',(-0.996912878205979,0.078515688031577,0.));
#15502=DIRECTION('center_axis',(0.,0.,-1.));
#15503=DIRECTION('ref_axis',(-1.,0.,0.));
#15504=DIRECTION('center_axis',(0.,0.,-1.));
#15505=DIRECTION('ref_axis',(1.,0.,0.));
#15506=DIRECTION('center_axis',(0.968133425390014,0.250434962899747,0.));
#15507=DIRECTION('ref_axis',(0.250434962899747,-0.968133425390014,0.));
#15508=DIRECTION('',(0.,0.,1.));
#15509=DIRECTION('',(0.250434962899747,-0.968133425390014,0.));
#15510=DIRECTION('',(0.,0.,-1.));
#15511=DIRECTION('',(0.250434962899747,-0.968133425390014,0.));
#15512=DIRECTION('center_axis',(0.,0.,1.));
#15513=DIRECTION('ref_axis',(1.,0.,0.));
#15514=DIRECTION('center_axis',(0.,0.,1.));
#15515=DIRECTION('ref_axis',(1.,0.,0.));
#15516=DIRECTION('',(-0.909937728342725,0.414744898146415,0.));
#15517=DIRECTION('center_axis',(-0.414744898146415,-0.909937728342725,0.));
#15518=DIRECTION('ref_axis',(-0.909937728342725,0.414744898146415,0.));
#15519=DIRECTION('',(0.,0.,-1.));
#15520=DIRECTION('',(-0.909937728342725,0.414744898146415,0.));
#15521=DIRECTION('center_axis',(0.,0.,-1.));
#15522=DIRECTION('ref_axis',(-1.,0.,0.));
#15523=DIRECTION('center_axis',(0.,0.,-1.));
#15524=DIRECTION('ref_axis',(1.,0.,0.));
#15525=DIRECTION('center_axis',(0.995401637679911,-0.0957892462865797,0.));
#15526=DIRECTION('ref_axis',(-0.0957892462865797,-0.995401637679911,0.));
#15527=DIRECTION('',(0.,0.,1.));
#15528=DIRECTION('',(-0.0957892462865797,-0.995401637679911,0.));
#15529=DIRECTION('',(0.,0.,-1.));
#15530=DIRECTION('',(-0.0957892462865797,-0.995401637679911,0.));
#15531=DIRECTION('center_axis',(0.,0.,1.));
#15532=DIRECTION('ref_axis',(1.,0.,0.));
#15533=DIRECTION('center_axis',(0.,0.,1.));
#15534=DIRECTION('ref_axis',(1.,0.,0.));
#15535=DIRECTION('',(-0.713210659190727,0.700949752562,0.));
#15536=DIRECTION('center_axis',(-0.700949752562,-0.713210659190727,0.));
#15537=DIRECTION('ref_axis',(-0.713210659190727,0.700949752562,0.));
#15538=DIRECTION('',(0.,0.,-1.));
#15539=DIRECTION('',(-0.713210659190727,0.700949752562,0.));
#15540=DIRECTION('center_axis',(0.,0.,-1.));
#15541=DIRECTION('ref_axis',(-1.,0.,0.));
#15542=DIRECTION('center_axis',(0.,0.,-1.));
#15543=DIRECTION('ref_axis',(1.,0.,0.));
#15544=DIRECTION('center_axis',(0.902609721902027,-0.430459858672031,0.));
#15545=DIRECTION('ref_axis',(-0.430459858672031,-0.902609721902027,0.));
#15546=DIRECTION('',(0.,0.,1.));
#15547=DIRECTION('',(-0.430459858672031,-0.902609721902027,0.));
#15548=DIRECTION('',(0.,0.,-1.));
#15549=DIRECTION('',(-0.430459858672031,-0.902609721902027,0.));
#15550=DIRECTION('center_axis',(0.,0.,1.));
#15551=DIRECTION('ref_axis',(1.,0.,0.));
#15552=DIRECTION('center_axis',(0.,0.,1.));
#15553=DIRECTION('ref_axis',(1.,0.,0.));
#15554=DIRECTION('',(-0.430459858672031,0.902609721902027,0.));
#15555=DIRECTION('center_axis',(-0.902609721902027,-0.430459858672031,0.));
#15556=DIRECTION('ref_axis',(-0.430459858672031,0.902609721902027,0.));
#15557=DIRECTION('',(0.,0.,-1.));
#15558=DIRECTION('',(-0.430459858672031,0.902609721902027,0.));
#15559=DIRECTION('center_axis',(0.,0.,-1.));
#15560=DIRECTION('ref_axis',(-1.,0.,0.));
#15561=DIRECTION('center_axis',(0.,0.,-1.));
#15562=DIRECTION('ref_axis',(1.,0.,0.));
#15563=DIRECTION('center_axis',(0.700949752562001,-0.713210659190726,0.));
#15564=DIRECTION('ref_axis',(-0.713210659190726,-0.700949752562001,0.));
#15565=DIRECTION('',(0.,0.,1.));
#15566=DIRECTION('',(-0.713210659190726,-0.700949752562001,0.));
#15567=DIRECTION('',(0.,0.,-1.));
#15568=DIRECTION('',(-0.713210659190726,-0.700949752562001,0.));
#15569=DIRECTION('center_axis',(0.,0.,1.));
#15570=DIRECTION('ref_axis',(1.,0.,0.));
#15571=DIRECTION('center_axis',(0.,0.,1.));
#15572=DIRECTION('ref_axis',(1.,0.,0.));
#15573=DIRECTION('',(-0.0957892462865797,0.995401637679911,0.));
#15574=DIRECTION('center_axis',(-0.995401637679911,-0.0957892462865797,
0.));
#15575=DIRECTION('ref_axis',(-0.0957892462865797,0.995401637679911,0.));
#15576=DIRECTION('',(0.,0.,-1.));
#15577=DIRECTION('',(-0.0957892462865797,0.995401637679911,0.));
#15578=DIRECTION('center_axis',(0.,0.,-1.));
#15579=DIRECTION('ref_axis',(-1.,0.,0.));
#15580=DIRECTION('center_axis',(0.,0.,-1.));
#15581=DIRECTION('ref_axis',(1.,0.,0.));
#15582=DIRECTION('center_axis',(0.414744898146414,-0.909937728342726,0.));
#15583=DIRECTION('ref_axis',(-0.909937728342726,-0.414744898146414,0.));
#15584=DIRECTION('',(0.,0.,1.));
#15585=DIRECTION('',(-0.909937728342726,-0.414744898146414,0.));
#15586=DIRECTION('',(0.,0.,-1.));
#15587=DIRECTION('',(-0.909937728342726,-0.414744898146414,0.));
#15588=DIRECTION('center_axis',(0.,0.,1.));
#15589=DIRECTION('ref_axis',(1.,0.,0.));
#15590=DIRECTION('center_axis',(0.,0.,1.));
#15591=DIRECTION('ref_axis',(1.,0.,0.));
#15592=DIRECTION('',(0.250434962899747,0.968133425390014,0.));
#15593=DIRECTION('center_axis',(-0.968133425390014,0.250434962899747,0.));
#15594=DIRECTION('ref_axis',(0.250434962899747,0.968133425390014,0.));
#15595=DIRECTION('',(0.,0.,-1.));
#15596=DIRECTION('',(0.250434962899747,0.968133425390014,0.));
#15597=DIRECTION('center_axis',(0.,0.,-1.));
#15598=DIRECTION('ref_axis',(-1.,0.,0.));
#15599=DIRECTION('center_axis',(0.,0.,-1.));
#15600=DIRECTION('ref_axis',(1.,0.,0.));
#15601=DIRECTION('center_axis',(0.078515688031576,-0.996912878205979,0.));
#15602=DIRECTION('ref_axis',(-0.996912878205979,-0.078515688031576,0.));
#15603=DIRECTION('',(0.,0.,1.));
#15604=DIRECTION('',(-0.996912878205979,-0.078515688031576,0.));
#15605=DIRECTION('',(0.,0.,-1.));
#15606=DIRECTION('',(-0.996912878205979,-0.078515688031576,0.));
#15607=DIRECTION('center_axis',(0.,0.,1.));
#15608=DIRECTION('ref_axis',(1.,0.,0.));
#15609=DIRECTION('center_axis',(0.,0.,1.));
#15610=DIRECTION('ref_axis',(1.,0.,0.));
#15611=DIRECTION('',(0.566453019533946,0.824094033870453,0.));
#15612=DIRECTION('center_axis',(-0.824094033870453,0.566453019533946,0.));
#15613=DIRECTION('ref_axis',(0.566453019533946,0.824094033870453,0.));
#15614=DIRECTION('',(0.,0.,-1.));
#15615=DIRECTION('',(0.566453019533946,0.824094033870453,0.));
#15616=DIRECTION('center_axis',(0.,0.,-1.));
#15617=DIRECTION('ref_axis',(-1.,0.,0.));
#15618=DIRECTION('center_axis',(0.,0.,-1.));
#15619=DIRECTION('ref_axis',(1.,0.,0.));
#15620=DIRECTION('center_axis',(-0.267183672828014,-0.963645622090472,0.));
#15621=DIRECTION('ref_axis',(-0.963645622090472,0.267183672828014,0.));
#15622=DIRECTION('',(0.,0.,1.));
#15623=DIRECTION('',(-0.963645622090472,0.267183672828014,0.));
#15624=DIRECTION('',(0.,0.,-1.));
#15625=DIRECTION('',(-0.963645622090472,0.267183672828014,0.));
#15626=DIRECTION('center_axis',(0.,0.,1.));
#15627=DIRECTION('ref_axis',(1.,0.,0.));
#15628=DIRECTION('center_axis',(0.,0.,1.));
#15629=DIRECTION('ref_axis',(1.,0.,0.));
#15630=DIRECTION('',(0.814148482056147,0.580656739533497,0.));
#15631=DIRECTION('center_axis',(-0.580656739533497,0.814148482056147,0.));
#15632=DIRECTION('ref_axis',(0.814148482056147,0.580656739533497,0.));
#15633=DIRECTION('',(0.,0.,-1.));
#15634=DIRECTION('',(0.814148482056147,0.580656739533497,0.));
#15635=DIRECTION('center_axis',(0.,0.,-1.));
#15636=DIRECTION('ref_axis',(-1.,0.,0.));
#15637=DIRECTION('center_axis',(0.,0.,-1.));
#15638=DIRECTION('ref_axis',(1.,0.,0.));
#15639=DIRECTION('center_axis',(-0.0957892462865788,-0.995401637679911,
0.));
#15640=DIRECTION('ref_axis',(-0.995401637679911,0.0957892462865788,0.));
#15641=DIRECTION('',(0.,0.,1.));
#15642=DIRECTION('',(-0.995401637679911,0.0957892462865788,0.));
#15643=DIRECTION('',(0.,0.,-1.));
#15644=DIRECTION('',(-0.995401637679911,0.0957892462865788,0.));
#15645=DIRECTION('center_axis',(0.,0.,1.));
#15646=DIRECTION('ref_axis',(1.,0.,0.));
#15647=DIRECTION('center_axis',(0.,0.,1.));
#15648=DIRECTION('ref_axis',(1.,0.,0.));
#15649=DIRECTION('',(0.700949752562,0.713210659190726,0.));
#15650=DIRECTION('center_axis',(-0.713210659190726,0.700949752562,0.));
#15651=DIRECTION('ref_axis',(0.700949752562,0.713210659190726,0.));
#15652=DIRECTION('',(0.,0.,-1.));
#15653=DIRECTION('',(0.700949752562,0.713210659190726,0.));
#15654=DIRECTION('center_axis',(0.,0.,-1.));
#15655=DIRECTION('ref_axis',(-1.,0.,0.));
#15656=DIRECTION('center_axis',(0.,0.,-1.));
#15657=DIRECTION('ref_axis',(1.,0.,0.));
#15658=DIRECTION('center_axis',(0.250434962899746,-0.968133425390014,0.));
#15659=DIRECTION('ref_axis',(-0.968133425390014,-0.250434962899746,0.));
#15660=DIRECTION('',(0.,0.,1.));
#15661=DIRECTION('',(-0.968133425390014,-0.250434962899746,0.));
#15662=DIRECTION('',(0.,0.,-1.));
#15663=DIRECTION('',(-0.968133425390014,-0.250434962899746,0.));
#15664=DIRECTION('center_axis',(0.,0.,1.));
#15665=DIRECTION('ref_axis',(1.,0.,0.));
#15666=DIRECTION('center_axis',(0.,0.,1.));
#15667=DIRECTION('ref_axis',(1.,0.,0.));
#15668=DIRECTION('',(0.414744898146414,0.909937728342726,0.));
#15669=DIRECTION('center_axis',(-0.909937728342726,0.414744898146414,0.));
#15670=DIRECTION('ref_axis',(0.414744898146414,0.909937728342726,0.));
#15671=DIRECTION('',(0.,0.,-1.));
#15672=DIRECTION('',(0.414744898146414,0.909937728342726,0.));
#15673=DIRECTION('center_axis',(0.,0.,-1.));
#15674=DIRECTION('ref_axis',(-1.,0.,0.));
#15675=DIRECTION('center_axis',(0.,0.,-1.));
#15676=DIRECTION('ref_axis',(1.,0.,0.));
#15677=DIRECTION('center_axis',(0.566453019533948,-0.824094033870452,0.));
#15678=DIRECTION('ref_axis',(-0.824094033870452,-0.566453019533948,0.));
#15679=DIRECTION('',(0.,0.,1.));
#15680=DIRECTION('',(-0.824094033870452,-0.566453019533948,0.));
#15681=DIRECTION('',(0.,0.,-1.));
#15682=DIRECTION('',(-0.824094033870452,-0.566453019533948,0.));
#15683=DIRECTION('center_axis',(0.,0.,1.));
#15684=DIRECTION('ref_axis',(1.,0.,0.));
#15685=DIRECTION('center_axis',(0.,0.,1.));
#15686=DIRECTION('ref_axis',(1.,0.,0.));
#15687=DIRECTION('',(0.0785156880315752,0.996912878205979,0.));
#15688=DIRECTION('center_axis',(-0.996912878205979,0.0785156880315752,0.));
#15689=DIRECTION('ref_axis',(0.0785156880315752,0.996912878205979,0.));
#15690=DIRECTION('',(0.,0.,-1.));
#15691=DIRECTION('',(0.0785156880315752,0.996912878205979,0.));
#15692=DIRECTION('center_axis',(0.,0.,-1.));
#15693=DIRECTION('ref_axis',(-1.,0.,0.));
#15694=DIRECTION('center_axis',(0.,0.,-1.));
#15695=DIRECTION('ref_axis',(1.,0.,0.));
#15696=DIRECTION('center_axis',(0.814148482056148,-0.580656739533496,0.));
#15697=DIRECTION('ref_axis',(-0.580656739533496,-0.814148482056148,0.));
#15698=DIRECTION('',(0.,0.,1.));
#15699=DIRECTION('',(-0.580656739533496,-0.814148482056148,0.));
#15700=DIRECTION('',(0.,0.,-1.));
#15701=DIRECTION('',(-0.580656739533496,-0.814148482056148,0.));
#15702=DIRECTION('center_axis',(0.,0.,1.));
#15703=DIRECTION('ref_axis',(1.,0.,0.));
#15704=DIRECTION('center_axis',(0.,0.,1.));
#15705=DIRECTION('ref_axis',(1.,0.,0.));
#15706=DIRECTION('',(-0.267183672828014,0.963645622090472,0.));
#15707=DIRECTION('center_axis',(-0.963645622090472,-0.267183672828014,0.));
#15708=DIRECTION('ref_axis',(-0.267183672828014,0.963645622090472,0.));
#15709=DIRECTION('',(0.,0.,-1.));
#15710=DIRECTION('',(-0.267183672828014,0.963645622090472,0.));
#15711=DIRECTION('center_axis',(0.,0.,-1.));
#15712=DIRECTION('ref_axis',(-1.,0.,0.));
#15713=DIRECTION('center_axis',(0.,0.,-1.));
#15714=DIRECTION('ref_axis',(1.,0.,0.));
#15715=DIRECTION('center_axis',(0.963645622090472,-0.267183672828014,0.));
#15716=DIRECTION('ref_axis',(-0.267183672828014,-0.963645622090472,0.));
#15717=DIRECTION('',(0.,0.,1.));
#15718=DIRECTION('',(-0.267183672828014,-0.963645622090472,0.));
#15719=DIRECTION('',(0.,0.,-1.));
#15720=DIRECTION('',(-0.267183672828014,-0.963645622090472,0.));
#15721=DIRECTION('center_axis',(0.,0.,1.));
#15722=DIRECTION('ref_axis',(1.,0.,0.));
#15723=DIRECTION('center_axis',(0.,0.,1.));
#15724=DIRECTION('ref_axis',(1.,0.,0.));
#15725=DIRECTION('',(-0.580656739533497,0.814148482056147,0.));
#15726=DIRECTION('center_axis',(-0.814148482056147,-0.580656739533497,0.));
#15727=DIRECTION('ref_axis',(-0.580656739533497,0.814148482056147,0.));
#15728=DIRECTION('',(0.,0.,-1.));
#15729=DIRECTION('',(-0.580656739533497,0.814148482056147,0.));
#15730=DIRECTION('center_axis',(0.,0.,-1.));
#15731=DIRECTION('ref_axis',(-1.,0.,0.));
#15732=DIRECTION('center_axis',(0.,0.,-1.));
#15733=DIRECTION('ref_axis',(1.,0.,0.));
#15734=DIRECTION('center_axis',(0.996912878205979,0.078515688031576,0.));
#15735=DIRECTION('ref_axis',(0.078515688031576,-0.996912878205979,0.));
#15736=DIRECTION('',(0.,0.,1.));
#15737=DIRECTION('',(0.078515688031576,-0.996912878205979,0.));
#15738=DIRECTION('',(0.,0.,-1.));
#15739=DIRECTION('',(0.078515688031576,-0.996912878205979,0.));
#15740=DIRECTION('center_axis',(0.,0.,1.));
#15741=DIRECTION('ref_axis',(1.,0.,0.));
#15742=DIRECTION('center_axis',(0.,0.,1.));
#15743=DIRECTION('ref_axis',(1.,0.,0.));
#15744=DIRECTION('',(-0.824094033870453,0.566453019533946,0.));
#15745=DIRECTION('center_axis',(-0.566453019533946,-0.824094033870453,0.));
#15746=DIRECTION('ref_axis',(-0.824094033870453,0.566453019533946,0.));
#15747=DIRECTION('',(0.,0.,-1.));
#15748=DIRECTION('',(-0.824094033870453,0.566453019533946,0.));
#15749=DIRECTION('center_axis',(0.,0.,-1.));
#15750=DIRECTION('ref_axis',(-1.,0.,0.));
#15751=DIRECTION('center_axis',(0.,0.,-1.));
#15752=DIRECTION('ref_axis',(1.,0.,0.));
#15753=DIRECTION('center_axis',(0.909937728342726,0.414744898146415,0.));
#15754=DIRECTION('ref_axis',(0.414744898146415,-0.909937728342726,0.));
#15755=DIRECTION('',(0.,0.,1.));
#15756=DIRECTION('',(0.414744898146415,-0.909937728342726,0.));
#15757=DIRECTION('',(0.,0.,-1.));
#15758=DIRECTION('',(0.414744898146415,-0.909937728342726,0.));
#15759=DIRECTION('center_axis',(0.,0.,1.));
#15760=DIRECTION('ref_axis',(1.,0.,0.));
#15761=DIRECTION('center_axis',(0.,0.,1.));
#15762=DIRECTION('ref_axis',(1.,0.,0.));
#15763=DIRECTION('',(-0.968133425390015,0.250434962899744,0.));
#15764=DIRECTION('center_axis',(-0.250434962899744,-0.968133425390015,0.));
#15765=DIRECTION('ref_axis',(-0.968133425390015,0.250434962899744,0.));
#15766=DIRECTION('',(0.,0.,-1.));
#15767=DIRECTION('',(-0.968133425390015,0.250434962899744,0.));
#15768=DIRECTION('center_axis',(0.,0.,-1.));
#15769=DIRECTION('ref_axis',(-1.,0.,0.));
#15770=DIRECTION('center_axis',(0.,0.,-1.));
#15771=DIRECTION('ref_axis',(1.,0.,0.));
#15772=DIRECTION('center_axis',(0.713210659190726,0.700949752562001,0.));
#15773=DIRECTION('ref_axis',(0.700949752562001,-0.713210659190726,0.));
#15774=DIRECTION('',(0.,0.,1.));
#15775=DIRECTION('',(0.700949752562001,-0.713210659190726,0.));
#15776=DIRECTION('',(0.,0.,-1.));
#15777=DIRECTION('',(0.700949752562001,-0.713210659190726,0.));
#15778=DIRECTION('center_axis',(0.,0.,1.));
#15779=DIRECTION('ref_axis',(1.,0.,0.));
#15780=DIRECTION('center_axis',(0.,0.,1.));
#15781=DIRECTION('ref_axis',(1.,0.,0.));
#15782=DIRECTION('',(-0.995401637679911,-0.0957892462865814,0.));
#15783=DIRECTION('center_axis',(0.0957892462865814,-0.995401637679911,0.));
#15784=DIRECTION('ref_axis',(-0.995401637679911,-0.0957892462865814,0.));
#15785=DIRECTION('',(0.,0.,-1.));
#15786=DIRECTION('',(-0.995401637679911,-0.0957892462865814,0.));
#15787=DIRECTION('center_axis',(0.,0.,-1.));
#15788=DIRECTION('ref_axis',(-1.,0.,0.));
#15789=DIRECTION('center_axis',(0.,0.,-1.));
#15790=DIRECTION('ref_axis',(1.,0.,0.));
#15791=DIRECTION('center_axis',(0.,0.,1.));
#15792=DIRECTION('ref_axis',(1.,0.,0.));
#15793=DIRECTION('center_axis',(0.,0.,1.));
#15794=DIRECTION('ref_axis',(1.,0.,0.));
#15795=DIRECTION('',(-0.902609721902027,0.430459858672031,0.));
#15796=DIRECTION('',(0.902609721902027,0.430459858672031,0.));
#15797=DIRECTION('center_axis',(-0.430459858672031,-0.902609721902027,0.));
#15798=DIRECTION('ref_axis',(-0.902609721902027,0.430459858672031,0.));
#15799=DIRECTION('',(0.,0.,1.));
#15800=DIRECTION('',(-0.902609721902027,0.430459858672031,0.));
#15801=DIRECTION('',(0.,0.,-1.));
#15802=DIRECTION('center_axis',(-0.430459858672031,0.902609721902027,0.));
#15803=DIRECTION('ref_axis',(0.902609721902027,0.430459858672031,0.));
#15804=DIRECTION('',(0.,0.,-1.));
#15805=DIRECTION('',(0.902609721902027,0.430459858672031,0.));
#15806=DIRECTION('center_axis',(0.,0.,-1.));
#15807=DIRECTION('ref_axis',(-1.,0.,0.));
#15808=DIRECTION('center_axis',(0.,0.,-1.));
#15809=DIRECTION('ref_axis',(1.,0.,0.));
#15810=DIRECTION('center_axis',(0.267183672828015,0.963645622090472,0.));
#15811=DIRECTION('ref_axis',(0.963645622090472,-0.267183672828015,0.));
#15812=DIRECTION('',(0.,0.,1.));
#15813=DIRECTION('',(0.963645622090472,-0.267183672828015,0.));
#15814=DIRECTION('',(0.,0.,-1.));
#15815=DIRECTION('',(0.963645622090472,-0.267183672828015,0.));
#15816=DIRECTION('center_axis',(0.,0.,1.));
#15817=DIRECTION('ref_axis',(1.,0.,0.));
#15818=DIRECTION('center_axis',(0.,0.,1.));
#15819=DIRECTION('ref_axis',(1.,0.,0.));
#15820=DIRECTION('',(-0.814148482056148,-0.580656739533496,0.));
#15821=DIRECTION('center_axis',(0.580656739533496,-0.814148482056148,0.));
#15822=DIRECTION('ref_axis',(-0.814148482056148,-0.580656739533496,0.));
#15823=DIRECTION('',(0.,0.,-1.));
#15824=DIRECTION('',(-0.814148482056148,-0.580656739533496,0.));
#15825=DIRECTION('center_axis',(0.,0.,-1.));
#15826=DIRECTION('ref_axis',(-1.,0.,0.));
#15827=DIRECTION('center_axis',(0.,0.,-1.));
#15828=DIRECTION('ref_axis',(1.,0.,0.));
#15829=DIRECTION('center_axis',(-0.0785156880315738,0.996912878205979,0.));
#15830=DIRECTION('ref_axis',(0.996912878205979,0.0785156880315738,0.));
#15831=DIRECTION('',(0.,0.,1.));
#15832=DIRECTION('',(0.996912878205979,0.0785156880315738,0.));
#15833=DIRECTION('',(0.,0.,-1.));
#15834=DIRECTION('',(0.996912878205979,0.0785156880315738,0.));
#15835=DIRECTION('center_axis',(0.,0.,1.));
#15836=DIRECTION('ref_axis',(1.,0.,0.));
#15837=DIRECTION('center_axis',(0.,0.,1.));
#15838=DIRECTION('ref_axis',(1.,0.,0.));
#15839=DIRECTION('',(-0.566453019533948,-0.824094033870452,0.));
#15840=DIRECTION('center_axis',(0.824094033870452,-0.566453019533948,0.));
#15841=DIRECTION('ref_axis',(-0.566453019533948,-0.824094033870452,0.));
#15842=DIRECTION('',(0.,0.,-1.));
#15843=DIRECTION('',(-0.566453019533948,-0.824094033870452,0.));
#15844=DIRECTION('center_axis',(0.,0.,-1.));
#15845=DIRECTION('ref_axis',(-1.,0.,0.));
#15846=DIRECTION('center_axis',(0.,0.,-1.));
#15847=DIRECTION('ref_axis',(1.,0.,0.));
#15848=DIRECTION('center_axis',(-0.414744898146415,0.909937728342726,0.));
#15849=DIRECTION('ref_axis',(0.909937728342726,0.414744898146415,0.));
#15850=DIRECTION('',(0.,0.,1.));
#15851=DIRECTION('',(0.909937728342726,0.414744898146415,0.));
#15852=DIRECTION('',(0.,0.,-1.));
#15853=DIRECTION('',(0.909937728342726,0.414744898146415,0.));
#15854=DIRECTION('center_axis',(0.,0.,1.));
#15855=DIRECTION('ref_axis',(1.,0.,0.));
#15856=DIRECTION('center_axis',(0.,0.,1.));
#15857=DIRECTION('ref_axis',(1.,0.,0.));
#15858=DIRECTION('',(-0.250434962899745,-0.968133425390015,0.));
#15859=DIRECTION('center_axis',(0.968133425390015,-0.250434962899745,0.));
#15860=DIRECTION('ref_axis',(-0.250434962899745,-0.968133425390015,0.));
#15861=DIRECTION('',(0.,0.,-1.));
#15862=DIRECTION('',(-0.250434962899745,-0.968133425390015,0.));
#15863=DIRECTION('center_axis',(0.,0.,-1.));
#15864=DIRECTION('ref_axis',(-1.,0.,0.));
#15865=DIRECTION('center_axis',(0.,0.,-1.));
#15866=DIRECTION('ref_axis',(1.,0.,0.));
#15867=DIRECTION('center_axis',(-0.700949752561999,0.713210659190727,0.));
#15868=DIRECTION('ref_axis',(0.713210659190727,0.700949752561999,0.));
#15869=DIRECTION('',(0.,0.,1.));
#15870=DIRECTION('',(0.713210659190727,0.700949752561999,0.));
#15871=DIRECTION('',(0.,0.,-1.));
#15872=DIRECTION('',(0.713210659190727,0.700949752561999,0.));
#15873=DIRECTION('center_axis',(0.,0.,1.));
#15874=DIRECTION('ref_axis',(1.,0.,0.));
#15875=DIRECTION('center_axis',(0.,0.,1.));
#15876=DIRECTION('ref_axis',(1.,0.,0.));
#15877=DIRECTION('',(0.0957892462865748,-0.995401637679912,0.));
#15878=DIRECTION('center_axis',(0.995401637679912,0.0957892462865748,0.));
#15879=DIRECTION('ref_axis',(0.0957892462865748,-0.995401637679912,0.));
#15880=DIRECTION('',(0.,0.,-1.));
#15881=DIRECTION('',(0.0957892462865748,-0.995401637679912,0.));
#15882=DIRECTION('center_axis',(0.,0.,-1.));
#15883=DIRECTION('ref_axis',(-1.,0.,0.));
#15884=DIRECTION('center_axis',(0.,0.,-1.));
#15885=DIRECTION('ref_axis',(1.,0.,0.));
#15886=DIRECTION('center_axis',(-0.902609721902026,0.430459858672033,0.));
#15887=DIRECTION('ref_axis',(0.430459858672033,0.902609721902026,0.));
#15888=DIRECTION('',(0.,0.,1.));
#15889=DIRECTION('',(0.430459858672033,0.902609721902026,0.));
#15890=DIRECTION('',(0.,0.,-1.));
#15891=DIRECTION('',(0.430459858672033,0.902609721902026,0.));
#15892=DIRECTION('center_axis',(0.,0.,1.));
#15893=DIRECTION('ref_axis',(1.,0.,0.));
#15894=DIRECTION('center_axis',(0.,0.,1.));
#15895=DIRECTION('ref_axis',(1.,0.,0.));
#15896=DIRECTION('',(0.430459858672033,-0.902609721902027,0.));
#15897=DIRECTION('center_axis',(0.902609721902027,0.430459858672033,0.));
#15898=DIRECTION('ref_axis',(0.430459858672033,-0.902609721902027,0.));
#15899=DIRECTION('',(0.,0.,-1.));
#15900=DIRECTION('',(0.430459858672033,-0.902609721902027,0.));
#15901=DIRECTION('center_axis',(0.,0.,-1.));
#15902=DIRECTION('ref_axis',(-1.,0.,0.));
#15903=DIRECTION('center_axis',(0.,0.,-1.));
#15904=DIRECTION('ref_axis',(1.,0.,0.));
#15905=DIRECTION('center_axis',(-0.995401637679911,0.0957892462865809,0.));
#15906=DIRECTION('ref_axis',(0.0957892462865809,0.995401637679911,0.));
#15907=DIRECTION('',(0.,0.,1.));
#15908=DIRECTION('',(0.0957892462865809,0.995401637679911,0.));
#15909=DIRECTION('',(0.,0.,-1.));
#15910=DIRECTION('',(0.0957892462865809,0.995401637679911,0.));
#15911=DIRECTION('center_axis',(0.,0.,1.));
#15912=DIRECTION('ref_axis',(1.,0.,0.));
#15913=DIRECTION('center_axis',(0.,0.,1.));
#15914=DIRECTION('ref_axis',(1.,0.,0.));
#15915=DIRECTION('',(0.713210659190723,-0.700949752562004,0.));
#15916=DIRECTION('center_axis',(0.700949752562004,0.713210659190723,0.));
#15917=DIRECTION('ref_axis',(0.713210659190723,-0.700949752562004,0.));
#15918=DIRECTION('',(0.,0.,-1.));
#15919=DIRECTION('',(0.713210659190723,-0.700949752562004,0.));
#15920=DIRECTION('center_axis',(0.,0.,-1.));
#15921=DIRECTION('ref_axis',(-1.,0.,0.));
#15922=DIRECTION('center_axis',(0.,0.,-1.));
#15923=DIRECTION('ref_axis',(1.,0.,0.));
#15924=DIRECTION('center_axis',(-0.968133425390015,-0.250434962899744,0.));
#15925=DIRECTION('ref_axis',(-0.250434962899744,0.968133425390015,0.));
#15926=DIRECTION('',(0.,0.,1.));
#15927=DIRECTION('',(-0.250434962899744,0.968133425390015,0.));
#15928=DIRECTION('',(0.,0.,-1.));
#15929=DIRECTION('',(-0.250434962899744,0.968133425390015,0.));
#15930=DIRECTION('center_axis',(0.,0.,1.));
#15931=DIRECTION('ref_axis',(1.,0.,0.));
#15932=DIRECTION('center_axis',(0.,0.,1.));
#15933=DIRECTION('ref_axis',(1.,0.,0.));
#15934=DIRECTION('',(0.909937728342727,-0.414744898146412,0.));
#15935=DIRECTION('center_axis',(0.414744898146412,0.909937728342727,0.));
#15936=DIRECTION('ref_axis',(0.909937728342727,-0.414744898146412,0.));
#15937=DIRECTION('',(0.,0.,-1.));
#15938=DIRECTION('',(0.909937728342727,-0.414744898146412,0.));
#15939=DIRECTION('center_axis',(0.,0.,-1.));
#15940=DIRECTION('ref_axis',(-1.,0.,0.));
#15941=DIRECTION('center_axis',(0.,0.,-1.));
#15942=DIRECTION('ref_axis',(1.,0.,0.));
#15943=DIRECTION('center_axis',(-0.82409403387045,-0.56645301953395,0.));
#15944=DIRECTION('ref_axis',(-0.56645301953395,0.82409403387045,0.));
#15945=DIRECTION('',(0.,0.,1.));
#15946=DIRECTION('',(-0.56645301953395,0.82409403387045,0.));
#15947=DIRECTION('',(0.,0.,-1.));
#15948=DIRECTION('',(-0.56645301953395,0.82409403387045,0.));
#15949=DIRECTION('center_axis',(0.,0.,1.));
#15950=DIRECTION('ref_axis',(1.,0.,0.));
#15951=DIRECTION('center_axis',(0.,0.,1.));
#15952=DIRECTION('ref_axis',(1.,0.,0.));
#15953=DIRECTION('',(0.996912878205979,-0.0785156880315738,0.));
#15954=DIRECTION('center_axis',(0.0785156880315738,0.996912878205979,0.));
#15955=DIRECTION('ref_axis',(0.996912878205979,-0.0785156880315738,0.));
#15956=DIRECTION('',(0.,0.,-1.));
#15957=DIRECTION('',(0.996912878205979,-0.0785156880315738,0.));
#15958=DIRECTION('center_axis',(0.,0.,-1.));
#15959=DIRECTION('ref_axis',(-1.,0.,0.));
#15960=DIRECTION('center_axis',(0.,0.,-1.));
#15961=DIRECTION('ref_axis',(1.,0.,0.));
#15962=DIRECTION('center_axis',(-0.580656739533499,-0.814148482056146,0.));
#15963=DIRECTION('ref_axis',(-0.814148482056146,0.580656739533499,0.));
#15964=DIRECTION('',(0.,0.,1.));
#15965=DIRECTION('',(-0.814148482056146,0.580656739533499,0.));
#15966=DIRECTION('',(0.,0.,-1.));
#15967=DIRECTION('',(-0.814148482056146,0.580656739533499,0.));
#15968=DIRECTION('center_axis',(0.,0.,1.));
#15969=DIRECTION('ref_axis',(1.,0.,0.));
#15970=DIRECTION('center_axis',(0.,0.,1.));
#15971=DIRECTION('ref_axis',(1.,0.,0.));
#15972=DIRECTION('',(0.963645622090472,0.267183672828016,0.));
#15973=DIRECTION('center_axis',(-0.267183672828016,0.963645622090472,0.));
#15974=DIRECTION('ref_axis',(0.963645622090472,0.267183672828016,0.));
#15975=DIRECTION('',(0.,0.,-1.));
#15976=DIRECTION('',(0.963645622090472,0.267183672828016,0.));
#15977=DIRECTION('center_axis',(0.,0.,-1.));
#15978=DIRECTION('ref_axis',(-1.,0.,0.));
#15979=DIRECTION('center_axis',(0.,0.,-1.));
#15980=DIRECTION('ref_axis',(1.,0.,0.));
#15981=DIRECTION('center_axis',(0.,0.,1.));
#15982=DIRECTION('ref_axis',(1.,0.,0.));
#15983=DIRECTION('center_axis',(0.,0.,1.));
#15984=DIRECTION('ref_axis',(-1.,1.22464679914735E-16,0.));
#15985=DIRECTION('center_axis',(1.22464679914735E-16,-1.,0.));
#15986=DIRECTION('ref_axis',(-1.,-1.22464679914735E-16,0.));
#15987=DIRECTION('center_axis',(0.,0.,-1.));
#15988=DIRECTION('ref_axis',(-1.,1.22464679914735E-16,0.));
#15989=DIRECTION('center_axis',(0.,0.,1.));
#15990=DIRECTION('ref_axis',(1.,0.,0.));
#15991=DIRECTION('',(0.,0.,-1.));
#15992=DIRECTION('center_axis',(0.,0.,1.));
#15993=DIRECTION('ref_axis',(1.,0.,0.));
#15994=DIRECTION('center_axis',(0.,0.,-1.));
#15995=DIRECTION('ref_axis',(-1.,0.,0.));
#15996=DIRECTION('center_axis',(0.,0.,1.));
#15997=DIRECTION('ref_axis',(1.,0.,0.));
#15998=DIRECTION('center_axis',(0.,0.,-1.));
#15999=DIRECTION('ref_axis',(-1.,0.,0.));
#16000=DIRECTION('center_axis',(0.,0.,1.));
#16001=DIRECTION('ref_axis',(1.,0.,0.));
#16002=DIRECTION('center_axis',(0.,0.,1.));
#16003=DIRECTION('ref_axis',(1.,0.,0.));
#16004=DIRECTION('',(0.707106781186547,8.65956056235493E-17,-0.707106781186548));
#16005=DIRECTION('center_axis',(0.,0.,1.));
#16006=DIRECTION('ref_axis',(1.,0.,0.));
#16007=DIRECTION('center_axis',(0.,0.,-1.));
#16008=DIRECTION('ref_axis',(1.,0.,0.));
#16009=DIRECTION('center_axis',(0.,0.,1.));
#16010=DIRECTION('ref_axis',(1.,0.,0.));
#16011=DIRECTION('center_axis',(0.,0.,1.));
#16012=DIRECTION('ref_axis',(1.,0.,0.));
#16013=DIRECTION('center_axis',(0.,0.,1.));
#16014=DIRECTION('ref_axis',(1.,0.,0.));
#16015=DIRECTION('',(0.707106781186548,8.65956056235494E-17,-0.707106781186547));
#16016=DIRECTION('center_axis',(0.,0.,1.));
#16017=DIRECTION('ref_axis',(1.,0.,0.));
#16018=DIRECTION('center_axis',(0.,0.,1.));
#16019=DIRECTION('ref_axis',(1.,0.,0.));
#16020=DIRECTION('center_axis',(0.,0.,1.));
#16021=DIRECTION('ref_axis',(1.,0.,0.));
#16022=DIRECTION('center_axis',(0.,0.,1.));
#16023=DIRECTION('ref_axis',(1.,0.,0.));
#16024=DIRECTION('center_axis',(0.,0.,1.));
#16025=DIRECTION('ref_axis',(1.,0.,0.));
#16026=DIRECTION('center_axis',(0.,0.,1.));
#16027=DIRECTION('ref_axis',(1.,0.,0.));
#16028=DIRECTION('center_axis',(0.,0.,1.));
#16029=DIRECTION('ref_axis',(1.,0.,0.));
#16030=DIRECTION('center_axis',(0.,0.,1.));
#16031=DIRECTION('ref_axis',(1.,0.,0.));
#16032=DIRECTION('center_axis',(0.,0.,1.));
#16033=DIRECTION('ref_axis',(1.,0.,0.));
#16034=DIRECTION('center_axis',(0.,0.,1.));
#16035=DIRECTION('ref_axis',(1.,0.,0.));
#16036=DIRECTION('center_axis',(0.,0.,1.));
#16037=DIRECTION('ref_axis',(1.,0.,0.));
#16038=DIRECTION('center_axis',(0.,0.,1.));
#16039=DIRECTION('ref_axis',(1.,0.,0.));
#16040=DIRECTION('center_axis',(0.,0.,1.));
#16041=DIRECTION('ref_axis',(1.,0.,0.));
#16042=DIRECTION('center_axis',(0.,0.,1.));
#16043=DIRECTION('ref_axis',(1.,0.,0.));
#16044=DIRECTION('center_axis',(0.,0.,1.));
#16045=DIRECTION('ref_axis',(1.,0.,0.));
#16046=DIRECTION('center_axis',(0.,0.,1.));
#16047=DIRECTION('ref_axis',(1.,0.,0.));
#16048=DIRECTION('center_axis',(0.,0.,1.));
#16049=DIRECTION('ref_axis',(1.,0.,0.));
#16050=DIRECTION('',(0.,0.,-1.));
#16051=DIRECTION('center_axis',(0.,0.,1.));
#16052=DIRECTION('ref_axis',(1.,0.,0.));
#16053=DIRECTION('center_axis',(0.,0.,1.));
#16054=DIRECTION('ref_axis',(1.,0.,0.));
#16055=DIRECTION('center_axis',(0.,0.,1.));
#16056=DIRECTION('ref_axis',(1.,0.,0.));
#16057=DIRECTION('center_axis',(0.,0.,1.));
#16058=DIRECTION('ref_axis',(1.,0.,0.));
#16059=DIRECTION('center_axis',(0.,0.,1.));
#16060=DIRECTION('ref_axis',(1.,0.,0.));
#16061=DIRECTION('center_axis',(0.,0.,1.));
#16062=DIRECTION('ref_axis',(1.,0.,0.));
#16063=DIRECTION('center_axis',(0.,0.,1.));
#16064=DIRECTION('ref_axis',(1.,0.,0.));
#16065=DIRECTION('center_axis',(0.,0.,1.));
#16066=DIRECTION('ref_axis',(1.,0.,0.));
#16067=DIRECTION('center_axis',(0.,0.,1.));
#16068=DIRECTION('ref_axis',(1.,0.,0.));
#16069=DIRECTION('center_axis',(0.,0.,1.));
#16070=DIRECTION('ref_axis',(1.,0.,0.));
#16071=DIRECTION('center_axis',(0.,0.,1.));
#16072=DIRECTION('ref_axis',(1.,0.,0.));
#16073=DIRECTION('center_axis',(0.,0.,1.));
#16074=DIRECTION('ref_axis',(1.,0.,0.));
#16075=DIRECTION('center_axis',(0.,0.,1.));
#16076=DIRECTION('ref_axis',(1.,0.,0.));
#16077=DIRECTION('center_axis',(0.,0.,1.));
#16078=DIRECTION('ref_axis',(1.,0.,0.));
#16079=DIRECTION('center_axis',(0.,0.,1.));
#16080=DIRECTION('ref_axis',(1.,0.,0.));
#16081=DIRECTION('center_axis',(0.,0.,1.));
#16082=DIRECTION('ref_axis',(1.,0.,0.));
#16083=DIRECTION('center_axis',(0.,0.,1.));
#16084=DIRECTION('ref_axis',(1.,0.,0.));
#16085=DIRECTION('center_axis',(0.,0.,1.));
#16086=DIRECTION('ref_axis',(1.,0.,0.));
#16087=DIRECTION('center_axis',(0.,0.,1.));
#16088=DIRECTION('ref_axis',(1.,0.,0.));
#16089=DIRECTION('center_axis',(0.,0.,1.));
#16090=DIRECTION('ref_axis',(1.,0.,0.));
#16091=DIRECTION('center_axis',(0.,0.,-1.));
#16092=DIRECTION('ref_axis',(1.,0.,0.));
#16093=DIRECTION('center_axis',(0.,0.,1.));
#16094=DIRECTION('ref_axis',(1.,0.,0.));
#16095=DIRECTION('',(-0.707106781186547,-8.65956056235493E-17,-0.707106781186547));
#16096=DIRECTION('center_axis',(0.,0.,1.));
#16097=DIRECTION('ref_axis',(1.,0.,0.));
#26908=CARTESIAN_POINT('',(0.,0.,0.));
#26909=CARTESIAN_POINT('Origin',(0.,0.,-4.78));
#26910=CARTESIAN_POINT('',(-0.294559949103625,0.000186743463070703,-5.93358238829104));
#26911=CARTESIAN_POINT('',(-0.294471258456466,0.000304903072910924,-5.94801761170896));
#26912=CARTESIAN_POINT('',(-0.2942,-3.60291088309151E-17,-4.78));
#26913=CARTESIAN_POINT('',(0.129048198622908,0.264655422342712,-5.9658));
#26914=CARTESIAN_POINT('Ctrl Pts',(-0.294559949103625,0.000186743463070703,
-5.93358238829104));
#26915=CARTESIAN_POINT('Ctrl Pts',(-0.294627032470039,0.0100023901992575,
-5.93411527799486));
#26916=CARTESIAN_POINT('Ctrl Pts',(-0.294179137669504,0.0198114650280941,
-5.93464816769869));
#26917=CARTESIAN_POINT('Ctrl Pts',(-0.293196168851624,0.0295661465485133,
-5.93518105740251));
#26918=CARTESIAN_POINT('Ctrl Pts',(-0.283428647221269,0.126496039964018,
-5.94047625254401));
#26919=CARTESIAN_POINT('Ctrl Pts',(-0.22082838450258,0.218055185618655,
-5.94577144768552));
#26920=CARTESIAN_POINT('Ctrl Pts',(-0.134050591616501,0.262404015513014,
-5.95106664282702));
#26921=CARTESIAN_POINT('Ctrl Pts',(-0.0535670473776308,0.303536094286101,
-5.95597776188468));
#26922=CARTESIAN_POINT('Ctrl Pts',(0.0477138908823457,0.304058088740004,
-5.96088888094234));
#26923=CARTESIAN_POINT('Ctrl Pts',(0.129204211840496,0.264848286765706,
-5.9658));
#26924=CARTESIAN_POINT('',(-0.128892185405324,0.264462557919717,-5.9658));
#26925=CARTESIAN_POINT('Origin',(0.,0.,-5.9658));
#26926=CARTESIAN_POINT('Ctrl Pts',(-0.128892185405323,0.264462557919717,
-5.9658));
#26927=CARTESIAN_POINT('Ctrl Pts',(-0.216880709330539,0.22157923549964,
-5.9605048048585));
#26928=CARTESIAN_POINT('Ctrl Pts',(-0.281018683526877,0.131692775518941,
-5.955209609717));
#26929=CARTESIAN_POINT('Ctrl Pts',(-0.292556379756586,0.0351079458526411,
-5.94991441457549));
#26930=CARTESIAN_POINT('Ctrl Pts',(-0.293934027145516,0.0235753282701674,
-5.94928214695332));
#26931=CARTESIAN_POINT('Ctrl Pts',(-0.294561735455353,0.0119472098769066,
-5.94864987933114));
#26932=CARTESIAN_POINT('Ctrl Pts',(-0.294471258456466,0.000304903072910924,
-5.94801761170896));
#26933=CARTESIAN_POINT('Origin',(0.,0.,-4.78));
#26934=CARTESIAN_POINT('',(-0.29380273100684,0.000158508790185821,-5.83358238829104));
#26935=CARTESIAN_POINT('',(-0.293774534382448,0.000134529535736241,-5.84801761170896));
#26936=CARTESIAN_POINT('',(-0.2942,-3.60291088309151E-17,-4.78));
#26937=CARTESIAN_POINT('Ctrl Pts',(-0.29380273100684,0.000158508790185821,
-5.83358238829104));
#26938=CARTESIAN_POINT('Ctrl Pts',(-0.293992111209095,0.0390074262588899,
-5.83567744047919));
#26939=CARTESIAN_POINT('Ctrl Pts',(-0.2868348483379,0.0777893022419187,
-5.83777249266733));
#26940=CARTESIAN_POINT('Ctrl Pts',(-0.272003615906625,0.11337249089091,
-5.83986754485547));
#26941=CARTESIAN_POINT('Ctrl Pts',(-0.234518024685059,0.203308163481623,
-5.84516273999698));
#26942=CARTESIAN_POINT('Ctrl Pts',(-0.148010061625874,0.272810181931049,
-5.85045793513847));
#26943=CARTESIAN_POINT('Ctrl Pts',(-0.0521100808352343,0.290040469587057,
-5.85575313027997));
#26944=CARTESIAN_POINT('Ctrl Pts',(0.0437898999554048,0.307270757243064,
-5.86104832542148));
#26945=CARTESIAN_POINT('Ctrl Pts',(0.149081898477497,0.272229314105654,
-5.86634352056299));
#26946=CARTESIAN_POINT('Ctrl Pts',(0.215528969047206,0.200965361943426,
-5.87163871570449));
#26947=CARTESIAN_POINT('Ctrl Pts',(0.281976039616915,0.129701409781198,
-5.87693391084599));
#26948=CARTESIAN_POINT('Ctrl Pts',(0.30957818223424,0.0222149485941525,
-5.88222910598749));
#26949=CARTESIAN_POINT('Ctrl Pts',(0.285692032174072,-0.0722451294262938,
-5.88752430112899));
#26950=CARTESIAN_POINT('Ctrl Pts',(0.261805882113904,-0.16670520744674,
-5.89281949627049));
#26951=CARTESIAN_POINT('Ctrl Pts',(0.186431439376243,-0.248138902300588,
-5.89811469141199));
#26952=CARTESIAN_POINT('Ctrl Pts',(0.0940958433066458,-0.279254488405062,
-5.9034098865535));
#26953=CARTESIAN_POINT('Ctrl Pts',(0.001760247237048,-0.310370074509537,
-5.908705081695));
#26954=CARTESIAN_POINT('Ctrl Pts',(-0.107536502164486,-0.291167551864638,
-5.9140002768365));
#26955=CARTESIAN_POINT('Ctrl Pts',(-0.183717486594243,-0.230415969954001,
-5.919295471978));
#26956=CARTESIAN_POINT('Ctrl Pts',(-0.252231886291065,-0.175778212298382,
-5.92405777741568));
#26957=CARTESIAN_POINT('Ctrl Pts',(-0.293960441403705,-0.0875332997103763,
-5.92882008285336));
#26958=CARTESIAN_POINT('Ctrl Pts',(-0.294559949103625,0.000186743463070703,
-5.93358238829104));
#26959=CARTESIAN_POINT('Ctrl Pts',(-0.294471258456466,0.000304903072910924,
-5.94801761170896));
#26960=CARTESIAN_POINT('Ctrl Pts',(-0.293803997200033,-0.0855562590056137,
-5.94335468418964));
#26961=CARTESIAN_POINT('Ctrl Pts',(-0.254074962086798,-0.172189122321664,
-5.93869175667031));
#26962=CARTESIAN_POINT('Ctrl Pts',(-0.188021191762815,-0.22697774332338,
-5.93402882915099));
#26963=CARTESIAN_POINT('Ctrl Pts',(-0.113010889276256,-0.289195403481199,
-5.92873363400948));
#26964=CARTESIAN_POINT('Ctrl Pts',(-0.00405286604006003,-0.310347524444936,
-5.92343843886798));
#26965=CARTESIAN_POINT('Ctrl Pts',(0.088859077893019,-0.280943894524006,
-5.91814324372648));
#26966=CARTESIAN_POINT('Ctrl Pts',(0.181771021826098,-0.251540264603077,
-5.91284804858498));
#26967=CARTESIAN_POINT('Ctrl Pts',(0.25863688645606,-0.171580883797481,
-5.90755285344348));
#26968=CARTESIAN_POINT('Ctrl Pts',(0.284283196980506,-0.0775964529077967,
-5.90225765830198));
#26969=CARTESIAN_POINT('Ctrl Pts',(0.309929507504952,0.0163879779818879,
-5.89696246316047));
#26970=CARTESIAN_POINT('Ctrl Pts',(0.284356263923882,0.124397458955661,
-5.89166726801896));
#26971=CARTESIAN_POINT('Ctrl Pts',(0.219258296584676,0.196899540204839,
-5.88637207287746));
#26972=CARTESIAN_POINT('Ctrl Pts',(0.154160329245471,0.269401621454017,
-5.88107687773596));
#26973=CARTESIAN_POINT('Ctrl Pts',(0.0495376381481295,0.306396302978599,
-5.87578168259446));
#26974=CARTESIAN_POINT('Ctrl Pts',(-0.0466695936054424,0.290962258147836,
-5.87048648745296));
#26975=CARTESIAN_POINT('Ctrl Pts',(-0.142876825359014,0.275528213317072,
-5.86519129231146));
#26976=CARTESIAN_POINT('Ctrl Pts',(-0.230668597768817,0.207665442130963,
-5.85989609716995));
#26977=CARTESIAN_POINT('Ctrl Pts',(-0.269831522332246,0.118449307439144,
-5.85460090202845));
#26978=CARTESIAN_POINT('Ctrl Pts',(-0.286061387034849,0.0814764354823459,
-5.85240647192195));
#26979=CARTESIAN_POINT('Ctrl Pts',(-0.293939577487073,0.0408362684106601,
-5.85021204181546));
#26980=CARTESIAN_POINT('Ctrl Pts',(-0.293774534382448,0.000134529535736241,
-5.84801761170896));
#26981=CARTESIAN_POINT('Origin',(0.,0.,-4.78));
#26982=CARTESIAN_POINT('',(-0.293985954688873,-0.000246338135983792,-5.73358238829104));
#26983=CARTESIAN_POINT('',(-0.294035653894533,-0.000257348498283876,-5.74801761170896));
#26984=CARTESIAN_POINT('',(-0.2942,-3.60291088309151E-17,-4.78));
#26985=CARTESIAN_POINT('Ctrl Pts',(-0.293985954688873,-0.000246338135983792,
-5.73358238829104));
#26986=CARTESIAN_POINT('Ctrl Pts',(-0.293449964951742,0.0674637013066885,
-5.7372396029635));
#26987=CARTESIAN_POINT('Ctrl Pts',(-0.270196227990946,0.135506165383028,
-5.74089681763597));
#26988=CARTESIAN_POINT('Ctrl Pts',(-0.227393008719715,0.187434463377991,
-5.74455403230843));
#26989=CARTESIAN_POINT('Ctrl Pts',(-0.165419233859773,0.262620225187336,
-5.74984922744993));
#26990=CARTESIAN_POINT('Ctrl Pts',(-0.0624629735245657,0.304025114087145,
-5.75514442259143));
#26991=CARTESIAN_POINT('Ctrl Pts',(0.0343097335839951,0.292680871287088,
-5.76043961773294));
#26992=CARTESIAN_POINT('Ctrl Pts',(0.131082440692556,0.281336628487032,
-5.76573481287444));
#26993=CARTESIAN_POINT('Ctrl Pts',(0.22167159457447,0.217243253987109,-5.77103000801594));
#26994=CARTESIAN_POINT('Ctrl Pts',(0.26457671740946,0.129762959220209,-5.77632520315744));
#26995=CARTESIAN_POINT('Ctrl Pts',(0.307481840244449,0.0422826644533097,
-5.78162039829895));
#26996=CARTESIAN_POINT('Ctrl Pts',(0.302702932032513,-0.0685845505805679,
-5.78691559344045));
#26997=CARTESIAN_POINT('Ctrl Pts',(0.252429325191917,-0.15204834975367,
-5.79221078858195));
#26998=CARTESIAN_POINT('Ctrl Pts',(0.202155718351321,-0.235512148926771,
-5.79750598372345));
#26999=CARTESIAN_POINT('Ctrl Pts',(0.106387412882064,-0.291572532239098,
-5.80280117886496));
#27000=CARTESIAN_POINT('Ctrl Pts',(0.00899746792928702,-0.294547543830657,
-5.80809637400646));
#27001=CARTESIAN_POINT('Ctrl Pts',(-0.0883924770234898,-0.297522555422217,
-5.81339156914796));
#27002=CARTESIAN_POINT('Ctrl Pts',(-0.187404061459786,-0.24741219529301,
-5.81868676428946));
#27003=CARTESIAN_POINT('Ctrl Pts',(-0.242678243985961,-0.167172351862406,
-5.82398195943096));
#27004=CARTESIAN_POINT('Ctrl Pts',(-0.276083110282096,-0.118679527203212,
-5.82718210238432));
#27005=CARTESIAN_POINT('Ctrl Pts',(-0.293513457201069,-0.0591822991317833,
-5.83038224533768));
#27006=CARTESIAN_POINT('Ctrl Pts',(-0.29380273100684,0.000158508790185821,
-5.83358238829104));
#27007=CARTESIAN_POINT('Ctrl Pts',(-0.293774534382448,0.000134529535736241,
-5.84801761170896));
#27008=CARTESIAN_POINT('Ctrl Pts',(-0.293541325821111,-0.0573776821285201,
-5.84491684667396));
#27009=CARTESIAN_POINT('Ctrl Pts',(-0.277248880893283,-0.115012828945004,
-5.84181608163895));
#27010=CARTESIAN_POINT('Ctrl Pts',(-0.245767387391927,-0.162598270025468,
-5.83871531660395));
#27011=CARTESIAN_POINT('Ctrl Pts',(-0.192006251171125,-0.243860214600734,
-5.83342012146245));
#27012=CARTESIAN_POINT('Ctrl Pts',(-0.0939499020124678,-0.295814605553739,
-5.82812492632094));
#27013=CARTESIAN_POINT('Ctrl Pts',(0.00347886280310267,-0.294663916819073,
-5.82282973117944));
#27014=CARTESIAN_POINT('Ctrl Pts',(0.100907627618673,-0.293513228084406,
-5.81753453603794));
#27015=CARTESIAN_POINT('Ctrl Pts',(0.197708808091157,-0.239257459662068,
-5.81223934089643));
#27016=CARTESIAN_POINT('Ctrl Pts',(0.249536873817293,-0.156750214773644,
-5.80694414575493));
#27017=CARTESIAN_POINT('Ctrl Pts',(0.30136493954343,-0.0742429698852198,
-5.80164895061343));
#27018=CARTESIAN_POINT('Ctrl Pts',(0.308219890523219,0.036515751469291,
-5.79635375547193));
#27019=CARTESIAN_POINT('Ctrl Pts',(0.266960957499969,0.12478447396498,-5.79105856033042));
#27020=CARTESIAN_POINT('Ctrl Pts',(0.22570202447672,0.213053196460669,-5.78576336518892));
#27021=CARTESIAN_POINT('Ctrl Pts',(0.136329207450433,0.278831920097537,
-5.78046817004742));
#27022=CARTESIAN_POINT('Ctrl Pts',(0.0397859484585213,0.291986781501344,
-5.77517297490592));
#27023=CARTESIAN_POINT('Ctrl Pts',(-0.0567573105333909,0.30514164290515,
-5.76987777976442));
#27024=CARTESIAN_POINT('Ctrl Pts',(-0.160471011490928,0.265672642075894,
-5.76458258462291));
#27025=CARTESIAN_POINT('Ctrl Pts',(-0.223842216941555,0.191660948472357,
-5.75928738948141));
#27026=CARTESIAN_POINT('Ctrl Pts',(-0.26879991812259,0.139154520966846,
-5.75553079689059));
#27027=CARTESIAN_POINT('Ctrl Pts',(-0.293453366349353,0.0692628632469418,
-5.75177420429978));
#27028=CARTESIAN_POINT('Ctrl Pts',(-0.294035653894533,-0.000257348498283876,
-5.74801761170896));
#27029=CARTESIAN_POINT('Origin',(0.,0.,-4.78));
#27030=CARTESIAN_POINT('',(-0.294682139675626,-2.60825238454776E-5,-5.63358238829104));
#27031=CARTESIAN_POINT('',(-0.294684718001967,8.11877721581833E-6,-5.64801761170896));
#27032=CARTESIAN_POINT('',(-0.2942,-3.60291088309151E-17,-4.78));
#27033=CARTESIAN_POINT('Ctrl Pts',(-0.294682139675626,-2.60825238454776E-5,
-5.63358238829104));
#27034=CARTESIAN_POINT('Ctrl Pts',(-0.294560459013795,0.0960166948008084,
-5.63880176544782));
#27035=CARTESIAN_POINT('Ctrl Pts',(-0.243173253454164,0.192171161974052,
-5.6440211426046));
#27036=CARTESIAN_POINT('Ctrl Pts',(-0.163207802563854,0.245361916625028,
-5.64924051976138));
#27037=CARTESIAN_POINT('Ctrl Pts',(-0.0820807534307584,0.299325333550112,
-5.65453571490289));
#27038=CARTESIAN_POINT('Ctrl Pts',(0.0284608409375124,0.309067768716717,
-5.6598309100444));
#27039=CARTESIAN_POINT('Ctrl Pts',(0.117775960523091,0.270126044465011,
-5.6651261051859));
#27040=CARTESIAN_POINT('Ctrl Pts',(0.20709108010867,0.231184320213304,-5.6704213003274));
#27041=CARTESIAN_POINT('Ctrl Pts',(0.275179724911557,0.143558436543284,
-5.6757164954689));
#27042=CARTESIAN_POINT('Ctrl Pts',(0.29084930638562,0.0473913279882392,
-5.6810116906104));
#27043=CARTESIAN_POINT('Ctrl Pts',(0.306518887859683,-0.0487757805668053,
-5.6863068857519));
#27044=CARTESIAN_POINT('Ctrl Pts',(0.269769406004923,-0.153484114006876,
-5.69160208089341));
#27045=CARTESIAN_POINT('Ctrl Pts',(0.197436435974479,-0.218764967327266,
-5.69689727603491));
#27046=CARTESIAN_POINT('Ctrl Pts',(0.125103465944034,-0.284045820647656,
-5.70219247117641));
#27047=CARTESIAN_POINT('Ctrl Pts',(0.0171870077379044,-0.309899193848366,
-5.70748766631791));
#27048=CARTESIAN_POINT('Ctrl Pts',(-0.0768745400119588,-0.284481213918727,
-5.71278286145941));
#27049=CARTESIAN_POINT('Ctrl Pts',(-0.170936087761821,-0.259063233989088,
-5.71807805660091));
#27050=CARTESIAN_POINT('Ctrl Pts',(-0.251142725055418,-0.182373900929101,
-5.72337325174242));
#27051=CARTESIAN_POINT('Ctrl Pts',(-0.280750399009877,-0.0895459170396675,
-5.72866844688392));
#27052=CARTESIAN_POINT('Ctrl Pts',(-0.289909040075056,-0.0608311255111185,
-5.73030642735296));
#27053=CARTESIAN_POINT('Ctrl Pts',(-0.294226011890775,-0.0305720729089783,
-5.731944407822));
#27054=CARTESIAN_POINT('Ctrl Pts',(-0.293985954688873,-0.000246338135983792,
-5.73358238829104));
#27055=CARTESIAN_POINT('Ctrl Pts',(-0.294035653894533,-0.000257348498283876,
-5.74801761170896));
#27056=CARTESIAN_POINT('Ctrl Pts',(-0.294274143717581,-0.0287310177955373,
-5.74647900915827));
#27057=CARTESIAN_POINT('Ctrl Pts',(-0.290474676140753,-0.0571423767188976,
-5.74494040660759));
#27058=CARTESIAN_POINT('Ctrl Pts',(-0.28237844057963,-0.084271428370518,
-5.7434018040569));
#27059=CARTESIAN_POINT('Ctrl Pts',(-0.254514748823363,-0.17763772523204,
-5.7381066089154));
#27060=CARTESIAN_POINT('Ctrl Pts',(-0.175758655367114,-0.255815932577267,
-5.7328114137739));
#27061=CARTESIAN_POINT('Ctrl Pts',(-0.0821897200362796,-0.282991329357579,
-5.7275162186324));
#27062=CARTESIAN_POINT('Ctrl Pts',(0.011379215294555,-0.310166726137891,
-5.72222102349089));
#27063=CARTESIAN_POINT('Ctrl Pts',(0.119760992499974,-0.286339312353287,
-5.71692582834939));
#27064=CARTESIAN_POINT('Ctrl Pts',(0.193304055814128,-0.222424802657665,
-5.71163063320789));
#27065=CARTESIAN_POINT('Ctrl Pts',(0.266847119128281,-0.158510292962043,
-5.70633543806639));
#27066=CARTESIAN_POINT('Ctrl Pts',(0.305551468551169,-0.0545086873554045,
-5.70104024292489));
#27067=CARTESIAN_POINT('Ctrl Pts',(0.291685963198157,0.0419350572632446,
-5.69574504778339));
#27068=CARTESIAN_POINT('Ctrl Pts',(0.277820457845145,0.138378801881894,
-5.69044985264189));
#27069=CARTESIAN_POINT('Ctrl Pts',(0.211385097716233,0.227264685512553,
-5.68515465750038));
#27070=CARTESIAN_POINT('Ctrl Pts',(0.122815076627005,0.267872554166424,
-5.67985946235887));
#27071=CARTESIAN_POINT('Ctrl Pts',(0.0342450555377765,0.308480422820294,
-5.67456426721737));
#27072=CARTESIAN_POINT('Ctrl Pts',(-0.0764596265117672,0.300810276497374,
-5.66926907207587));
#27073=CARTESIAN_POINT('Ctrl Pts',(-0.158583238089704,0.248375937095584,
-5.66397387693437));
#27074=CARTESIAN_POINT('Ctrl Pts',(-0.240706849667642,0.195941597693793,
-5.65867868179287));
#27075=CARTESIAN_POINT('Ctrl Pts',(-0.294249390773972,0.0987430652131304,
-5.65338348665136));
#27076=CARTESIAN_POINT('Ctrl Pts',(-0.294682094323317,0.00130867455497656,
-5.64808829150986));
#27077=CARTESIAN_POINT('Ctrl Pts',(-0.294684019553008,0.000875159317817163,
-5.64806473157622));
#27078=CARTESIAN_POINT('Ctrl Pts',(-0.294684893404035,0.000441639411536826,
-5.64804117164259));
#27079=CARTESIAN_POINT('Ctrl Pts',(-0.294684718001967,8.11877721581833E-6,
-5.64801761170896));
#27080=CARTESIAN_POINT('Origin',(0.,0.,-4.78));
#27081=CARTESIAN_POINT('',(-0.294062830248701,0.000261802542909251,-5.53358238829104));
#27082=CARTESIAN_POINT('',(-0.294011745337965,0.000252542567362749,-5.54801761170896));
#27083=CARTESIAN_POINT('',(-0.2942,-3.60291088309151E-17,-4.78));
#27084=CARTESIAN_POINT('Ctrl Pts',(-0.294062830248701,0.000261802542909251,
-5.53358238829104));
#27085=CARTESIAN_POINT('Ctrl Pts',(-0.294298842664649,0.0277619258901645,
-5.53506873279064));
#27086=CARTESIAN_POINT('Ctrl Pts',(-0.290757561165195,0.0552024351269035,
-5.53655507729024));
#27087=CARTESIAN_POINT('Ctrl Pts',(-0.28319483979987,0.081485824609101,
-5.53804142178984));
#27088=CARTESIAN_POINT('Ctrl Pts',(-0.256252172443144,0.175122041734979,
-5.54333661693134));
#27089=CARTESIAN_POINT('Ctrl Pts',(-0.178269987897413,0.254072266884979,
-5.54863181207284));
#27090=CARTESIAN_POINT('Ctrl Pts',(-0.084973276416993,0.282168033621128,
-5.55392700721435));
#27091=CARTESIAN_POINT('Ctrl Pts',(0.00832343506342488,0.310263800357276,
-5.55922220235585));
#27092=CARTESIAN_POINT('Ctrl Pts',(0.116934673478531,0.287505108679576,
-5.56451739749735));
#27093=CARTESIAN_POINT('Ctrl Pts',(0.191103748167855,0.224318109691484,
-5.56981259263885));
#27094=CARTESIAN_POINT('Ctrl Pts',(0.265272822857179,0.161131110703392,
-5.57510778778036));
#27095=CARTESIAN_POINT('Ctrl Pts',(0.304999733820722,0.0575158044049082,
-5.58040298292186));
#27096=CARTESIAN_POINT('Ctrl Pts',(0.29208489463139,-0.0390598416549937,
-5.58569817806336));
#27097=CARTESIAN_POINT('Ctrl Pts',(0.279170055442058,-0.135635487714897,
-5.59099337320486));
#27098=CARTESIAN_POINT('Ctrl Pts',(0.213613466099853,-0.225171473536216,
-5.59628856834637));
#27099=CARTESIAN_POINT('Ctrl Pts',(0.125447736357934,-0.266649812209754,
-5.60158376348787));
#27100=CARTESIAN_POINT('Ctrl Pts',(0.0372820066160163,-0.308128150883291,
-5.60687895862937));
#27101=CARTESIAN_POINT('Ctrl Pts',(-0.0734928635256134,-0.301548842409048,
-5.61217415377087));
#27102=CARTESIAN_POINT('Ctrl Pts',(-0.156128986234019,-0.249925982127323,
-5.61746934891237));
#27103=CARTESIAN_POINT('Ctrl Pts',(-0.238765108942426,-0.198303121845597,
-5.62276454405388));
#27104=CARTESIAN_POINT('Ctrl Pts',(-0.293262484217608,-0.101636709756389,
-5.62805973919538));
#27105=CARTESIAN_POINT('Ctrl Pts',(-0.294654919906238,-0.00421130437000306,
-5.63335493433688));
#27106=CARTESIAN_POINT('Ctrl Pts',(-0.294674857163496,-0.002816342012704,
-5.6334307523216));
#27107=CARTESIAN_POINT('Ctrl Pts',(-0.29468390723951,-0.00142122405222277,
-5.63350657030632));
#27108=CARTESIAN_POINT('Ctrl Pts',(-0.294682139675626,-2.60825238454776E-5,
-5.63358238829104));
#27109=CARTESIAN_POINT('Ctrl Pts',(-0.294684718001967,8.11877721581833E-6,
-5.64801761170896));
#27110=CARTESIAN_POINT('Ctrl Pts',(-0.294645471044368,-0.0969939642816139,
-5.64274597650109));
#27111=CARTESIAN_POINT('Ctrl Pts',(-0.242074357435456,-0.194032497397622,
-5.63747434129323));
#27112=CARTESIAN_POINT('Ctrl Pts',(-0.160783000885537,-0.246957639589329,
-5.63220270608536));
#27113=CARTESIAN_POINT('Ctrl Pts',(-0.0791283379060545,-0.300119314239834,
-5.62690751094386));
#27114=CARTESIAN_POINT('Ctrl Pts',(0.0315038540452678,-0.308772414705198,
-5.62161231580235));
#27115=CARTESIAN_POINT('Ctrl Pts',(0.120431050747587,-0.268952804993428,
-5.61631712066085));
#27116=CARTESIAN_POINT('Ctrl Pts',(0.209358247449906,-0.229133195281657,
-5.61102192551934));
#27117=CARTESIAN_POINT('Ctrl Pts',(0.276580448903222,-0.140840875392752,
-5.60572673037785));
#27118=CARTESIAN_POINT('Ctrl Pts',(0.291301999444768,-0.0445240876285061,
-5.60043153523634));
#27119=CARTESIAN_POINT('Ctrl Pts',(0.306023549986313,0.0517927001357388,
-5.59513634009484));
#27120=CARTESIAN_POINT('Ctrl Pts',(0.268244449616089,0.156133955775324,
-5.58984114495334));
#27121=CARTESIAN_POINT('Ctrl Pts',(0.195271959040515,0.220699141927202,
-5.58454594981184));
#27122=CARTESIAN_POINT('Ctrl Pts',(0.12229946846494,0.285264328079082,-5.57925075467033));
#27123=CARTESIAN_POINT('Ctrl Pts',(0.0141335876840122,0.310053444743254,
-5.57395555952883));
#27124=CARTESIAN_POINT('Ctrl Pts',(-0.0796730187285941,0.28371016785751,
-5.56866036438733));
#27125=CARTESIAN_POINT('Ctrl Pts',(-0.1734796251412,0.257366890971767,-5.56336516924582));
#27126=CARTESIAN_POINT('Ctrl Pts',(-0.252926957185485,0.179891220536109,
-5.55806997410432));
#27127=CARTESIAN_POINT('Ctrl Pts',(-0.281618815126852,0.0867761039612887,
-5.55277477896282));
#27128=CARTESIAN_POINT('Ctrl Pts',(-0.290211005052726,0.0588914417614489,
-5.55118905654487));
#27129=CARTESIAN_POINT('Ctrl Pts',(-0.294251498631625,0.0296042508468538,
-5.54960333412692));
#27130=CARTESIAN_POINT('Ctrl Pts',(-0.294011745337965,0.000252542567362749,
-5.54801761170896));
#27131=CARTESIAN_POINT('Origin',(0.,0.,-4.78));
#27132=CARTESIAN_POINT('',(-0.293762945406406,-0.000118368460801849,-5.43358238829104));
#27133=CARTESIAN_POINT('',(-0.293787729549656,-0.000144936987199139,-5.44801761170896));
#27134=CARTESIAN_POINT('',(-0.2942,-3.60291088309151E-17,-4.78));
#27135=CARTESIAN_POINT('Ctrl Pts',(-0.293762945406406,-0.000118368460801849,
-5.43358238829104));
#27136=CARTESIAN_POINT('Ctrl Pts',(-0.29355838126358,0.0564296933406882,
-5.43663089527496));
#27137=CARTESIAN_POINT('Ctrl Pts',(-0.27784549825086,0.113082938218205,
-5.43967940225888));
#27138=CARTESIAN_POINT('Ctrl Pts',(-0.247356669228761,0.160168458472912,
-5.4427279092428));
#27139=CARTESIAN_POINT('Ctrl Pts',(-0.194398188188848,0.241955057422185,
-5.4480231043843));
#27140=CARTESIAN_POINT('Ctrl Pts',(-0.0968592162767127,0.29487488466396,
-5.4533182995258));
#27141=CARTESIAN_POINT('Ctrl Pts',(0.00057595302291618,0.294684450183038,
-5.4586134946673));
#27142=CARTESIAN_POINT('Ctrl Pts',(0.0980111223225464,0.294494015702115,
-5.4639086898088));
#27143=CARTESIAN_POINT('Ctrl Pts',(0.19534248900967,0.241193319498494,-5.46920388495031));
#27144=CARTESIAN_POINT('Ctrl Pts',(0.247980867151239,0.159200334259781,
-5.47449908009182));
#27145=CARTESIAN_POINT('Ctrl Pts',(0.300619245292808,0.0772073490210695,
-5.47979427523332));
#27146=CARTESIAN_POINT('Ctrl Pts',(0.308564634888824,-0.033477925252733,
-5.48508947037482));
#27147=CARTESIAN_POINT('Ctrl Pts',(0.268177115263378,-0.122148646126489,
-5.49038466551632));
#27148=CARTESIAN_POINT('Ctrl Pts',(0.227789595637931,-0.210819367000247,
-5.49567986065782));
#27149=CARTESIAN_POINT('Ctrl Pts',(0.13906916679102,-0.277475534473958,
-5.50097505579933));
#27150=CARTESIAN_POINT('Ctrl Pts',(0.0426601947948733,-0.291580803006248,
-5.50627025094083));
#27151=CARTESIAN_POINT('Ctrl Pts',(-0.0537487772012731,-0.305686071538539,
-5.51156544608233));
#27152=CARTESIAN_POINT('Ctrl Pts',(-0.157846292346655,-0.26724044112941,
-5.51686064122383));
#27153=CARTESIAN_POINT('Ctrl Pts',(-0.221943474835486,-0.193856521373968,
-5.52215583636533));
#27154=CARTESIAN_POINT('Ctrl Pts',(-0.26804878127703,-0.141071235393637,
-5.52596468700723));
#27155=CARTESIAN_POINT('Ctrl Pts',(-0.293458033687594,-0.0702089816473159,
-5.52977353764913));
#27156=CARTESIAN_POINT('Ctrl Pts',(-0.294062830248701,0.000261802542909251,
-5.53358238829104));
#27157=CARTESIAN_POINT('Ctrl Pts',(-0.294011745337965,0.000252542567362749,
-5.54801761170896));
#27158=CARTESIAN_POINT('Ctrl Pts',(-0.293450891626658,-0.0684097655514012,
-5.54430813898541));
#27159=CARTESIAN_POINT('Ctrl Pts',(-0.269467235735366,-0.137425132154906,
-5.54059866626186));
#27160=CARTESIAN_POINT('Ctrl Pts',(-0.225535691601695,-0.18966523419781,
-5.53688919353831));
#27161=CARTESIAN_POINT('Ctrl Pts',(-0.162824326296723,-0.264236893068108,
-5.53159399839681));
#27162=CARTESIAN_POINT('Ctrl Pts',(-0.0594652118483327,-0.304625648094722,
-5.52629880325531));
#27163=CARTESIAN_POINT('Ctrl Pts',(0.0371910500992316,-0.292328710607396,
-5.52100360811381));
#27164=CARTESIAN_POINT('Ctrl Pts',(0.133847312046796,-0.28003177312007,
-5.51570841297231));
#27165=CARTESIAN_POINT('Ctrl Pts',(0.223800721493533,-0.215049143118806,
-5.5104132178308));
#27166=CARTESIAN_POINT('Ctrl Pts',(0.265842062583014,-0.127150489630659,
-5.5051180226893));
#27167=CARTESIAN_POINT('Ctrl Pts',(0.307883403672496,-0.0392518361425124,
-5.4998228275478));
#27168=CARTESIAN_POINT('Ctrl Pts',(0.302012676404721,0.0715628408325163,
-5.4945276324063));
#27169=CARTESIAN_POINT('Ctrl Pts',(0.250919362688317,0.154527417242256,
-5.48923243726479));
#27170=CARTESIAN_POINT('Ctrl Pts',(0.199826048971912,0.237491993651996,
-5.48393724212329));
#27171=CARTESIAN_POINT('Ctrl Pts',(0.103510148806877,0.292606469496448,
-5.47864204698179));
#27172=CARTESIAN_POINT('Ctrl Pts',(0.00609564531270745,0.294621948198257,
-5.47334685184029));
#27173=CARTESIAN_POINT('Ctrl Pts',(-0.0913188581814613,0.296637426900067,
-5.46805165669878));
#27174=CARTESIAN_POINT('Ctrl Pts',(-0.189831965004765,0.245553908459236,
-5.46275646155728));
#27175=CARTESIAN_POINT('Ctrl Pts',(-0.244313113586537,0.164773638004936,
-5.45746126641578));
#27176=CARTESIAN_POINT('Ctrl Pts',(-0.276701038959653,0.116751424097918,
-5.45431338151351));
#27177=CARTESIAN_POINT('Ctrl Pts',(-0.29352781213388,0.0582342039193331,
-5.45116549661124));
#27178=CARTESIAN_POINT('Ctrl Pts',(-0.293787729549656,-0.000144936987199139,
-5.44801761170896));
#27179=CARTESIAN_POINT('Origin',(0.,0.,-4.78));
#27180=CARTESIAN_POINT('',(-0.294496711936401,-0.000204427085817055,-5.33358238829104));
#27181=CARTESIAN_POINT('',(-0.294542023011264,-0.000181426215594961,-5.34801761170896));
#27182=CARTESIAN_POINT('',(-0.2942,-3.60291088309151E-17,-4.78));
#27183=CARTESIAN_POINT('Ctrl Pts',(-0.294496711936401,-0.000204427085817055,
-5.33358238829104));
#27184=CARTESIAN_POINT('Ctrl Pts',(-0.293823771455211,0.084778691105119,
-5.33819305775928));
#27185=CARTESIAN_POINT('Ctrl Pts',(-0.255021031632015,0.170297643646105,
-5.34280372722752));
#27186=CARTESIAN_POINT('Ctrl Pts',(-0.190225443788733,0.225063407591993,
-5.34741439669576));
#27187=CARTESIAN_POINT('Ctrl Pts',(-0.115809942026555,0.287960001929239,
-5.35270959183726));
#27188=CARTESIAN_POINT('Ctrl Pts',(-0.00711057119819164,0.310293965717217,
-5.35800478697876));
#27189=CARTESIAN_POINT('Ctrl Pts',(0.0860756030468191,0.281833723073849,
-5.36329998212026));
#27190=CARTESIAN_POINT('Ctrl Pts',(0.179261777291827,0.253373480430482,
-5.36859517726177));
#27191=CARTESIAN_POINT('Ctrl Pts',(0.256934754953484,0.174119031355772,
-5.37389037240327));
#27192=CARTESIAN_POINT('Ctrl Pts',(0.283511198811562,0.0803782125328151,
-5.37918556754477));
#27193=CARTESIAN_POINT('Ctrl Pts',(0.310087642669642,-0.0133626062901439,
-5.38448076268627));
#27194=CARTESIAN_POINT('Ctrl Pts',(0.285567552724141,-0.121589794861351,
-5.38977595782778));
#27195=CARTESIAN_POINT('Ctrl Pts',(0.221184007137732,-0.194722602406693,
-5.39507115296928));
#27196=CARTESIAN_POINT('Ctrl Pts',(0.156800461551325,-0.267855409952034,
-5.40036634811078));
#27197=CARTESIAN_POINT('Ctrl Pts',(0.052553460324011,-0.305893836471511,
-5.40566154325228));
#27198=CARTESIAN_POINT('Ctrl Pts',(-0.0437996385731037,-0.29141181953107,
-5.41095673839378));
#27199=CARTESIAN_POINT('Ctrl Pts',(-0.140152737470219,-0.276929802590629,
-5.41625193353528));
#27200=CARTESIAN_POINT('Ctrl Pts',(-0.228611934037135,-0.209927342190269,
-5.42154712867679));
#27201=CARTESIAN_POINT('Ctrl Pts',(-0.268652537236749,-0.121099426661703,
-5.42684232381829));
#27202=CARTESIAN_POINT('Ctrl Pts',(-0.28564128772226,-0.0834108013045968,
-5.42908901197587));
#27203=CARTESIAN_POINT('Ctrl Pts',(-0.293913705053531,-0.0417931494122248,
-5.43133570013346));
#27204=CARTESIAN_POINT('Ctrl Pts',(-0.293762945406406,-0.000118368460801849,
-5.43358238829104));
#27205=CARTESIAN_POINT('Ctrl Pts',(-0.293787729549656,-0.000144936987199139,
-5.44801761170896));
#27206=CARTESIAN_POINT('Ctrl Pts',(-0.293965030609122,-0.039967907304658,
-5.44587030146973));
#27207=CARTESIAN_POINT('Ctrl Pts',(-0.286433439129297,-0.0797266265484263,
-5.4437229912305));
#27208=CARTESIAN_POINT('Ctrl Pts',(-0.270873729417273,-0.11604599072477,
-5.44157568099127));
#27209=CARTESIAN_POINT('Ctrl Pts',(-0.232504006325994,-0.205608326532409,
-5.43628048584977));
#27210=CARTESIAN_POINT('Ctrl Pts',(-0.145315369803193,-0.27425597567992,
-5.43098529070827));
#27211=CARTESIAN_POINT('Ctrl Pts',(-0.0492504453095419,-0.290540260357468,
-5.42569009556676));
#27212=CARTESIAN_POINT('Ctrl Pts',(0.0468144791841089,-0.306824545035016,
-5.42039490042526));
#27213=CARTESIAN_POINT('Ctrl Pts',(0.15175569164861,-0.270745465242601,
-5.41509970528376));
#27214=CARTESIAN_POINT('Ctrl Pts',(0.217497803913647,-0.19883147272121,
-5.40980451014226));
#27215=CARTESIAN_POINT('Ctrl Pts',(0.283239916178685,-0.126917480199819,
-5.40450931500076));
#27216=CARTESIAN_POINT('Ctrl Pts',(0.30978292824426,-0.0191685749494507,
-5.39921411985926));
#27217=CARTESIAN_POINT('Ctrl Pts',(0.284967026265175,0.0750536021342638,
-5.39391892471775));
#27218=CARTESIAN_POINT('Ctrl Pts',(0.26015112428609,0.169275779217978,-5.38862372957625));
#27219=CARTESIAN_POINT('Ctrl Pts',(0.183976308262347,0.249971228135038,
-5.38332853443475));
#27220=CARTESIAN_POINT('Ctrl Pts',(0.0913395816031329,0.280171965200513,
-5.37803333929324));
#27221=CARTESIAN_POINT('Ctrl Pts',(-0.00129714505608075,0.310372702265987,
-5.37273814415174));
#27222=CARTESIAN_POINT('Ctrl Pts',(-0.110395782350765,0.290078727479875,
-5.36744294901024));
#27223=CARTESIAN_POINT('Ctrl Pts',(-0.185976353743453,0.228587062407386,
-5.36214775386874));
#27224=CARTESIAN_POINT('Ctrl Pts',(-0.253204862467365,0.173890559515195,
-5.35743770648215));
#27225=CARTESIAN_POINT('Ctrl Pts',(-0.293913856983524,0.0865984189131595,
-5.35272765909555));
#27226=CARTESIAN_POINT('Ctrl Pts',(-0.294542023011264,-0.000181426215594961,
-5.34801761170896));
#27227=CARTESIAN_POINT('Origin',(0.,0.,-4.78));
#27228=CARTESIAN_POINT('',(-0.294398673878215,0.000239804230613712,-5.23358238829104));
#27229=CARTESIAN_POINT('',(-0.294344694043696,0.00025285010085293,-5.24801761170896));
#27230=CARTESIAN_POINT('',(-0.2942,-3.60291088309151E-17,-4.78));
#27231=CARTESIAN_POINT('Ctrl Pts',(-0.294398673878215,0.000239804230613712,
-5.23358238829104));
#27232=CARTESIAN_POINT('Ctrl Pts',(-0.294541575596084,0.0164302863513783,
-5.2344600251021));
#27233=CARTESIAN_POINT('Ctrl Pts',(-0.293321228623321,0.0325992101967099,
-5.23533766191315));
#27234=CARTESIAN_POINT('Ctrl Pts',(-0.290661834729239,0.0485278758382486,
-5.23621529872421));
#27235=CARTESIAN_POINT('Ctrl Pts',(-0.274616462144716,0.144632997972109,
-5.24151049386571));
#27236=CARTESIAN_POINT('Ctrl Pts',(-0.206185814037005,0.231992059073534,
-5.24680568900721));
#27237=CARTESIAN_POINT('Ctrl Pts',(-0.116719156278496,0.270584359228645,
-5.25210088414871));
#27238=CARTESIAN_POINT('Ctrl Pts',(-0.0272524985199846,0.309176659383756,
-5.25739607929022));
#27239=CARTESIAN_POINT('Ctrl Pts',(0.0832501688893253,0.299002198592552,
-5.26269127443172));
#27240=CARTESIAN_POINT('Ctrl Pts',(0.164165658883164,0.244722073677462,
-5.26798646957322));
#27241=CARTESIAN_POINT('Ctrl Pts',(0.245081148877002,0.190441948762372,
-5.27328166471472));
#27242=CARTESIAN_POINT('Ctrl Pts',(0.296409461455368,0.0920561597233961,
-5.27857685985622));
#27243=CARTESIAN_POINT('Ctrl Pts',(0.294636207053114,-0.0053630583527391,
-5.28387205499773));
#27244=CARTESIAN_POINT('Ctrl Pts',(0.292862952650859,-0.102782276428872,
-5.28916725013923));
#27245=CARTESIAN_POINT('Ctrl Pts',(0.237988131267985,-0.199234923542167,
-5.29446244528074));
#27246=CARTESIAN_POINT('Ctrl Pts',(0.155150849617668,-0.250534370425409,
-5.29975764042224));
#27247=CARTESIAN_POINT('Ctrl Pts',(0.0723135679673499,-0.301833817308652,
-5.30505283556374));
#27248=CARTESIAN_POINT('Ctrl Pts',(-0.03848617395041,-0.307980063961841,
-5.31034803070524));
#27249=CARTESIAN_POINT('Ctrl Pts',(-0.126489094088413,-0.266157408272309,
-5.31564322584674));
#27250=CARTESIAN_POINT('Ctrl Pts',(-0.214492014226414,-0.224334752582778,
-5.32093842098825));
#27251=CARTESIAN_POINT('Ctrl Pts',(-0.279698112584657,-0.134543194550528,
-5.32623361612975));
#27252=CARTESIAN_POINT('Ctrl Pts',(-0.292235345415782,-0.0379178030911469,
-5.33152881127125));
#27253=CARTESIAN_POINT('Ctrl Pts',(-0.293856070906581,-0.0254267504716328,
-5.33221333694452));
#27254=CARTESIAN_POINT('Ctrl Pts',(-0.294596620428893,-0.0128214942159667,
-5.33289786261778));
#27255=CARTESIAN_POINT('Ctrl Pts',(-0.294496711936401,-0.000204427085817055,
-5.33358238829104));
#27256=CARTESIAN_POINT('Ctrl Pts',(-0.294542023011264,-0.000181426215594961,
-5.34801761170896));
#27257=CARTESIAN_POINT('Ctrl Pts',(-0.294620062553263,-0.0109624284817407,
-5.34743246395405));
#27258=CARTESIAN_POINT('Ctrl Pts',(-0.294079491686475,-0.021735523942461,
-5.34684731619914));
#27259=CARTESIAN_POINT('Ctrl Pts',(-0.292894307463314,-0.0324372302660748,
-5.34626216844423));
#27260=CARTESIAN_POINT('Ctrl Pts',(-0.282169184299795,-0.129280502508182,
-5.34096697330273));
#27261=CARTESIAN_POINT('Ctrl Pts',(-0.218656432482065,-0.220277691633531,
-5.33567177816123));
#27262=CARTESIAN_POINT('Ctrl Pts',(-0.131452344359818,-0.263741408227941,
-5.33037658301973));
#27263=CARTESIAN_POINT('Ctrl Pts',(-0.0442482562375699,-0.307205124822352,
-5.32508138787822));
#27264=CARTESIAN_POINT('Ctrl Pts',(0.0666471681891957,-0.30313536888582,
-5.31978619273672));
#27265=CARTESIAN_POINT('Ctrl Pts',(0.150430813057623,-0.253396566145975,
-5.31449099759522));
#27266=CARTESIAN_POINT('Ctrl Pts',(0.234214457926051,-0.20365776340613,
-5.30919580245371));
#27267=CARTESIAN_POINT('Ctrl Pts',(0.29088632323614,-0.108249913862972,
-5.30390060731221));
#27268=CARTESIAN_POINT('Ctrl Pts',(0.294484045307019,-0.0108810069094036,
-5.29860541217071));
#27269=CARTESIAN_POINT('Ctrl Pts',(0.298081767377898,0.0864879000441643,
-5.29331021702921));
#27270=CARTESIAN_POINT('Ctrl Pts',(0.248605346209566,0.185817864408143,
-5.28801502188771));
#27271=CARTESIAN_POINT('Ctrl Pts',(0.168720787817032,0.24160410801588,-5.28271982674621));
#27272=CARTESIAN_POINT('Ctrl Pts',(0.088836229424499,0.297390351623618,
-5.2774246316047));
#27273=CARTESIAN_POINT('Ctrl Pts',(-0.0214564661922352,0.309632874475115,
-5.2721294364632));
#27274=CARTESIAN_POINT('Ctrl Pts',(-0.111630303684109,0.272723164676459,
-5.2668342413217));
#27275=CARTESIAN_POINT('Ctrl Pts',(-0.201804141175983,0.235813454877802,
-5.26153904618019));
#27276=CARTESIAN_POINT('Ctrl Pts',(-0.271859120542995,0.149751512428991,
-5.25624385103869));
#27277=CARTESIAN_POINT('Ctrl Pts',(-0.289701841611522,0.0539638047087275,
-5.25094865589719));
#27278=CARTESIAN_POINT('Ctrl Pts',(-0.292993996259435,0.0362900459825212,
-5.24997164116778));
#27279=CARTESIAN_POINT('Ctrl Pts',(-0.294508646194196,0.0182851850559431,
-5.24899462643837));
#27280=CARTESIAN_POINT('Ctrl Pts',(-0.294344694043696,0.00025285010085293,
-5.24801761170896));
#27281=CARTESIAN_POINT('Origin',(0.,0.,-4.78));
#27282=CARTESIAN_POINT('',(-0.293729850984995,6.28784883607292E-5,-5.13358238829104));
#27283=CARTESIAN_POINT('',(-0.29372088508174,3.30216514158299E-5,-5.14801761170896));
#27284=CARTESIAN_POINT('',(-0.2942,-3.60291088309151E-17,-4.78));
#27285=CARTESIAN_POINT('Ctrl Pts',(-0.293729850984995,6.28784883607292E-5,
-5.13358238829104));
#27286=CARTESIAN_POINT('Ctrl Pts',(-0.29381626506198,0.0453324939186312,
-5.13602218758642));
#27287=CARTESIAN_POINT('Ctrl Pts',(-0.283993710042448,0.090566575165814,
-5.13846198688179));
#27288=CARTESIAN_POINT('Ctrl Pts',(-0.264067456747889,0.130796158920061,
-5.14090178617717));
#27289=CARTESIAN_POINT('Ctrl Pts',(-0.220820702871991,0.218108052502425,
-5.14619698131867));
#27290=CARTESIAN_POINT('Ctrl Pts',(-0.129981713533421,0.281846872486101,
-5.15149217646017));
#27291=CARTESIAN_POINT('Ctrl Pts',(-0.033165404082267,0.292812760776576,
-5.15678737160167));
#27292=CARTESIAN_POINT('Ctrl Pts',(0.0636509053688859,0.30377864906705,
-5.16208256674318));
#27293=CARTESIAN_POINT('Ctrl Pts',(0.166444534932621,0.261971605664325,
-5.16737776188468));
#27294=CARTESIAN_POINT('Ctrl Pts',(0.228123941385365,0.186544161710697,
-5.17267295702618));
#27295=CARTESIAN_POINT('Ctrl Pts',(0.289803347838111,0.111116717757068,
-5.17796815216768));
#27296=CARTESIAN_POINT('Ctrl Pts',(0.310368531179863,0.00206887325253695,
-5.18326334730918));
#27297=CARTESIAN_POINT('Ctrl Pts',(0.280398224505767,-0.090642664322898,
-5.18855854245068));
#27298=CARTESIAN_POINT('Ctrl Pts',(0.250427917831671,-0.183354201898333,
-5.19385373759219));
#27299=CARTESIAN_POINT('Ctrl Pts',(0.169922121141726,-0.259729432544673,
-5.19914893273369));
#27300=CARTESIAN_POINT('Ctrl Pts',(0.0757619351487175,-0.284779539440708,
-5.2044441278752));
#27301=CARTESIAN_POINT('Ctrl Pts',(-0.0183982508442894,-0.309829646336743,
-5.2097393230167));
#27302=CARTESIAN_POINT('Ctrl Pts',(-0.126212826140359,-0.283554629482476,
-5.2150345181582));
#27303=CARTESIAN_POINT('Ctrl Pts',(-0.198290065257727,-0.217991529472194,
-5.2203297132997));
#27304=CARTESIAN_POINT('Ctrl Pts',(-0.258421070742859,-0.163294995939315,
-5.22474727163015));
#27305=CARTESIAN_POINT('Ctrl Pts',(-0.293679382405638,-0.0812544975871136,
-5.2291648299606));
#27306=CARTESIAN_POINT('Ctrl Pts',(-0.294398673878215,0.000239804230613712,
-5.23358238829104));
#27307=CARTESIAN_POINT('Ctrl Pts',(-0.294344694043696,0.00025285010085293,
-5.24801761170896));
#27308=CARTESIAN_POINT('Ctrl Pts',(-0.293620063243877,-0.0794459233602251,
-5.24369943129687));
#27309=CARTESIAN_POINT('Ctrl Pts',(-0.260105003184177,-0.159681384578527,
-5.23938125088478));
#27310=CARTESIAN_POINT('Ctrl Pts',(-0.202338510586488,-0.214239063630774,
-5.23506307047268));
#27311=CARTESIAN_POINT('Ctrl Pts',(-0.131501995722885,-0.281140751258297,
-5.22976787533118));
#27312=CARTESIAN_POINT('Ctrl Pts',(-0.0241985032256398,-0.309430653521625,
-5.22447268018968));
#27313=CARTESIAN_POINT('Ctrl Pts',(0.0704143773112224,-0.286148675900522,
-5.21917748504818));
#27314=CARTESIAN_POINT('Ctrl Pts',(0.165027257848083,-0.262866698279419,
-5.21388228990667));
#27315=CARTESIAN_POINT('Ctrl Pts',(0.24694952642456,-0.188012840773886,
-5.20858709476517));
#27316=CARTESIAN_POINT('Ctrl Pts',(0.278651172007717,-0.0958789528023486,
-5.20329189962367));
#27317=CARTESIAN_POINT('Ctrl Pts',(0.310352817590874,-0.00374506483081084,
-5.19799670448217));
#27318=CARTESIAN_POINT('Ctrl Pts',(0.291833840180711,0.10566885360673,-5.19270150934067));
#27319=CARTESIAN_POINT('Ctrl Pts',(0.231578104281948,0.182238390217124,
-5.18740631419916));
#27320=CARTESIAN_POINT('Ctrl Pts',(0.171322368383185,0.258807926827517,
-5.18211111905766));
#27321=CARTESIAN_POINT('Ctrl Pts',(0.0693298739958214,0.302533081610763,
-5.17681592391616));
#27322=CARTESIAN_POINT('Ctrl Pts',(-0.0276748495653676,0.293382603358283,
-5.17152072877465));
#27323=CARTESIAN_POINT('Ctrl Pts',(-0.124679573126557,0.284232125105803,
-5.16622553363315));
#27324=CARTESIAN_POINT('Ctrl Pts',(-0.216696525861573,0.222206013817596,
-5.16093033849165));
#27325=CARTESIAN_POINT('Ctrl Pts',(-0.261571146973085,0.13571950605176,
-5.15563514335015));
#27326=CARTESIAN_POINT('Ctrl Pts',(-0.283089639182754,0.0942470836111143,
-5.15309596613642));
#27327=CARTESIAN_POINT('Ctrl Pts',(-0.293768035010674,0.0471501397218707,
-5.15055678892269));
#27328=CARTESIAN_POINT('Ctrl Pts',(-0.29372088508174,3.30216514158299E-5,
-5.14801761170896));
#27329=CARTESIAN_POINT('Origin',(0.,0.,-4.78));
#27330=CARTESIAN_POINT('',(-0.294167685007082,-0.000269782114602712,-5.03358238829104));
#27331=CARTESIAN_POINT('',(-0.294223320968512,-0.000268522322062943,-5.04801761170896));
#27332=CARTESIAN_POINT('',(-0.2942,-3.60291088309151E-17,-4.78));
#27333=CARTESIAN_POINT('Ctrl Pts',(-0.294167685007082,-0.000269782114602712,
-5.03358238829104));
#27334=CARTESIAN_POINT('Ctrl Pts',(-0.2934934036862,0.0737067916099429,
-5.03758435007074));
#27335=CARTESIAN_POINT('Ctrl Pts',(-0.265170690824886,0.148143361035309,
-5.04158631185043));
#27336=CARTESIAN_POINT('Ctrl Pts',(-0.214741519260896,0.20180519519344,
-5.04558827363013));
#27337=CARTESIAN_POINT('Ctrl Pts',(-0.148016168306652,0.272807843184718,
-5.05088346877163));
#27338=CARTESIAN_POINT('Ctrl Pts',(-0.042588475632073,0.307439631678508,
-5.05617866391313));
#27339=CARTESIAN_POINT('Ctrl Pts',(0.0532433055771352,0.289835138160921,
-5.06147385905463));
#27340=CARTESIAN_POINT('Ctrl Pts',(0.149075086786345,0.272230644643333,
-5.06676905419613));
#27341=CARTESIAN_POINT('Ctrl Pts',(0.235310956530186,0.202389869114365,
-5.07206424933764));
#27342=CARTESIAN_POINT('Ctrl Pts',(0.272444768321761,0.112308081257059,
-5.07735944447914));
#27343=CARTESIAN_POINT('Ctrl Pts',(0.309578580113335,0.0222262933997549,
-5.08265463962064));
#27344=CARTESIAN_POINT('Ctrl Pts',(0.297610333952645,-0.0880965067858862,
-5.08794983476214));
#27345=CARTESIAN_POINT('Ctrl Pts',(0.242022890828046,-0.168119532526044,
-5.09324502990365));
#27346=CARTESIAN_POINT('Ctrl Pts',(0.186435447703447,-0.248142558266203,
-5.09854022504515));
#27347=CARTESIAN_POINT('Ctrl Pts',(0.0872288076149375,-0.297865809560878,
-5.10383542018665));
#27348=CARTESIAN_POINT('Ctrl Pts',(-0.010148748258762,-0.294510203236357,
-5.10913061532816));
#27349=CARTESIAN_POINT('Ctrl Pts',(-0.107526304132462,-0.291154596911837,
-5.11442581046966));
#27350=CARTESIAN_POINT('Ctrl Pts',(-0.203074775791352,-0.234720132968122,
-5.11972100561116));
#27351=CARTESIAN_POINT('Ctrl Pts',(-0.253021752414184,-0.151060417405737,
-5.12501620075266));
#27352=CARTESIAN_POINT('Ctrl Pts',(-0.279955299859418,-0.105947518273335,
-5.12787159659879));
#27353=CARTESIAN_POINT('Ctrl Pts',(-0.293628717093803,-0.0529179843639099,
-5.13072699244491));
#27354=CARTESIAN_POINT('Ctrl Pts',(-0.293729850984995,6.28784883607292E-5,
-5.13358238829104));
#27355=CARTESIAN_POINT('Ctrl Pts',(-0.29372088508174,3.30216514158299E-5,
-5.14801761170896));
#27356=CARTESIAN_POINT('Ctrl Pts',(-0.293669708642092,-0.0511078051506823,
-5.14526159378119));
#27357=CARTESIAN_POINT('Ctrl Pts',(-0.280982886140013,-0.102272398931093,
-5.14250557585341));
#27358=CARTESIAN_POINT('Ctrl Pts',(-0.255806892924437,-0.146294507019556,
-5.13974955792564));
#27359=CARTESIAN_POINT('Ctrl Pts',(-0.207435728276266,-0.23087510808157,
-5.13445436278414));
#27360=CARTESIAN_POINT('Ctrl Pts',(-0.112961109491914,-0.28908940596213,
-5.12915916764264));
#27361=CARTESIAN_POINT('Ctrl Pts',(-0.0156634967798184,-0.294268421887871,
-5.12386397250114));
#27362=CARTESIAN_POINT('Ctrl Pts',(0.0816341159322764,-0.299447437813612,
-5.11856877735963));
#27363=CARTESIAN_POINT('Ctrl Pts',(0.181754722572115,-0.251591171784534,
-5.11327358221813));
#27364=CARTESIAN_POINT('Ctrl Pts',(0.238831338043824,-0.172623408667382,
-5.10797838707663));
#27365=CARTESIAN_POINT('Ctrl Pts',(0.295907953515533,-0.0936556455502302,
-5.10268319193513));
#27366=CARTESIAN_POINT('Ctrl Pts',(0.309940577819113,0.0164236146549957,
-5.09738799679363));
#27367=CARTESIAN_POINT('Ctrl Pts',(0.27450062256113,0.107185155060303,-5.09209280165212));
#27368=CARTESIAN_POINT('Ctrl Pts',(0.239060667303148,0.197946695465609,
-5.08679760651062));
#27369=CARTESIAN_POINT('Ctrl Pts',(0.154148132483604,0.269390516070998,
-5.08150241136912));
#27370=CARTESIAN_POINT('Ctrl Pts',(0.0586629219258051,0.28878696446148,
-5.07620721622761));
#27371=CARTESIAN_POINT('Ctrl Pts',(-0.0368222886319945,0.308183412851963,
-5.07091202108611));
#27372=CARTESIAN_POINT('Ctrl Pts',(-0.14288017492805,0.275532489027539,
-5.06561682594461));
#27373=CARTESIAN_POINT('Ctrl Pts',(-0.210923781156748,0.20579214706662,
-5.06032163080311));
#27374=CARTESIAN_POINT('Ctrl Pts',(-0.26362626632805,0.151775472440597,
-5.05622029110506));
#27375=CARTESIAN_POINT('Ctrl Pts',(-0.293523528977382,0.0755084110569016,
-5.05211895140701));
#27376=CARTESIAN_POINT('Ctrl Pts',(-0.294223320968512,-0.000268522322062943,
-5.04801761170896));
#27377=CARTESIAN_POINT('Origin',(0.,0.,-4.78));
#27378=CARTESIAN_POINT('',(-0.294651137856664,9.05457447918836E-5,-4.93358238829104));
#27379=CARTESIAN_POINT('',(-0.294623644711037,0.000121576380800716,-4.94801761170896));
#27380=CARTESIAN_POINT('',(-0.2942,-3.60291088309151E-17,-4.78));
#27381=CARTESIAN_POINT('Ctrl Pts',(-0.294651137856664,9.05457447918836E-5,
-4.93358238829104));
#27382=CARTESIAN_POINT('Ctrl Pts',(-0.294671139319386,0.00504055750254152,
-4.93385131741355));
#27383=CARTESIAN_POINT('Ctrl Pts',(-0.294557213003961,0.00998962927470263,
-4.93412024653607));
#27384=CARTESIAN_POINT('Ctrl Pts',(-0.294306471987783,0.0149317596968457,
-4.93438917565858));
#27385=CARTESIAN_POINT('Ctrl Pts',(-0.289369399356023,0.112241953384708,
-4.93968437080008));
#27386=CARTESIAN_POINT('Ctrl Pts',(-0.231390187092484,0.206861032339553,
-4.94497956594158));
#27387=CARTESIAN_POINT('Ctrl Pts',(-0.146930117175096,0.255442356645199,
-4.95027476108308));
#27388=CARTESIAN_POINT('Ctrl Pts',(-0.0624700472577058,0.304023680950845,
-4.95556995622458));
#27389=CARTESIAN_POINT('Ctrl Pts',(0.048470880313534,0.306567250607288,
-4.96086515136609));
#27390=CARTESIAN_POINT('Ctrl Pts',(0.13506870389667,0.261907812272208,-4.96616034650759));
#27391=CARTESIAN_POINT('Ctrl Pts',(0.221666527479803,0.217248373937128,
-4.9714555416491));
#27392=CARTESIAN_POINT('Ctrl Pts',(0.283921247074832,0.125385927610527,
-4.9767507367906));
#27393=CARTESIAN_POINT('Ctrl Pts',(0.293312896696289,0.028404252026281,
-4.9820459319321));
#27394=CARTESIAN_POINT('Ctrl Pts',(0.302704546317745,-0.0685774235579688,
-4.9873411270736));
#27395=CARTESIAN_POINT('Ctrl Pts',(0.259233125965623,-0.170678328399865,
-4.99263632221511));
#27396=CARTESIAN_POINT('Ctrl Pts',(0.182813646708123,-0.231124268476544,
-4.99793151735661));
#27397=CARTESIAN_POINT('Ctrl Pts',(0.106394167450625,-0.291570208553221,
-5.00322671249811));
#27398=CARTESIAN_POINT('Ctrl Pts',(-0.00297337071224937,-0.310361183864684,
-5.00852190763961));
#27399=CARTESIAN_POINT('Ctrl Pts',(-0.095185803094993,-0.278888722953621,
-5.01381710278111));
#27400=CARTESIAN_POINT('Ctrl Pts',(-0.187398235477738,-0.247416262042557,
-5.01911229792261));
#27401=CARTESIAN_POINT('Ctrl Pts',(-0.262455562080351,-0.165680364908966,
-5.02440749306412));
#27402=CARTESIAN_POINT('Ctrl Pts',(-0.285972720764702,-0.0711256625977863,
-5.02970268820562));
#27403=CARTESIAN_POINT('Ctrl Pts',(-0.291716262479935,-0.0480327845683877,
-5.03099592156743));
#27404=CARTESIAN_POINT('Ctrl Pts',(-0.294385578916972,-0.0241753010573829,
-5.03228915492924));
#27405=CARTESIAN_POINT('Ctrl Pts',(-0.294167685007082,-0.000269782114602712,
-5.03358238829104));
#27406=CARTESIAN_POINT('Ctrl Pts',(-0.294223320968512,-0.000268522322062943,
-5.04801761170896));
#27407=CARTESIAN_POINT('Ctrl Pts',(-0.29442702281703,-0.0223263646523878,
-5.04682375626551));
#27408=CARTESIAN_POINT('Ctrl Pts',(-0.292156738679848,-0.0443426770218096,
-5.04562990082206));
#27409=CARTESIAN_POINT('Ctrl Pts',(-0.28725480488683,-0.0657565686542278,
-5.0444360453786));
#27410=CARTESIAN_POINT('Ctrl Pts',(-0.265512896226875,-0.160735182316747,
-5.0391408502371));
#27411=CARTESIAN_POINT('Ctrl Pts',(-0.191999752745621,-0.243862649544373,
-5.0338456550956));
#27412=CARTESIAN_POINT('Ctrl Pts',(-0.100393019531007,-0.277056836914731,
-5.02855045995409));
#27413=CARTESIAN_POINT('Ctrl Pts',(-0.00878628631639407,-0.31025102428509,
-5.02325526481259));
#27414=CARTESIAN_POINT('Ctrl Pts',(0.10091403663158,-0.293511931798183,
-5.01796006967109));
#27415=CARTESIAN_POINT('Ctrl Pts',(0.178452330149845,-0.234508027828132,
-5.01266487452959));
#27416=CARTESIAN_POINT('Ctrl Pts',(0.255990623668112,-0.17550412385808,
-5.00736967938809));
#27417=CARTESIAN_POINT('Ctrl Pts',(0.30136688775667,-0.0742354084048829,
-5.00207448424658));
#27418=CARTESIAN_POINT('Ctrl Pts',(0.293793469418738,0.0229051648902689,
-4.99677928910508));
#27419=CARTESIAN_POINT('Ctrl Pts',(0.286220051080805,0.12004573818542,-4.99148409396357));
#27420=CARTESIAN_POINT('Ctrl Pts',(0.225696950316382,0.213058169322525,
-4.98618889882207));
#27421=CARTESIAN_POINT('Ctrl Pts',(0.139950848513885,0.259331851595582,
-4.98089370368057));
#27422=CARTESIAN_POINT('Ctrl Pts',(0.0542047467113887,0.305605533868638,
-4.97559850853907));
#27423=CARTESIAN_POINT('Ctrl Pts',(-0.0567643561291807,0.305140467277647,
-4.97030331339757));
#27424=CARTESIAN_POINT('Ctrl Pts',(-0.142119590786683,0.258149706888029,
-4.96500811825607));
#27425=CARTESIAN_POINT('Ctrl Pts',(-0.227474825444186,0.21115894649841,
-4.95971292311456));
#27426=CARTESIAN_POINT('Ctrl Pts',(-0.287216191918622,0.117642492310163,
-4.95441772797306));
#27427=CARTESIAN_POINT('Ctrl Pts',(-0.293975134848083,0.0204418527242618,
-4.94912253283156));
#27428=CARTESIAN_POINT('Ctrl Pts',(-0.294445252795243,0.0136810669591461,
-4.94875422579069));
#27429=CARTESIAN_POINT('Ctrl Pts',(-0.294659047538173,0.00690245750566513,
-4.94838591874983));
#27430=CARTESIAN_POINT('Ctrl Pts',(-0.294623644711037,0.000121576380800716,
-4.94801761170896));
#27431=CARTESIAN_POINT('Origin',(0.,0.,-4.78));
#27432=CARTESIAN_POINT('',(-0.293898321762298,0.000215997425517533,-4.83358238829104));
#27433=CARTESIAN_POINT('',(-0.293858731285566,0.00019623248150203,-4.84801761170896));
#27434=CARTESIAN_POINT('',(-0.2942,-3.60291088309151E-17,-4.78));
#27435=CARTESIAN_POINT('Ctrl Pts',(-0.293898321762298,0.000215997425517533,
-4.83358238829104));
#27436=CARTESIAN_POINT('Ctrl Pts',(-0.29412892854093,0.0341424934738597,
-4.83541347989787));
#27437=CARTESIAN_POINT('Ctrl Pts',(-0.288705448149838,0.0679975401570607,
-4.8372445715047));
#27438=CARTESIAN_POINT('Ctrl Pts',(-0.277305616806589,0.0997038203333129,
-4.83907566311153));
#27439=CARTESIAN_POINT('Ctrl Pts',(-0.244339307902389,0.191392810724597,
-4.84437085825304));
#27440=CARTESIAN_POINT('Ctrl Pts',(-0.161394882146101,0.265112424077647,
-4.84966605339454));
#27441=CARTESIAN_POINT('Ctrl Pts',(-0.0664706184897772,0.287090427877919,
-4.85496124853604));
#27442=CARTESIAN_POINT('Ctrl Pts',(0.0284536451665497,0.309068431678192,
-4.86025644367755));
#27443=CARTESIAN_POINT('Ctrl Pts',(0.135357746722915,0.279304825925683,
-4.86555163881905));
#27444=CARTESIAN_POINT('Ctrl Pts',(0.205267064497167,0.211434834249837,
-4.87084683396055));
#27445=CARTESIAN_POINT('Ctrl Pts',(0.275176382271419,0.143564842573991,
-4.87614202910205));
#27446=CARTESIAN_POINT('Ctrl Pts',(0.308090916263558,0.0375884649748095,
-4.88143722424355));
#27447=CARTESIAN_POINT('Ctrl Pts',(0.288931948008704,-0.0579446832887666,
-4.88673241938505));
#27448=CARTESIAN_POINT('Ctrl Pts',(0.269772979753852,-0.15347783155234,
-4.89202761452656));
#27449=CARTESIAN_POINT('Ctrl Pts',(0.198540509252008,-0.238567750480307,
-4.89732280966807));
#27450=CARTESIAN_POINT('Ctrl Pts',(0.107867365772809,-0.274233273515041,
-4.90261800480957));
#27451=CARTESIAN_POINT('Ctrl Pts',(0.01719422229361,-0.309898796549775,
-4.90791319995107));
#27452=CARTESIAN_POINT('Ctrl Pts',(-0.0929195941629457,-0.296139923691275,
-4.91320839509257));
#27453=CARTESIAN_POINT('Ctrl Pts',(-0.172029035891234,-0.239259833051586,
-4.91850359023407));
#27454=CARTESIAN_POINT('Ctrl Pts',(-0.247120715822662,-0.18526853356225,
-4.92352985625306));
#27455=CARTESIAN_POINT('Ctrl Pts',(-0.294277311952389,-0.0924248191183649,
-4.92855612227205));
#27456=CARTESIAN_POINT('Ctrl Pts',(-0.294651137856664,9.05457447918836E-5,
-4.93358238829104));
#27457=CARTESIAN_POINT('Ctrl Pts',(-0.294623644711037,0.000121576380800716,
-4.94801761170896));
#27458=CARTESIAN_POINT('Ctrl Pts',(-0.29415005678468,-0.0905870955125116,
-4.94309072360833));
#27459=CARTESIAN_POINT('Ctrl Pts',(-0.249083215497219,-0.181702277058098,
-4.93816383550769));
#27460=CARTESIAN_POINT('Ctrl Pts',(-0.176480470572474,-0.235995535462575,
-4.93323694740705));
#27461=CARTESIAN_POINT('Ctrl Pts',(-0.0984503439829113,-0.294347459079958,
-4.92794175226555));
#27462=CARTESIAN_POINT('Ctrl Pts',(0.0113864285807017,-0.310166481331168,
-4.92264655712404));
#27463=CARTESIAN_POINT('Ctrl Pts',(0.10271171802156,-0.27620563396283,-4.91735136198254));
#27464=CARTESIAN_POINT('Ctrl Pts',(0.194037007462415,-0.242244786594493,
-4.91205616684104));
#27465=CARTESIAN_POINT('Ctrl Pts',(0.266850813780515,-0.158504069606611,
-4.90676097169955));
#27466=CARTESIAN_POINT('Ctrl Pts',(0.287795870362606,-0.0633465567649832,
-4.90146577655804));
#27467=CARTESIAN_POINT('Ctrl Pts',(0.308740926944698,0.0318109560766487,
-4.89617058141654));
#27468=CARTESIAN_POINT('Ctrl Pts',(0.277817233790773,0.13838526477203,-4.89087538627503));
#27469=CARTESIAN_POINT('Ctrl Pts',(0.209191470674386,0.207552831464273,
-4.88558019113353));
#27470=CARTESIAN_POINT('Ctrl Pts',(0.140565707558001,0.276720398156514,
-4.88028499599203));
#27471=CARTESIAN_POINT('Ctrl Pts',(0.0342378744791568,0.308481222845622,
-4.87498980085053));
#27472=CARTESIAN_POINT('Ctrl Pts',(-0.0610814054568818,0.288285121293419,
-4.86969460570903));
#27473=CARTESIAN_POINT('Ctrl Pts',(-0.15640068539292,0.268089019741216,
-4.86439941056753));
#27474=CARTESIAN_POINT('Ctrl Pts',(-0.240711412186152,0.195935991947701,
-4.85910421542602));
#27475=CARTESIAN_POINT('Ctrl Pts',(-0.275389380700085,0.104880590432038,
-4.85380902028452));
#27476=CARTESIAN_POINT('Ctrl Pts',(-0.288031929203502,0.0716845187043262,
-4.85187855075933));
#27477=CARTESIAN_POINT('Ctrl Pts',(-0.294077722442252,0.0359761075925212,
-4.84994808123415));
#27478=CARTESIAN_POINT('Ctrl Pts',(-0.293858731285566,0.00019623248150203,
-4.84801761170896));
#27479=CARTESIAN_POINT('Origin',(0.,0.,-4.78));
#27480=CARTESIAN_POINT('',(-0.293869683561436,-0.000202171647430832,-4.73358238829104));
#27481=CARTESIAN_POINT('',(-0.29391040772598,-0.000221175939017525,-4.74801761170896));
#27482=CARTESIAN_POINT('',(-0.2942,-3.60291088309151E-17,-4.78));
#27483=CARTESIAN_POINT('Ctrl Pts',(-0.293869683561436,-0.000202171647430832,
-4.73358238829104));
#27484=CARTESIAN_POINT('Ctrl Pts',(-0.293472176975345,0.0626834963700132,
-4.73697564238219));
#27485=CARTESIAN_POINT('Ctrl Pts',(-0.273702122510387,0.125797236938147,
-4.74036889647334));
#27486=CARTESIAN_POINT('Ctrl Pts',(-0.236433629577098,0.175893137178628,
-4.7437621505645));
#27487=CARTESIAN_POINT('Ctrl Pts',(-0.178275903273585,0.254068116250875,
-4.749057345706));
#27488=CARTESIAN_POINT('Ctrl Pts',(-0.0775063189671733,0.300542303018127,
-4.7543525408475));
#27489=CARTESIAN_POINT('Ctrl Pts',(0.0197108303297479,0.29402506707635,
-4.759647735989));
#27490=CARTESIAN_POINT('Ctrl Pts',(0.11692797962667,0.287507831134573,-4.7649429311305));
#27491=CARTESIAN_POINT('Ctrl Pts',(0.210592693914104,0.227999172483765,
-4.77023812627201));
#27492=CARTESIAN_POINT('Ctrl Pts',(0.257795544270133,0.142761038998762,
-4.77553332141351));
#27493=CARTESIAN_POINT('Ctrl Pts',(0.304998394626161,0.0575229055137613,
-4.78082851655501));
#27494=CARTESIAN_POINT('Ctrl Pts',(0.305739381050789,-0.0534447028054307,
-4.78612371169651));
#27495=CARTESIAN_POINT('Ctrl Pts',(0.259679044820831,-0.139305601403824,
-4.79141890683801));
#27496=CARTESIAN_POINT('Ctrl Pts',(0.213618708590872,-0.225166500002218,
-4.79671410197952));
#27497=CARTESIAN_POINT('Ctrl Pts',(0.120757049706323,-0.28592068887981,
-4.80200929712102));
#27498=CARTESIAN_POINT('Ctrl Pts',(0.0236356034912526,-0.293735621178543,
-4.80730449226252));
#27499=CARTESIAN_POINT('Ctrl Pts',(-0.0734858427238168,-0.301550553477275,
-4.81259968740402));
#27500=CARTESIAN_POINT('Ctrl Pts',(-0.17486707626941,-0.25642622919715,
-4.81789488254553));
#27501=CARTESIAN_POINT('Ctrl Pts',(-0.234063597016152,-0.179034883342326,
-4.82319007768703));
#27502=CARTESIAN_POINT('Ctrl Pts',(-0.272789814139247,-0.128405656738881,
-4.8266541812217));
#27503=CARTESIAN_POINT('Ctrl Pts',(-0.293462054262629,-0.0639669710516069,
-4.83011828475637));
#27504=CARTESIAN_POINT('Ctrl Pts',(-0.293898321762298,0.000215997425517533,
-4.83358238829104));
#27505=CARTESIAN_POINT('Ctrl Pts',(-0.293858731285566,0.00019623248150203,
-4.84801761170896));
#27506=CARTESIAN_POINT('Ctrl Pts',(-0.29347703908839,-0.0621665558267297,
-4.84465288609264));
#27507=CARTESIAN_POINT('Ctrl Pts',(-0.27406356122904,-0.124746444585632,
-4.84128816047633));
#27508=CARTESIAN_POINT('Ctrl Pts',(-0.237376059777544,-0.174619172762435,
-4.83792343486001));
#27509=CARTESIAN_POINT('Ctrl Pts',(-0.179639560106439,-0.253105759203433,
-4.83262823971851));
#27510=CARTESIAN_POINT('Ctrl Pts',(-0.079121350529597,-0.30012115684762,
-4.82733304457701));
#27511=CARTESIAN_POINT('Ctrl Pts',(0.0181294350607954,-0.294126797208492,
-4.82203784943551));
#27512=CARTESIAN_POINT('Ctrl Pts',(0.115380220651189,-0.288132437569365,
-4.816742654294));
#27513=CARTESIAN_POINT('Ctrl Pts',(0.209363582255135,-0.229128320646921,
-4.8114474591525));
#27514=CARTESIAN_POINT('Ctrl Pts',(0.257024113092535,-0.144145255006,-4.806152264011));
#27515=CARTESIAN_POINT('Ctrl Pts',(0.304684643929936,-0.0591621893650789,
-4.80085706886949));
#27516=CARTESIAN_POINT('Ctrl Pts',(0.306022344000792,0.0517998249943176,
-4.795561873728));
#27517=CARTESIAN_POINT('Ctrl Pts',(0.260424389718913,0.13790716620713,-4.79026667858649));
#27518=CARTESIAN_POINT('Ctrl Pts',(0.214826435437034,0.224014507419941,
-4.78497148344499));
#27519=CARTESIAN_POINT('Ctrl Pts',(0.122292826802418,0.285267175486166,
-4.77967628830348));
#27520=CARTESIAN_POINT('Ctrl Pts',(0.0252148136341864,0.29360426159227,
-4.77438109316198));
#27521=CARTESIAN_POINT('Ctrl Pts',(-0.0718631995340452,0.301941347698375,
-4.76908589802048));
#27522=CARTESIAN_POINT('Ctrl Pts',(-0.173485617235893,0.25736285184436,
-4.76379070287898));
#27523=CARTESIAN_POINT('Ctrl Pts',(-0.233097448700031,0.180290955572612,
-4.75849550773748));
#27524=CARTESIAN_POINT('Ctrl Pts',(-0.272416526685478,0.129455478360035,
-4.75500287572798));
#27525=CARTESIAN_POINT('Ctrl Pts',(-0.293458791912228,0.0644836643687234,
-4.75151024371847));
#27526=CARTESIAN_POINT('Ctrl Pts',(-0.29391040772598,-0.000221175939017525,
-4.74801761170896));
#27527=CARTESIAN_POINT('Origin',(0.,0.,-4.78));
#27528=CARTESIAN_POINT('',(-0.294632262618422,-0.000112863968801113,-4.63358238829104));
#27529=CARTESIAN_POINT('',(-0.294657663022813,-8.13145974722069E-5,-4.64801761170896));
#27530=CARTESIAN_POINT('',(-0.2942,-3.60291088309151E-17,-4.78));
#27531=CARTESIAN_POINT('Ctrl Pts',(-0.294632262618422,-0.000112863968801113,
-4.63358238829104));
#27532=CARTESIAN_POINT('Ctrl Pts',(-0.294185344683986,0.0911139735210852,
-4.63853780486651));
#27533=CARTESIAN_POINT('Ctrl Pts',(-0.248524608202355,0.182726981672203,
-4.64349322144198));
#27534=CARTESIAN_POINT('Ctrl Pts',(-0.175208868908362,0.236941151253623,
-4.64844863801746));
#27535=CARTESIAN_POINT('Ctrl Pts',(-0.0968660816587778,0.29487262946458,
-4.65374383315896));
#27536=CARTESIAN_POINT('Ctrl Pts',(0.0130541738897331,0.310100780275279,
-4.65903902830046));
#27537=CARTESIAN_POINT('Ctrl Pts',(0.104195523638138,0.275649323879661,
-4.66433422344196));
#27538=CARTESIAN_POINT('Ctrl Pts',(0.195336873386545,0.241197867484043,
-4.66962941858346));
#27539=CARTESIAN_POINT('Ctrl Pts',(0.267699317334844,0.157066803882104,
-4.67492461372497));
#27540=CARTESIAN_POINT('Ctrl Pts',(0.288132365793964,0.0617980313886571,
-4.68021980886647));
#27541=CARTESIAN_POINT('Ctrl Pts',(0.308565414253084,-0.0334707411047907,
-4.68551500400797));
#27542=CARTESIAN_POINT('Ctrl Pts',(0.277069067223022,-0.139877222489745,
-4.69081019914947));
#27543=CARTESIAN_POINT('Ctrl Pts',(0.208072347142677,-0.208674759508852,
-4.69610539429097));
#27544=CARTESIAN_POINT('Ctrl Pts',(0.139075627062335,-0.277472296527957,
-4.70140058943247));
#27545=CARTESIAN_POINT('Ctrl Pts',(0.0325785339317089,-0.308660889181219,
-4.70669578457398));
#27546=CARTESIAN_POINT('Ctrl Pts',(-0.0626307681807567,-0.287952502643454,
-4.71199097971548));
#27547=CARTESIAN_POINT('Ctrl Pts',(-0.157840070293225,-0.267244116105689,
-4.71728617485699));
#27548=CARTESIAN_POINT('Ctrl Pts',(-0.241761581387535,-0.194638750376895,
-4.72258136999848));
#27549=CARTESIAN_POINT('Ctrl Pts',(-0.275949402784381,-0.103398181823877,
-4.72787656513999));
#27550=CARTESIAN_POINT('Ctrl Pts',(-0.288229067499113,-0.0706261728325144,
-4.72977850619034));
#27551=CARTESIAN_POINT('Ctrl Pts',(-0.294092488595649,-0.0354499987385414,
-4.73168044724069));
#27552=CARTESIAN_POINT('Ctrl Pts',(-0.293869683561436,-0.000202171647430832,
-4.73358238829104));
#27553=CARTESIAN_POINT('Ctrl Pts',(-0.29391040772598,-0.000221175939017525,
-4.74801761170896));
#27554=CARTESIAN_POINT('Ctrl Pts',(-0.294143488684261,-0.0336156358429093,
-4.74621504857697));
#27555=CARTESIAN_POINT('Ctrl Pts',(-0.28889196467631,-0.0669389836045177,
-4.74441248544497));
#27556=CARTESIAN_POINT('Ctrl Pts',(-0.277837748893218,-0.0982111732019241,
-4.74260992231297));
#27557=CARTESIAN_POINT('Ctrl Pts',(-0.245364972395839,-0.190076109015233,
-4.73731472717147));
#27558=CARTESIAN_POINT('Ctrl Pts',(-0.162818174174651,-0.264240683952366,
-4.73201953202996));
#27559=CARTESIAN_POINT('Ctrl Pts',(-0.0680134731165798,-0.286728820885466,
-4.72672433688846));
#27560=CARTESIAN_POINT('Ctrl Pts',(0.02679122794149,-0.309216957818565,
-4.72142914174696));
#27561=CARTESIAN_POINT('Ctrl Pts',(0.133853831836441,-0.280028656747631,
-4.71613394660546));
#27562=CARTESIAN_POINT('Ctrl Pts',(0.20412710421781,-0.21253558425685,-4.71083875146396));
#27563=CARTESIAN_POINT('Ctrl Pts',(0.274400376599178,-0.145042511766069,
-4.70554355632246));
#27564=CARTESIAN_POINT('Ctrl Pts',(0.307884317466962,-0.0392446678554377,
-4.70024836118095));
#27565=CARTESIAN_POINT('Ctrl Pts',(0.289239353198137,0.0563901215929949,
-4.69495316603945));
#27566=CARTESIAN_POINT('Ctrl Pts',(0.27059438892931,0.15202491104143,-4.68965797089795));
#27567=CARTESIAN_POINT('Ctrl Pts',(0.199820519523876,0.237496646027665,
-4.68436277575645));
#27568=CARTESIAN_POINT('Ctrl Pts',(0.109340481141167,0.273649243440517,
-4.67906758061494));
#27569=CARTESIAN_POINT('Ctrl Pts',(0.0188604427584614,0.309801840853368,
-4.67377238547344));
#27570=CARTESIAN_POINT('Ctrl Pts',(-0.0913257646015185,0.296635300692835,
-4.66847719033194));
#27571=CARTESIAN_POINT('Ctrl Pts',(-0.170739929705677,0.240181443196284,
-4.66318199519044));
#27572=CARTESIAN_POINT('Ctrl Pts',(-0.246548709887166,0.186290577911231,
-4.65812720069661));
#27573=CARTESIAN_POINT('Ctrl Pts',(-0.29431610970276,0.0929536427050627,
-4.65307240620278));
#27574=CARTESIAN_POINT('Ctrl Pts',(-0.294657663022813,-8.13145974722069E-5,
-4.64801761170896));
#27575=CARTESIAN_POINT('Origin',(0.,0.,-4.78));
#27576=CARTESIAN_POINT('',(-0.294207300827486,0.000269263671129533,-4.53358238829104));
#27577=CARTESIAN_POINT('',(-0.294151842938781,0.000269461638096479,-4.54801761170896));
#27578=CARTESIAN_POINT('',(-0.2942,-3.60291088309151E-17,-4.78));
#27579=CARTESIAN_POINT('Ctrl Pts',(-0.294207300827486,0.000269263671129533,
-4.53358238829104));
#27580=CARTESIAN_POINT('Ctrl Pts',(-0.294415377118081,0.0228573529575127,
-4.53480477220933));
#27581=CARTESIAN_POINT('Ctrl Pts',(-0.29203396319701,0.0454020295514724,
-4.53602715612762));
#27582=CARTESIAN_POINT('Ctrl Pts',(-0.286897060561383,0.0673003234968311,
-4.5372495400459));
#27583=CARTESIAN_POINT('Ctrl Pts',(-0.264644721119102,0.162160651722523,
-4.54254473518741));
#27584=CARTESIAN_POINT('Ctrl Pts',(-0.190685622245191,0.244891606332771,
-4.54783993032891));
#27585=CARTESIAN_POINT('Ctrl Pts',(-0.0989017089218338,0.277592703207201,
-4.55313512547041));
#27586=CARTESIAN_POINT('Ctrl Pts',(-0.00711779559847499,0.310293800081631,
-4.55843032061192));
#27587=CARTESIAN_POINT('Ctrl Pts',(0.102490932174331,0.292965039220241,
-4.56372551575342));
#27588=CARTESIAN_POINT('Ctrl Pts',(0.179710816570699,0.233545026299069,
-4.56902071089492));
#27589=CARTESIAN_POINT('Ctrl Pts',(0.256930700967065,0.174125013377898,
-4.57431590603642));
#27590=CARTESIAN_POINT('Ctrl Pts',(0.301761741986994,0.0726137483969471,
-4.57961110117793));
#27591=CARTESIAN_POINT('Ctrl Pts',(0.293666062770727,-0.0244846988602953,
-4.58490629631943));
#27592=CARTESIAN_POINT('Ctrl Pts',(0.285570383554461,-0.12158314611754,
-4.59020149146093));
#27593=CARTESIAN_POINT('Ctrl Pts',(0.224547984101994,-0.214268775651076,
-4.59549668660243));
#27594=CARTESIAN_POINT('Ctrl Pts',(0.138554283184103,-0.260080694233308,
-4.60079188174393));
#27595=CARTESIAN_POINT('Ctrl Pts',(0.0525605822662109,-0.30589261281554,
-4.60608707688543));
#27596=CARTESIAN_POINT('Ctrl Pts',(-0.0584044201171068,-0.304830820446466,
-4.61138227202694));
#27597=CARTESIAN_POINT('Ctrl Pts',(-0.14350573323524,-0.257381742612324,
-4.61667746716844));
#27598=CARTESIAN_POINT('Ctrl Pts',(-0.22860704635337,-0.209932664778183,
-4.62197266230994));
#27599=CARTESIAN_POINT('Ctrl Pts',(-0.287844670206317,-0.116096301478976,
-4.62726785745144));
#27600=CARTESIAN_POINT('Ctrl Pts',(-0.294080822657462,-0.0188607170237647,
-4.63256305259294));
#27601=CARTESIAN_POINT('Ctrl Pts',(-0.294480979947379,-0.0126213686011803,
-4.63290283115898));
#27602=CARTESIAN_POINT('Ctrl Pts',(-0.294662906487123,-0.00636802406559657,
-4.63324260972501));
#27603=CARTESIAN_POINT('Ctrl Pts',(-0.294632262618422,-0.000112863968801113,
-4.63358238829104));
#27604=CARTESIAN_POINT('Ctrl Pts',(-0.294657663022813,-8.13145974722069E-5,
-4.64801761170896));
#27605=CARTESIAN_POINT('Ctrl Pts',(-0.294673906935292,-0.00450595817486475,
-4.64777721106128));
#27606=CARTESIAN_POINT('Ctrl Pts',(-0.294582880583495,-0.00892991872281405,
-4.6475368104136));
#27607=CARTESIAN_POINT('Ctrl Pts',(-0.294382498755337,-0.0133489204924204,
-4.64729640976593));
#27608=CARTESIAN_POINT('Ctrl Pts',(-0.289968779852495,-0.110684251851997,
-4.64200121462443));
#27609=CARTESIAN_POINT('Ctrl Pts',(-0.232499219198468,-0.205613739738578,
-4.63670601948293));
#27610=CARTESIAN_POINT('Ctrl Pts',(-0.148301618536078,-0.254648540524639,
-4.63141082434142));
#27611=CARTESIAN_POINT('Ctrl Pts',(-0.0641040178736896,-0.303683341310699,
-4.62611562919992));
#27612=CARTESIAN_POINT('Ctrl Pts',(0.0468216227970628,-0.306823454996241,
-4.62082043405841));
#27613=CARTESIAN_POINT('Ctrl Pts',(0.133658345028275,-0.262630341080485,
-4.61552523891691));
#27614=CARTESIAN_POINT('Ctrl Pts',(0.220495067259488,-0.218437227164728,
-4.61023004377541));
#27615=CARTESIAN_POINT('Ctrl Pts',(0.283242871051162,-0.126910885647671,
-4.60493484863391));
#27616=CARTESIAN_POINT('Ctrl Pts',(0.293155900001679,-0.029981119824895,
-4.59963965349241));
#27617=CARTESIAN_POINT('Ctrl Pts',(0.303068928952196,0.0669486459978793,
-4.59434445835091));
#27618=CARTESIAN_POINT('Ctrl Pts',(0.260147183061562,0.16928183612637,-4.5890492632094));
#27619=CARTESIAN_POINT('Ctrl Pts',(0.184053858000735,0.230137842622187,
-4.5837540680679));
#27620=CARTESIAN_POINT('Ctrl Pts',(0.107960532939904,0.290993849118007,
-4.5784588729264));
#27621=CARTESIAN_POINT('Ctrl Pts',(-0.00130437129112189,0.310372671981147,
-4.5731636777849));
#27622=CARTESIAN_POINT('Ctrl Pts',(-0.0936847083897634,0.279396536602861,
-4.5678684826434));
#27623=CARTESIAN_POINT('Ctrl Pts',(-0.186065045488401,0.248420401224577,
-4.56257328750189));
#27624=CARTESIAN_POINT('Ctrl Pts',(-0.261560815454657,0.167089307604873,
-4.55727809236039));
#27625=CARTESIAN_POINT('Ctrl Pts',(-0.285586097646837,0.0726624392833101,
-4.55198289721889));
#27626=CARTESIAN_POINT('Ctrl Pts',(-0.291583176180787,0.0490920462069799,
-4.55066113538224));
#27627=CARTESIAN_POINT('Ctrl Pts',(-0.294373241412294,0.024705684106633,
-4.5493393735456));
#27628=CARTESIAN_POINT('Ctrl Pts',(-0.294151842938781,0.000269461638096479,
-4.54801761170896));
#27629=CARTESIAN_POINT('Origin',(0.,0.,-4.78));
#27630=CARTESIAN_POINT('',(-0.293722896168541,-4.16502199041546E-5,-4.43358238829104));
#27631=CARTESIAN_POINT('',(-0.293733435156352,-7.13230564683106E-5,-4.44801761170896));
#27632=CARTESIAN_POINT('',(-0.2942,-3.60291088309151E-17,-4.78));
#27633=CARTESIAN_POINT('Ctrl Pts',(-0.293722896168541,-4.16502199041546E-5,
-4.43358238829104));
#27634=CARTESIAN_POINT('Ctrl Pts',(-0.293657654434464,0.0516276781612295,
-4.43636693469365));
#27635=CARTESIAN_POINT('Ctrl Pts',(-0.280691921537164,0.103327620603503,
-4.43915148109626));
#27636=CARTESIAN_POINT('Ctrl Pts',(-0.25501651195302,0.147667990887853,
-4.44193602749886));
#27637=CARTESIAN_POINT('Ctrl Pts',(-0.206191215323489,0.23198725850077,
-4.44723122264037));
#27638=CARTESIAN_POINT('Ctrl Pts',(-0.111404912997885,0.28969268327525,
-4.45252641778187));
#27639=CARTESIAN_POINT('Ctrl Pts',(-0.0140808528166932,0.294348410027122,
-4.45782161292337));
#27640=CARTESIAN_POINT('Ctrl Pts',(0.0832432073645018,0.299004136778995,
-4.46311680806487));
#27641=CARTESIAN_POINT('Ctrl Pts',(0.183105025401282,0.250610165508259,
-4.46841200320637));
#27642=CARTESIAN_POINT('Ctrl Pts',(0.239756171741916,0.171336613171852,
-4.47370719834788));
#27643=CARTESIAN_POINT('Ctrl Pts',(0.296407318082549,0.0920630608354474,
-4.47900239348938));
#27644=CARTESIAN_POINT('Ctrl Pts',(0.309847792727033,-0.0180900725666295,
-4.48429758863088));
#27645=CARTESIAN_POINT('Ctrl Pts',(0.273920281303337,-0.108659727554603,
-4.48959278377238));
#27646=CARTESIAN_POINT('Ctrl Pts',(0.237992769879641,-0.199229382542577,
-4.49488797891389));
#27647=CARTESIAN_POINT('Ctrl Pts',(0.152697272387766,-0.270215559116452,
-4.50018317405539));
#27648=CARTESIAN_POINT('Ctrl Pts',(0.0571091344883531,-0.289098259523525,
-4.50547836919689));
#27649=CARTESIAN_POINT('Ctrl Pts',(-0.0384790034110612,-0.307980959930598,
-4.5107735643384));
#27650=CARTESIAN_POINT('Ctrl Pts',(-0.144359781718014,-0.274760184170866,
-4.5160687594799));
#27651=CARTESIAN_POINT('Ctrl Pts',(-0.212027380866164,-0.204654945370432,
-4.5213639546214));
#27652=CARTESIAN_POINT('Ctrl Pts',(-0.264074066567786,-0.150733343661248,
-4.52543676584461));
#27653=CARTESIAN_POINT('Ctrl Pts',(-0.293514019904086,-0.0749910716295408,
-4.52950957706782));
#27654=CARTESIAN_POINT('Ctrl Pts',(-0.294207300827486,0.000269263671129533,
-4.53358238829104));
#27655=CARTESIAN_POINT('Ctrl Pts',(-0.294151842938781,0.000269461638096479,
-4.54801761170896));
#27656=CARTESIAN_POINT('Ctrl Pts',(-0.293486282741844,-0.0731898390541624,
-4.5440441784041));
#27657=CARTESIAN_POINT('Ctrl Pts',(-0.26560605257346,-0.147099729093613,
-4.54007074509924));
#27658=CARTESIAN_POINT('Ctrl Pts',(-0.215823605232151,-0.200647503538783,
-4.53609731179438));
#27659=CARTESIAN_POINT('Ctrl Pts',(-0.149481036207181,-0.27200793501589,
-4.53080211665288));
#27660=CARTESIAN_POINT('Ctrl Pts',(-0.0442411037391331,-0.307206154946681,
-4.52550692151137));
#27661=CARTESIAN_POINT('Ctrl Pts',(0.0516839551909757,-0.290117248759129,
-4.52021172636987));
#27662=CARTESIAN_POINT('Ctrl Pts',(0.147609014121084,-0.273028342571577,
-4.51491653122837));
#27663=CARTESIAN_POINT('Ctrl Pts',(0.234219199513256,-0.203652310265684,
-4.50962133608687));
#27664=CARTESIAN_POINT('Ctrl Pts',(0.271836884394817,-0.113771514599516,
-4.50432614094537));
#27665=CARTESIAN_POINT('Ctrl Pts',(0.309454569276379,-0.0238907189333472,
-4.49903094580387));
#27666=CARTESIAN_POINT('Ctrl Pts',(0.298079753647327,0.0864948400930953,
-4.49373575066236));
#27667=CARTESIAN_POINT('Ctrl Pts',(0.242923437684707,0.166815624793344,
-4.48844055552086));
#27668=CARTESIAN_POINT('Ctrl Pts',(0.187767121722086,0.247136409493592,
-4.48314536037936));
#27669=CARTESIAN_POINT('Ctrl Pts',(0.0888293054258945,0.297392419867646,
-4.47785016523786));
#27670=CARTESIAN_POINT('Ctrl Pts',(-0.00856488286340162,0.294560506574261,
-4.47255497009635));
#27671=CARTESIAN_POINT('Ctrl Pts',(-0.105959071152695,0.291728593280876,
-4.46725977495485));
#27672=CARTESIAN_POINT('Ctrl Pts',(-0.201809631435093,0.235808756320058,
-4.46196457981334));
#27673=CARTESIAN_POINT('Ctrl Pts',(-0.252205760855412,0.152418842152444,
-4.45666938467184));
#27674=CARTESIAN_POINT('Ctrl Pts',(-0.279653025674511,0.107002158694258,
-4.45378546035088));
#27675=CARTESIAN_POINT('Ctrl Pts',(-0.293617493229099,0.0534372380940554,
-4.45090153602992));
#27676=CARTESIAN_POINT('Ctrl Pts',(-0.293733435156352,-7.13230564683106E-5,
-4.44801761170896));
#27677=CARTESIAN_POINT('Origin',(0.,0.,-4.78));
#27678=CARTESIAN_POINT('',(-0.294360370562084,-0.000249476265296811,-4.33358238829104));
#27679=CARTESIAN_POINT('',(-0.294413795075237,-0.00023539599080995,-4.34801761170896));
#27680=CARTESIAN_POINT('',(-0.2942,-3.60291088309151E-17,-4.78));
#27681=CARTESIAN_POINT('Ctrl Pts',(-0.294360370562084,-0.000249476265296811,
-4.33358238829104));
#27682=CARTESIAN_POINT('Ctrl Pts',(-0.293636096245715,0.0799648134312458,
-4.33792909717797));
#27683=CARTESIAN_POINT('Ctrl Pts',(-0.259626145442727,0.160719405307108,
-4.3422758060649));
#27684=CARTESIAN_POINT('Ctrl Pts',(-0.201183530857245,0.215324043741873,
-4.34662251495182));
#27685=CARTESIAN_POINT('Ctrl Pts',(-0.129988275582514,0.281843846117607,
-4.35191771009333));
#27686=CARTESIAN_POINT('Ctrl Pts',(-0.02253420186159,0.30955631980262,-4.35721290523483));
#27687=CARTESIAN_POINT('Ctrl Pts',(0.0719521168432027,0.285765900315839,
-4.36250810037633));
#27688=CARTESIAN_POINT('Ctrl Pts',(0.166438435547995,0.261975480829059,
-4.36780329551783));
#27689=CARTESIAN_POINT('Ctrl Pts',(0.247956999236658,0.186682168170484,
-4.37309849065933));
#27690=CARTESIAN_POINT('Ctrl Pts',(0.279162741081986,0.0943791337803656,
-4.37839368580084));
#27691=CARTESIAN_POINT('Ctrl Pts',(0.310368482927314,0.00207609939024855,
-4.38368888094234));
#27692=CARTESIAN_POINT('Ctrl Pts',(0.29126140292931,-0.107236656731413,
-4.38898407608384));
#27693=CARTESIAN_POINT('Ctrl Pts',(0.230594785580612,-0.183481066501619,
-4.39427927122535));
#27694=CARTESIAN_POINT('Ctrl Pts',(0.169928168231914,-0.259725476271827,
-4.39957446636685));
#27695=CARTESIAN_POINT('Ctrl Pts',(0.067702013532521,-0.302901539690579,
-4.40486966150834));
#27696=CARTESIAN_POINT('Ctrl Pts',(-0.0292521053642755,-0.293229553819695,
-4.41016485664985));
#27697=CARTESIAN_POINT('Ctrl Pts',(-0.126206224261071,-0.283557567948812,
-4.41546005179135));
#27698=CARTESIAN_POINT('Ctrl Pts',(-0.217888307355266,-0.221037532788297,
-4.42075524693286));
#27699=CARTESIAN_POINT('Ctrl Pts',(-0.262297203435638,-0.134310959982362,
-4.42605044207436));
#27700=CARTESIAN_POINT('Ctrl Pts',(-0.283353110906546,-0.093190669827754,
-4.42856109081325));
#27701=CARTESIAN_POINT('Ctrl Pts',(-0.293781720498863,-0.0466286038501627,
-4.43107173955215));
#27702=CARTESIAN_POINT('Ctrl Pts',(-0.293722896168541,-4.16502199041546E-5,
-4.43358238829104));
#27703=CARTESIAN_POINT('Ctrl Pts',(-0.293733435156352,-7.13230564683106E-5,
-4.44801761170896));
#27704=CARTESIAN_POINT('Ctrl Pts',(-0.29383037507396,-0.0448102335797182,
-4.44560634088842));
#27705=CARTESIAN_POINT('Ctrl Pts',(-0.284246145997896,-0.0895097445761582,
-4.44319507006788));
#27706=CARTESIAN_POINT('Ctrl Pts',(-0.264766978775821,-0.129374248603317,
-4.44078379924734));
#27707=CARTESIAN_POINT('Ctrl Pts',(-0.221990368717675,-0.216917433817043,
-4.43548860410584));
#27708=CARTESIAN_POINT('Ctrl Pts',(-0.131495450043148,-0.281143812870087,
-4.43019340896433));
#27709=CARTESIAN_POINT('Ctrl Pts',(-0.0347395133680276,-0.292630168408354,
-4.42489821382283));
#27710=CARTESIAN_POINT('Ctrl Pts',(0.0620164233070968,-0.304116523946622,
-4.41960301868133));
#27711=CARTESIAN_POINT('Ctrl Pts',(0.165033377982814,-0.262862855970111,
-4.41430782353983));
#27712=CARTESIAN_POINT('Ctrl Pts',(0.227117498331296,-0.187768184747797,
-4.40901262839833));
#27713=CARTESIAN_POINT('Ctrl Pts',(0.289201618679778,-0.112673513525485,
-4.40371743325683));
#27714=CARTESIAN_POINT('Ctrl Pts',(0.310352904701023,-0.00373783905737107,
-4.39842223811532));
#27715=CARTESIAN_POINT('Ctrl Pts',(0.280881585694931,0.0891335182142501,
-4.39312704297382));
#27716=CARTESIAN_POINT('Ctrl Pts',(0.25141026668884,0.18200487548587,-4.38783184783232));
#27717=CARTESIAN_POINT('Ctrl Pts',(0.171316342655413,0.258811915561,-4.38253665269081));
#27718=CARTESIAN_POINT('Ctrl Pts',(0.0772922283053036,0.284368002235396,
-4.37724145754931));
#27719=CARTESIAN_POINT('Ctrl Pts',(-0.0167318860448084,0.309924088909792,
-4.37194626240781));
#27720=CARTESIAN_POINT('Ctrl Pts',(-0.124686190711601,0.284229222183455,
-4.36665106726631));
#27721=CARTESIAN_POINT('Ctrl Pts',(-0.197114947766929,0.219054665822461,
-4.36135587212481));
#27722=CARTESIAN_POINT('Ctrl Pts',(-0.257929428151737,0.164331142452089,
-4.35690978531953));
#27723=CARTESIAN_POINT('Ctrl Pts',(-0.293698234899642,0.081774257223651,
-4.35246369851424));
#27724=CARTESIAN_POINT('Ctrl Pts',(-0.294413795075237,-0.00023539599080995,
-4.34801761170896));
#27725=CARTESIAN_POINT('Origin',(0.,0.,-4.78));
#27726=CARTESIAN_POINT('',(-0.294529459134955,0.000188340711244316,-4.23358238829104));
#27727=CARTESIAN_POINT('',(-0.294482957137414,0.000210451042227086,-4.24801761170896));
#27728=CARTESIAN_POINT('',(-0.2942,-3.60291088309151E-17,-4.78));
#27729=CARTESIAN_POINT('Ctrl Pts',(-0.294529459134955,0.000188340711244316,
-4.23358238829104));
#27730=CARTESIAN_POINT('Ctrl Pts',(-0.294613692761748,0.0114962305757796,
-4.23419606452079));
#27731=CARTESIAN_POINT('Ctrl Pts',(-0.294018958340253,0.0227951767893906,
-4.23480974075053));
#27732=CARTESIAN_POINT('Ctrl Pts',(-0.292715655427141,0.0340117916229041,
-4.23542341698028));
#27733=CARTESIAN_POINT('Ctrl Pts',(-0.281469915541974,0.130795993929768,
-4.24071861212178));
#27734=CARTESIAN_POINT('Ctrl Pts',(-0.217468745024552,0.221450333756189,
-4.24601380726328));
#27735=CARTESIAN_POINT('Ctrl Pts',(-0.130032189295706,0.264444486893763,
-4.25130900240478));
#27736=CARTESIAN_POINT('Ctrl Pts',(-0.0425956335668611,0.307438640031337,
-4.25660419754628));
#27737=CARTESIAN_POINT('Ctrl Pts',(0.0682763073734012,0.302772606480067,
-4.26189939268779));
#27738=CARTESIAN_POINT('Ctrl Pts',(0.151791275854399,0.252583977076999,
-4.26719458782929));
#27739=CARTESIAN_POINT('Ctrl Pts',(0.235306244335397,0.202395347673931,
-4.27248978297079));
#27740=CARTESIAN_POINT('Ctrl Pts',(0.291464240357126,0.106684122419057,
-4.27778497811229));
#27741=CARTESIAN_POINT('Ctrl Pts',(0.294538312665593,0.00929727237664749,
-4.28308017325379));
#27742=CARTESIAN_POINT('Ctrl Pts',(0.297612384974061,-0.0880895776657633,
-4.2883753683953));
#27743=CARTESIAN_POINT('Ctrl Pts',(0.24760253356927,-0.187152052495716,
-4.2936705635368));
#27744=CARTESIAN_POINT('Ctrl Pts',(0.167419138102454,-0.242507915537971,
-4.2989657586783));
#27745=CARTESIAN_POINT('Ctrl Pts',(0.0872357426356381,-0.297863778580225,
-4.30426095381981));
#27746=CARTESIAN_POINT('Ctrl Pts',(-0.0231211968932015,-0.309513029834782,
-4.30955614896131));
#27747=CARTESIAN_POINT('Ctrl Pts',(-0.113095253885456,-0.272118945408298,
-4.31485134410281));
#27748=CARTESIAN_POINT('Ctrl Pts',(-0.203069310877712,-0.234724860981814,
-4.32014653924431));
#27749=CARTESIAN_POINT('Ctrl Pts',(-0.272660485333381,-0.148287440874289,
-4.32544173438581));
#27750=CARTESIAN_POINT('Ctrl Pts',(-0.289987854146947,-0.0524051652872991,
-4.33073692952732));
#27751=CARTESIAN_POINT('Ctrl Pts',(-0.293091568119413,-0.0352305346983667,
-4.33168541578189));
#27752=CARTESIAN_POINT('Ctrl Pts',(-0.294518412945755,-0.0177528686425654,
-4.33263390203647));
#27753=CARTESIAN_POINT('Ctrl Pts',(-0.294360370562084,-0.000249476265296811,
-4.33358238829104));
#27754=CARTESIAN_POINT('Ctrl Pts',(-0.294413795075237,-0.00023539599080995,
-4.34801761170896));
#27755=CARTESIAN_POINT('Ctrl Pts',(-0.294550451901065,-0.0158975013982573,
-4.34716850337274));
#27756=CARTESIAN_POINT('Ctrl Pts',(-0.293408615057636,-0.0315396476654283,
-4.34631939503652));
#27757=CARTESIAN_POINT('Ctrl Pts',(-0.29091857628131,-0.0469641483070301,
-4.3454702867003));
#27758=CARTESIAN_POINT('Ctrl Pts',(-0.275390238296502,-0.143154160079883,
-4.34017509155879));
#27759=CARTESIAN_POINT('Ctrl Pts',(-0.207430352883024,-0.230879937629941,
-4.33487989641729));
#27760=CARTESIAN_POINT('Ctrl Pts',(-0.118172521364231,-0.269952781882628,
-4.32958470127579));
#27761=CARTESIAN_POINT('Ctrl Pts',(-0.0289146898454392,-0.309025626135314,
-4.32428950613429));
#27762=CARTESIAN_POINT('Ctrl Pts',(0.0816410877786669,-0.299445537090632,
-4.31899431099279));
#27763=CARTESIAN_POINT('Ctrl Pts',(0.162847293731964,-0.245601319572848,
-4.31369911585128));
#27764=CARTESIAN_POINT('Ctrl Pts',(0.244053499685263,-0.191757102055065,
-4.30840392070978));
#27765=CARTESIAN_POINT('Ctrl Pts',(0.295910133967752,-0.0936487560641784,
-4.30310872556828));
#27766=CARTESIAN_POINT('Ctrl Pts',(0.29466077368526,0.00377858478179017,
-4.29781353042678));
#27767=CARTESIAN_POINT('Ctrl Pts',(0.293411413402767,0.101205925627759,
-4.29251833528528));
#27768=CARTESIAN_POINT('Ctrl Pts',(0.239056058555293,0.19795226132881,-4.28722314014377));
#27769=CARTESIAN_POINT('Ctrl Pts',(0.156495839233253,0.24969641878575,-4.28192794500227));
#27770=CARTESIAN_POINT('Ctrl Pts',(0.0739356199112137,0.301440576242691,
-4.27663274986077));
#27771=CARTESIAN_POINT('Ctrl Pts',(-0.0368294638853918,0.308182555455522,
-4.27133755471927));
#27772=CARTESIAN_POINT('Ctrl Pts',(-0.125056007595323,0.266833738901338,
-4.26604235957776));
#27773=CARTESIAN_POINT('Ctrl Pts',(-0.213282551305254,0.225484922347155,
-4.26074716443626));
#27774=CARTESIAN_POINT('Ctrl Pts',(-0.278970554928511,0.13604531002596,
-4.25545196929476));
#27775=CARTESIAN_POINT('Ctrl Pts',(-0.292027205563913,0.0394887384235212,
-4.25015677415325));
#27776=CARTESIAN_POINT('Ctrl Pts',(-0.293785421955766,0.0264863726810973,
-4.24944372000516));
#27777=CARTESIAN_POINT('Ctrl Pts',(-0.294589248926741,0.0133549517223198,
-4.24873066585706));
#27778=CARTESIAN_POINT('Ctrl Pts',(-0.294482957137414,0.000210451042227086,
-4.24801761170896));
#27779=CARTESIAN_POINT('Origin',(0.,0.,-4.78));
#27780=CARTESIAN_POINT('',(-0.293780102848547,0.000137479377752783,-4.13358238829104));
#27781=CARTESIAN_POINT('',(-0.293756768933342,0.000110456432129071,-4.14801761170896));
#27782=CARTESIAN_POINT('',(-0.2942,-3.60291088309151E-17,-4.78));
#27783=CARTESIAN_POINT('Ctrl Pts',(-0.293780102848547,0.000137479377752783,
-4.13358238829104));
#27784=CARTESIAN_POINT('Ctrl Pts',(-0.293950256150424,0.0404921514148337,
-4.13575822700511));
#27785=CARTESIAN_POINT('Ctrl Pts',(-0.286209896249464,0.0807843543255878,
-4.13793406571917));
#27786=CARTESIAN_POINT('Ctrl Pts',(-0.270245791604979,0.1175009320021,-4.14010990443324));
#27787=CARTESIAN_POINT('Ctrl Pts',(-0.231395003260468,0.206855644954183,
-4.14540509957474));
#27788=CARTESIAN_POINT('Ctrl Pts',(-0.143838473188879,0.275033450718222,
-4.15070029471624));
#27789=CARTESIAN_POINT('Ctrl Pts',(-0.0476873652618052,0.29080091488151,
-4.15599548985774));
#27790=CARTESIAN_POINT('Ctrl Pts',(0.0484637426652683,0.306568379044798,
-4.16129068499924));
#27791=CARTESIAN_POINT('Ctrl Pts',(0.153209428447825,0.269925501607335,
-4.16658588014074));
#27792=CARTESIAN_POINT('Ctrl Pts',(0.218563878077358,0.197659019782356,
-4.17188107528225));
#27793=CARTESIAN_POINT('Ctrl Pts',(0.283918327706889,0.12539253795738,-4.17717627042375));
#27794=CARTESIAN_POINT('Ctrl Pts',(0.309881541183399,0.017502451744889,
-4.18247146556526));
#27795=CARTESIAN_POINT('Ctrl Pts',(0.284559320443789,-0.0765849205138502,
-4.18776666070676));
#27796=CARTESIAN_POINT('Ctrl Pts',(0.259237099704177,-0.170672292772595,
-4.19306185584826));
#27797=CARTESIAN_POINT('Ctrl Pts',(0.18262944474844,-0.250956951077586,
-4.19835705098976));
#27798=CARTESIAN_POINT('Ctrl Pts',(0.0898316500020959,-0.280659102042746,
-4.20365224613126));
#27799=CARTESIAN_POINT('Ctrl Pts',(-0.0029661447442441,-0.310361253007904,
-4.20894744127276));
#27800=CARTESIAN_POINT('Ctrl Pts',(-0.111954079281189,-0.289480896633235,
-4.21424263641427));
#27801=CARTESIAN_POINT('Ctrl Pts',(-0.187202891923205,-0.227583686052249,
-4.21953783155577));
#27802=CARTESIAN_POINT('Ctrl Pts',(-0.253730891374979,-0.172859930991974,
-4.22421935046753));
#27803=CARTESIAN_POINT('Ctrl Pts',(-0.293886870587892,-0.0860755516916222,
-4.22890086937928));
#27804=CARTESIAN_POINT('Ctrl Pts',(-0.294529459134955,0.000188340711244316,
-4.23358238829104));
#27805=CARTESIAN_POINT('Ctrl Pts',(-0.294482957137414,0.000210451042227086,
-4.24801761170896));
#27806=CARTESIAN_POINT('Ctrl Pts',(-0.293799917894968,-0.0842571248980618,
-4.24343547071556));
#27807=CARTESIAN_POINT('Ctrl Pts',(-0.255534008629857,-0.169264820971633,
-4.23885332972216));
#27808=CARTESIAN_POINT('Ctrl Pts',(-0.191432955524924,-0.224037212959682,
-4.23427118872875));
#27809=CARTESIAN_POINT('Ctrl Pts',(-0.117356757202993,-0.287333061856756,
-4.22897599358725));
#27810=CARTESIAN_POINT('Ctrl Pts',(-0.00877906291158649,-0.310251228767228,
-4.22368079844574));
#27811=CARTESIAN_POINT('Ctrl Pts',(0.0845588038301234,-0.282292504233761,
-4.21838560330424));
#27812=CARTESIAN_POINT('Ctrl Pts',(0.177896670571836,-0.254333779700292,
-4.21309040816274));
#27813=CARTESIAN_POINT('Ctrl Pts',(0.255994709763852,-0.175498163722882,
-4.20779521302124));
#27814=CARTESIAN_POINT('Ctrl Pts',(0.283074856132123,-0.081901618283934,
-4.20250001787973));
#27815=CARTESIAN_POINT('Ctrl Pts',(0.310155002500395,0.0116949271550137,
-4.19720482273823));
#27816=CARTESIAN_POINT('Ctrl Pts',(0.286217256044923,0.120052402055498,
-4.19190962759673));
#27817=CARTESIAN_POINT('Ctrl Pts',(0.222227913282986,0.193530369217956,
-4.18661443245523));
#27818=CARTESIAN_POINT('Ctrl Pts',(0.158238570521051,0.267008336380412,
-4.18131923731373));
#27819=CARTESIAN_POINT('Ctrl Pts',(0.0541976314526524,0.305606795804842,
-4.17602404217222));
#27820=CARTESIAN_POINT('Ctrl Pts',(-0.0422319465973879,0.291643124277504,
-4.17072884703072));
#27821=CARTESIAN_POINT('Ctrl Pts',(-0.138661524647431,0.277679452750165,
-4.16543365188922));
#27822=CARTESIAN_POINT('Ctrl Pts',(-0.227479741679115,0.211153650271055,
-4.16013845674772));
#27823=CARTESIAN_POINT('Ctrl Pts',(-0.267997433158201,0.12254233991714,
-4.15484326160622));
#27824=CARTESIAN_POINT('Ctrl Pts',(-0.285406900249956,0.0844682138934502,
-4.1525680449738));
#27825=CARTESIAN_POINT('Ctrl Pts',(-0.293899066372842,0.0423166349121218,
-4.15029282834138));
#27826=CARTESIAN_POINT('Ctrl Pts',(-0.293756768933342,0.000110456432129071,
-4.14801761170896));
#27827=CARTESIAN_POINT('Origin',(0.,0.,-4.78));
#27828=CARTESIAN_POINT('',(-0.294026166038071,-0.000255545996156264,-4.03358238829104));
#27829=CARTESIAN_POINT('',(-0.294077901483341,-0.000263827746408872,-4.04801761170896));
#27830=CARTESIAN_POINT('',(-0.2942,-3.60291088309151E-17,-4.78));
#27831=CARTESIAN_POINT('Ctrl Pts',(-0.294026166038071,-0.000255545996156264,
-4.03358238829104));
#27832=CARTESIAN_POINT('Ctrl Pts',(-0.293452221785546,0.0689262477218108,
-4.03732038948942));
#27833=CARTESIAN_POINT('Ctrl Pts',(-0.26906437292607,0.138472261120715,
-4.04105839068781));
#27834=CARTESIAN_POINT('Ctrl Pts',(-0.224512522408552,0.190875310567925,
-4.04479639188619));
#27835=CARTESIAN_POINT('Ctrl Pts',(-0.16140105457187,0.265108666339113,
-4.05009158702769));
#27836=CARTESIAN_POINT('Ctrl Pts',(-0.0578262408769573,0.304941029133992,
-4.05538678216919));
#27837=CARTESIAN_POINT('Ctrl Pts',(0.038762501456049,0.292124503221433,
-4.0606819773107));
#27838=CARTESIAN_POINT('Ctrl Pts',(0.135351243789059,0.279307977308873,
-4.0659771724522));
#27839=CARTESIAN_POINT('Ctrl Pts',(0.22495391476016,0.213842562688867,-4.07127236759371));
#27840=CARTESIAN_POINT('Ctrl Pts',(0.266521977893879,0.125719100381765,
-4.07656756273521));
#27841=CARTESIAN_POINT('Ctrl Pts',(0.308090041027596,0.0375956380746656,
-4.08186275787671));
#27842=CARTESIAN_POINT('Ctrl Pts',(0.301623496323935,-0.0731858719195301,
-4.08715795301821));
#27843=CARTESIAN_POINT('Ctrl Pts',(0.250084779981618,-0.155874499913395,
-4.09245314815971));
#27844=CARTESIAN_POINT('Ctrl Pts',(0.198546063639301,-0.238563127907258,
-4.09774834330121));
#27845=CARTESIAN_POINT('Ctrl Pts',(0.10193517565833,-0.293158873900794,
-4.10304353844272));
#27846=CARTESIAN_POINT('Ctrl Pts',(0.00451123819089411,-0.294650480453547,
-4.10833873358422));
#27847=CARTESIAN_POINT('Ctrl Pts',(-0.092912699276546,-0.296142087006301,
-4.11363392872572));
#27848=CARTESIAN_POINT('Ctrl Pts',(-0.191149686230449,-0.24452955411827,
-4.11892912386722));
#27849=CARTESIAN_POINT('Ctrl Pts',(-0.245195656398686,-0.16345747760419,
-4.12422431900872));
#27850=CARTESIAN_POINT('Ctrl Pts',(-0.277033698230241,-0.115698576146939,
-4.12734367543616));
#27851=CARTESIAN_POINT('Ctrl Pts',(-0.293536165284412,-0.0577163517827691,
-4.1304630318636));
#27852=CARTESIAN_POINT('Ctrl Pts',(-0.293780102848547,0.000137479377752783,
-4.13358238829104));
#27853=CARTESIAN_POINT('Ctrl Pts',(-0.293756768933342,0.000110456432129071,
-4.14801761170896));
#27854=CARTESIAN_POINT('Ctrl Pts',(-0.293567892321301,-0.0559113527195887,
-4.14499763319988));
#27855=CARTESIAN_POINT('Ctrl Pts',(-0.278166621949572,-0.112029356506533,
-4.14197765469079));
#27856=CARTESIAN_POINT('Ctrl Pts',(-0.248214382111388,-0.158835983847513,
-4.13895767618171));
#27857=CARTESIAN_POINT('Ctrl Pts',(-0.195696473658997,-0.240906179029544,
-4.13366248104021));
#27858=CARTESIAN_POINT('Ctrl Pts',(-0.0984434908277233,-0.294349751164889,
-4.1283672858987));
#27859=CARTESIAN_POINT('Ctrl Pts',(-0.00100871054776456,-0.294683273625728,
-4.1230720907572));
#27860=CARTESIAN_POINT('Ctrl Pts',(0.0964260697321914,-0.295016796086566,
-4.1177768956157));
#27861=CARTESIAN_POINT('Ctrl Pts',(0.194042647460834,-0.242240268872898,
-4.1124817004742));
#27862=CARTESIAN_POINT('Ctrl Pts',(0.247121176583794,-0.16053153377332,
-4.1071865053327));
#27863=CARTESIAN_POINT('Ctrl Pts',(0.300199705706755,-0.0788227986737399,
-4.1018913101912));
#27864=CARTESIAN_POINT('Ctrl Pts',(0.308740186224036,0.0318181443117522,
-4.09659611504969));
#27865=CARTESIAN_POINT('Ctrl Pts',(0.268830075995526,0.12070476167888,-4.09130091990819));
#27866=CARTESIAN_POINT('Ctrl Pts',(0.228919965767017,0.209591379046007,
-4.08600572476668));
#27867=CARTESIAN_POINT('Ctrl Pts',(0.140559264792717,0.27672367079477,-4.08071052962518));
#27868=CARTESIAN_POINT('Ctrl Pts',(0.0442275415712278,0.291347170602866,
-4.07541533448368));
#27869=CARTESIAN_POINT('Ctrl Pts',(-0.0521041816502612,0.305970670410962,
-4.07012013934218));
#27870=CARTESIAN_POINT('Ctrl Pts',(-0.156406927118939,0.268085378278393,
-4.06482494420068));
#27871=CARTESIAN_POINT('Ctrl Pts',(-0.220897799459659,0.195047203122207,
-4.05952974905918));
#27872=CARTESIAN_POINT('Ctrl Pts',(-0.267633740275297,0.142117110731031,
-4.05569236994244));
#27873=CARTESIAN_POINT('Ctrl Pts',(-0.293461411669798,0.0707255421157874,
-4.0518549908257));
#27874=CARTESIAN_POINT('Ctrl Pts',(-0.294077901483341,-0.000263827746408872,
-4.04801761170896));
#27875=CARTESIAN_POINT('Origin',(0.,0.,-4.78));
#27876=CARTESIAN_POINT('',(-0.294685005132684,1.71253444288745E-6,-3.93358238829104));
#27877=CARTESIAN_POINT('',(-0.294679608262217,3.58352270703291E-5,-3.94801761170896));
#27878=CARTESIAN_POINT('',(-0.2942,-3.60291088309151E-17,-4.78));
#27879=CARTESIAN_POINT('Ctrl Pts',(-0.294685000185643,1.71251697507702E-6,
-3.93358238829104));
#27880=CARTESIAN_POINT('Ctrl Pts',(-0.2946934016704,0.097528503871605,-3.93888255197374));
#27881=CARTESIAN_POINT('Ctrl Pts',(-0.241468922813224,0.195047402076887,
-3.94418271565645));
#27882=CARTESIAN_POINT('Ctrl Pts',(-0.159452677353124,0.247818684994796,
-3.94948287933915));
#27883=CARTESIAN_POINT('Ctrl Pts',(-0.0775133165175665,0.300540498441735,
-3.95477807448065));
#27884=CARTESIAN_POINT('Ctrl Pts',(0.0331638128330922,0.308598552980046,
-3.96007326962216));
#27885=CARTESIAN_POINT('Ctrl Pts',(0.121875599210725,0.268301314246642,
-3.96536846476366));
#27886=CARTESIAN_POINT('Ctrl Pts',(0.210587385588363,0.228004075513236,
-3.97066365990516));
#27887=CARTESIAN_POINT('Ctrl Pts',(0.277333828992975,0.139351543508113,
-3.97595885504666));
#27888=CARTESIAN_POINT('Ctrl Pts',(0.291537227113789,0.0429569795443333,
-3.98125405018816));
#27889=CARTESIAN_POINT('Ctrl Pts',(0.305740625234603,-0.0534375844194461,
-3.98654924532967));
#27890=CARTESIAN_POINT('Ctrl Pts',(0.267400978071619,-0.15757418034188,
-3.99184444047117));
#27891=CARTESIAN_POINT('Ctrl Pts',(0.194082342353633,-0.221746028815296,
-3.99713963561267));
#27892=CARTESIAN_POINT('Ctrl Pts',(0.120763706635648,-0.285917877288712,
-4.00243483075417));
#27893=CARTESIAN_POINT('Ctrl Pts',(0.0124660823626598,-0.31012497831311,
-4.00773002589568));
#27894=CARTESIAN_POINT('Ctrl Pts',(-0.0811975118224673,-0.283277639385434,
-4.01302522103718));
#27895=CARTESIAN_POINT('Ctrl Pts',(-0.174861106007593,-0.256430300457758,
-4.01832041617868));
#27896=CARTESIAN_POINT('Ctrl Pts',(-0.25389067010486,-0.17852852157801,
-4.02361561132018));
#27897=CARTESIAN_POINT('Ctrl Pts',(-0.282081391164271,-0.0852604577643881,
-4.02891080646168));
#27898=CARTESIAN_POINT('Ctrl Pts',(-0.290371627673553,-0.0578324857679226,
-4.0304680004048));
#27899=CARTESIAN_POINT('Ctrl Pts',(-0.294265262407036,-0.0290756197292115,
-4.03202519434792));
#27900=CARTESIAN_POINT('Ctrl Pts',(-0.294026166038071,-0.000255545996156264,
-4.03358238829104));
#27901=CARTESIAN_POINT('Ctrl Pts',(-0.294077901483341,-0.000263827746408872,
-4.04801761170896));
#27902=CARTESIAN_POINT('Ctrl Pts',(-0.294312105272423,-0.0272326097782939,
-4.04655979568419));
#27903=CARTESIAN_POINT('Ctrl Pts',(-0.290907751712052,-0.0541433452158874,
-4.04510197965943));
#27904=CARTESIAN_POINT('Ctrl Pts',(-0.283628919847751,-0.0799617726008578,
-4.04364416363466));
#27905=CARTESIAN_POINT('Ctrl Pts',(-0.257190168682364,-0.173741514987928,
-4.03834896849316));
#27906=CARTESIAN_POINT('Ctrl Pts',(-0.179633667138827,-0.253109941582263,
-4.03305377335166));
#27907=CARTESIAN_POINT('Ctrl Pts',(-0.0864893927053731,-0.281707000625053,
-4.02775857821016));
#27908=CARTESIAN_POINT('Ctrl Pts',(0.00665488172808236,-0.310304059667843,
-4.02246338306866));
#27909=CARTESIAN_POINT('Ctrl Pts',(0.115386929051455,-0.288129751159088,
-4.01716818792715));
#27910=CARTESIAN_POINT('Ctrl Pts',(0.189894713939502,-0.225342510127807,
-4.01187299278565));
#27911=CARTESIAN_POINT('Ctrl Pts',(0.264402498827548,-0.162555269096528,
-4.00657779764415));
#27912=CARTESIAN_POINT('Ctrl Pts',(0.304686021280268,-0.0591550955427229,
-4.00128260250265));
#27913=CARTESIAN_POINT('Ctrl Pts',(0.292290701520345,0.0374885989910175,
-3.99598740736115));
#27914=CARTESIAN_POINT('Ctrl Pts',(0.279895381760423,0.134132293524755,
-3.99069221221964));
#27915=CARTESIAN_POINT('Ctrl Pts',(0.214821219787862,0.224019509038431,
-3.98539701707814));
#27916=CARTESIAN_POINT('Ctrl Pts',(0.126879816978892,0.265971354276274,
-3.98010182193664));
#27917=CARTESIAN_POINT('Ctrl Pts',(0.0389384141699212,0.307923199514117,
-3.97480662679514));
#27918=CARTESIAN_POINT('Ctrl Pts',(-0.0718702294754556,0.301939674476127,
-3.96951143165363));
#27919=CARTESIAN_POINT('Ctrl Pts',(-0.154782753823608,0.250761935663777,
-3.96421623651213));
#27920=CARTESIAN_POINT('Ctrl Pts',(-0.237695278171766,0.199584196851422,
-3.95892104137063));
#27921=CARTESIAN_POINT('Ctrl Pts',(-0.292711683222693,0.103212244264697,
-3.95362584622913));
#27922=CARTESIAN_POINT('Ctrl Pts',(-0.294628000429138,0.00579573964666751,
-3.94833065108763));
#27923=CARTESIAN_POINT('Ctrl Pts',(-0.294665763138638,0.00387606207341759,
-3.94822630462807));
#27924=CARTESIAN_POINT('Ctrl Pts',(-0.294682905939502,0.00195597887809947,
-3.94812195816852));
#27925=CARTESIAN_POINT('Ctrl Pts',(-0.294679608262217,3.58352270703291E-5,
-3.94801761170896));
#27926=CARTESIAN_POINT('Origin',(0.,0.,-4.78));
#27927=CARTESIAN_POINT('',(-0.29402112681354,0.000254531718302781,-3.83358238829104));
#27928=CARTESIAN_POINT('',(-0.29397219999165,0.000242578469533487,-3.84801761170896));
#27929=CARTESIAN_POINT('',(-0.2942,-3.60291088309151E-17,-4.78));
#27930=CARTESIAN_POINT('Ctrl Pts',(-0.29402112681354,0.000254531718302781,
-3.83358238829104));
#27931=CARTESIAN_POINT('Ctrl Pts',(-0.294260484629604,0.0292597759619457,
-3.83514951931656));
#27932=CARTESIAN_POINT('Ctrl Pts',(-0.290316015523389,0.0582013467529887,
-3.83671665034208));
#27933=CARTESIAN_POINT('Ctrl Pts',(-0.281921184254449,0.0857886711899819,
-3.8382837813676));
#27934=CARTESIAN_POINT('Ctrl Pts',(-0.253555802531341,0.179003765490896,
-3.84357897650911));
#27935=CARTESIAN_POINT('Ctrl Pts',(-0.17438048147878,0.256757382147876,
-3.84887417165061));
#27936=CARTESIAN_POINT('Ctrl Pts',(-0.0806667692689985,0.283429234222764,
-3.85416936679211));
#27937=CARTESIAN_POINT('Ctrl Pts',(0.013046942940783,0.310101086297652,
-3.85946456193361));
#27938=CARTESIAN_POINT('Ctrl Pts',(0.121299046307785,0.285691173790448,
-3.86475975707511));
#27939=CARTESIAN_POINT('Ctrl Pts',(0.194497356191566,0.221382104600103,
-3.87005495221662));
#27940=CARTESIAN_POINT('Ctrl Pts',(0.267695666075345,0.15707303540976,-3.87535014735812));
#27941=CARTESIAN_POINT('Ctrl Pts',(0.305840182475905,0.052864809536277,
-3.88064534249962));
#27942=CARTESIAN_POINT('Ctrl Pts',(0.291456251676112,-0.0435029807442393,
-3.88594053764112));
#27943=CARTESIAN_POINT('Ctrl Pts',(0.277072320876318,-0.139870771024758,
-3.89123573278263));
#27944=CARTESIAN_POINT('Ctrl Pts',(0.210159942876168,-0.22839812571231,
-3.89653092792413));
#27945=CARTESIAN_POINT('Ctrl Pts',(0.121372832354126,-0.268529128301459,
-3.90182612306563));
#27946=CARTESIAN_POINT('Ctrl Pts',(0.0325857218320838,-0.308660130890608,
-3.90712131820713));
#27947=CARTESIAN_POINT('Ctrl Pts',(-0.0780761212118509,-0.300394781381353,
-3.91241651334864));
#27948=CARTESIAN_POINT('Ctrl Pts',(-0.159916585829454,-0.247519580175258,
-3.91771170849014));
#27949=CARTESIAN_POINT('Ctrl Pts',(-0.241680258617952,-0.194693992365591,
-3.92300193509044));
#27950=CARTESIAN_POINT('Ctrl Pts',(-0.294676614452523,-0.0973422294352269,
-3.92829216169074));
#27951=CARTESIAN_POINT('Ctrl Pts',(-0.294685000185643,1.71251697507702E-6,
-3.93358238829104));
#27952=CARTESIAN_POINT('Ctrl Pts',(-0.294679608262217,3.58352270703291E-5,
-3.94801761170896));
#27953=CARTESIAN_POINT('Ctrl Pts',(-0.294515561069259,-0.0954841774555884,
-3.94282676302701));
#27954=CARTESIAN_POINT('Ctrl Pts',(-0.24376760897675,-0.191153799453464,
-3.93763591434507));
#27955=CARTESIAN_POINT('Ctrl Pts',(-0.164524860722765,-0.244480713889306,
-3.93244506566312));
#27956=CARTESIAN_POINT('Ctrl Pts',(-0.0836891744479772,-0.298879606157931,
-3.92714987052162));
#27957=CARTESIAN_POINT('Ctrl Pts',(0.0267984274635758,-0.309216334045853,
-3.92185467538011));
#27958=CARTESIAN_POINT('Ctrl Pts',(0.116321659345001,-0.27075546322323,
-3.91655948023861));
#27959=CARTESIAN_POINT('Ctrl Pts',(0.205844891226431,-0.232294592400605,
-3.91126428509711));
#27960=CARTESIAN_POINT('Ctrl Pts',(0.274403753077735,-0.145036122867431,
-3.90596908995561));
#27961=CARTESIAN_POINT('Ctrl Pts',(0.290590242796307,-0.0489546720638047,
-3.9006738948141));
#27962=CARTESIAN_POINT('Ctrl Pts',(0.30677673251488,0.0471267787398241,
-3.8953786996726));
#27963=CARTESIAN_POINT('Ctrl Pts',(0.270590850100718,0.152031210813905,
-3.8900835045311));
#27964=CARTESIAN_POINT('Ctrl Pts',(0.198609974058795,0.217700086238457,
-3.8847883093896));
#27965=CARTESIAN_POINT('Ctrl Pts',(0.126629098016877,0.283368961663006,
-3.8794931142481));
#27966=CARTESIAN_POINT('Ctrl Pts',(0.0188532283472031,0.309802280438032,
-3.87419791910659));
#27967=CARTESIAN_POINT('Ctrl Pts',(-0.0753436385431076,0.284890480118608,
-3.86890272396509));
#27968=CARTESIAN_POINT('Ctrl Pts',(-0.169540505433421,0.259978679799183,
-3.86360752882359));
#27969=CARTESIAN_POINT('Ctrl Pts',(-0.250158369544369,0.183721760385306,
-3.85831233368208));
#27970=CARTESIAN_POINT('Ctrl Pts',(-0.280264795244433,0.0910543401993367,
-3.85301713854058));
#27971=CARTESIAN_POINT('Ctrl Pts',(-0.289739918701928,0.0618899599604794,
-3.85135062959671));
#27972=CARTESIAN_POINT('Ctrl Pts',(-0.294211920145012,0.0311001313031377,
-3.84968412065283));
#27973=CARTESIAN_POINT('Ctrl Pts',(-0.29397219999165,0.000242578469533487,
-3.84801761170896));
#27974=CARTESIAN_POINT('Origin',(0.,0.,-4.78));
#27975=CARTESIAN_POINT('',(-0.29378381590831,-0.000139877028472651,-3.73358238829104));
#27976=CARTESIAN_POINT('',(-0.293811721941862,-0.000165168621852261,-3.74801761170896));
#27977=CARTESIAN_POINT('',(-0.2942,-3.60291088309151E-17,-4.78));
#27978=CARTESIAN_POINT('Ctrl Pts',(-0.29378381590831,-0.000139877028472651,
-3.73358238829104));
#27979=CARTESIAN_POINT('Ctrl Pts',(-0.293533849155245,0.0578968704636794,
-3.73671168180088));
#27980=CARTESIAN_POINT('Ctrl Pts',(-0.27691793885819,0.116065279437388,
-3.73984097531072));
#27981=CARTESIAN_POINT('Ctrl Pts',(-0.244888473326125,0.163916351090838,
-3.74297026882056));
#27982=CARTESIAN_POINT('Ctrl Pts',(-0.190690211086743,0.244886947597132,
-3.74826546396206));
#27983=CARTESIAN_POINT('Ctrl Pts',(-0.0923578601504312,0.296315606927623,
-3.75356065910357));
#27984=CARTESIAN_POINT('Ctrl Pts',(0.00506283766768875,0.294641572816598,
-3.75885585424507));
#27985=CARTESIAN_POINT('Ctrl Pts',(0.102483535485809,0.292967538705573,
-3.76415104938657));
#27986=CARTESIAN_POINT('Ctrl Pts',(0.198992580185736,0.238190811153031,
-3.76944624452807));
#27987=CARTESIAN_POINT('Ctrl Pts',(0.250376464661925,0.155405763325283,
-3.77474143966957));
#27988=CARTESIAN_POINT('Ctrl Pts',(0.301760349138113,0.0726207154975354,
-3.78003663481108));
#27989=CARTESIAN_POINT('Ctrl Pts',(0.308019073390562,-0.0381726526054187,
-3.78533182995258));
#27990=CARTESIAN_POINT('Ctrl Pts',(0.266285946015037,-0.126218084919271,
-3.79062702509408));
#27991=CARTESIAN_POINT('Ctrl Pts',(0.224552818639513,-0.214263517233121,
-3.79592222023558));
#27992=CARTESIAN_POINT('Ctrl Pts',(0.134827839636018,-0.279561013757871,
-3.80121741537709));
#27993=CARTESIAN_POINT('Ctrl Pts',(0.0382152982347072,-0.292196604806581,
-3.80651261051859));
#27994=CARTESIAN_POINT('Ctrl Pts',(-0.0583972431666067,-0.304832195855292,
-3.81180780566009));
#27995=CARTESIAN_POINT('Ctrl Pts',(-0.161897346965737,-0.264805881427962,
-3.81710300080159));
#27996=CARTESIAN_POINT('Ctrl Pts',(-0.224869677668475,-0.190454438241872,
-3.8223981959431));
#27997=CARTESIAN_POINT('Ctrl Pts',(-0.26920513275918,-0.138107557738643,
-3.82612626005908));
#27998=CARTESIAN_POINT('Ctrl Pts',(-0.293451716042893,-0.068746342158254,
-3.82985432417506));
#27999=CARTESIAN_POINT('Ctrl Pts',(-0.29402112681354,0.000254531718302781,
-3.83358238829104));
#28000=CARTESIAN_POINT('Ctrl Pts',(-0.29397219999165,0.000242578469533487,
-3.84801761170896));
#28001=CARTESIAN_POINT('Ctrl Pts',(-0.293450229068545,-0.0669472055825752,
-3.84438892551133));
#28002=CARTESIAN_POINT('Ctrl Pts',(-0.270589287922796,-0.134458079989008,
-3.84076023931371));
#28003=CARTESIAN_POINT('Ctrl Pts',(-0.228397637201052,-0.186208940374743,
-3.83713155311608));
#28004=CARTESIAN_POINT('Ctrl Pts',(-0.166829066168424,-0.261726879804802,
-3.83183635797458));
#28005=CARTESIAN_POINT('Ctrl Pts',(-0.0640969368139846,-0.303684837706857,
-3.82654116283307));
#28006=CARTESIAN_POINT('Ctrl Pts',(0.0327353628682028,-0.292861139192928,
-3.82124596769157));
#28007=CARTESIAN_POINT('Ctrl Pts',(0.12956766255039,-0.282037440678999,
-3.81595077255007));
#28008=CARTESIAN_POINT('Ctrl Pts',(0.220500132560325,-0.218432085749086,
-3.81065557740857));
#28009=CARTESIAN_POINT('Ctrl Pts',(0.263875069310696,-0.131183803754455,
-3.80536038226706));
#28010=CARTESIAN_POINT('Ctrl Pts',(0.307250006061066,-0.0439355217598243,
-3.80006518712556));
#28011=CARTESIAN_POINT('Ctrl Pts',(0.303067409551872,0.0669556872995245,
-3.79476999198406));
#28012=CARTESIAN_POINT('Ctrl Pts',(0.253243328461185,0.150688665578043,
-3.78947479684256));
#28013=CARTESIAN_POINT('Ctrl Pts',(0.203419247370498,0.234421643856562,
-3.78417960170105));
#28014=CARTESIAN_POINT('Ctrl Pts',(0.107953681698318,0.290996391354251,
-3.77888440655955));
#28015=CARTESIAN_POINT('Ctrl Pts',(0.0105811993363878,0.294494983786205,
-3.77358921141805));
#28016=CARTESIAN_POINT('Ctrl Pts',(-0.08679128302554,0.297993576218159,
-3.76829401627655));
#28017=CARTESIAN_POINT('Ctrl Pts',(-0.186070682077219,0.248416013584381,
-3.76299882113504));
#28018=CARTESIAN_POINT('Ctrl Pts',(-0.241775650694887,0.168474736970626,
-3.75770362599354));
#28019=CARTESIAN_POINT('Ctrl Pts',(-0.275740978842037,0.11973165785098,
-3.75447495456535));
#28020=CARTESIAN_POINT('Ctrl Pts',(-0.29350628959498,0.0597000159267478,
-3.75124628313715));
#28021=CARTESIAN_POINT('Ctrl Pts',(-0.293811721941862,-0.000165168621852261,
-3.74801761170896));
#28022=CARTESIAN_POINT('Origin',(0.,0.,-4.78));
#28023=CARTESIAN_POINT('',(-0.294602820716591,-0.000172945526623114,-3.63358238829104));
#28024=CARTESIAN_POINT('',(-0.294584692827634,-0.000157098441292656,-3.64801761170896));
#28025=CARTESIAN_POINT('',(-0.2942,-3.60291088309151E-17,-4.78));
#28026=CARTESIAN_POINT('Ctrl Pts',(-0.294602820716591,-0.000172945526623114,
-3.63358238829104));
#28027=CARTESIAN_POINT('Ctrl Pts',(-0.293985296127081,0.0862757997737715,
-3.6382738442852));
#28028=CARTESIAN_POINT('Ctrl Pts',(-0.253543207095474,0.173218312496561,
-3.64296530027936));
#28029=CARTESIAN_POINT('Ctrl Pts',(-0.186746316274069,0.227928150582927,
-3.64765675627352));
#28030=CARTESIAN_POINT('Ctrl Pts',(-0.111353395145683,0.289678547301548,
-3.65295195141502));
#28031=CARTESIAN_POINT('Ctrl Pts',(-0.00238606325056179,0.310366481589784,
-3.65824714655652));
#28032=CARTESIAN_POINT('Ctrl Pts',(0.0903415413845116,0.280493415878642,
-3.66354234169803));
#28033=CARTESIAN_POINT('Ctrl Pts',(0.183069146019585,0.2506203501675,-3.66883753683953));
#28034=CARTESIAN_POINT('Ctrl Pts',(0.259557023394611,0.17018628445698,-3.67413273198103));
#28035=CARTESIAN_POINT('Ctrl Pts',(0.284710385565443,0.0760501837047467,
-3.67942792712253));
#28036=CARTESIAN_POINT('Ctrl Pts',(0.309863747736276,-0.0180859170474864,
-3.68472312226404));
#28037=CARTESIAN_POINT('Ctrl Pts',(0.283682594702916,-0.125924052841432,
-3.69001831740554));
#28038=CARTESIAN_POINT('Ctrl Pts',(0.218189061309932,-0.198067237438836,
-3.69531351254704));
#28039=CARTESIAN_POINT('Ctrl Pts',(0.152695527916949,-0.27021042203624,
-3.70060870768854));
#28040=CARTESIAN_POINT('Ctrl Pts',(0.0478896141643412,-0.306658655437101,
-3.70590390283004));
#28041=CARTESIAN_POINT('Ctrl Pts',(-0.0482298065556536,-0.290711509461145,
-3.71119909797155));
#28042=CARTESIAN_POINT('Ctrl Pts',(-0.144349227275646,-0.274764363485189,
-3.71649429311305));
#28043=CARTESIAN_POINT('Ctrl Pts',(-0.231782154963025,-0.206421838132418,
-3.72178948825455));
#28044=CARTESIAN_POINT('Ctrl Pts',(-0.270466532035491,-0.116994308614986,
-3.72708468339606));
#28045=CARTESIAN_POINT('Ctrl Pts',(-0.286289660963147,-0.0804156317350293,
-3.72925058502772));
#28046=CARTESIAN_POINT('Ctrl Pts',(-0.29395682729143,-0.040309290889572,
-3.73141648665938));
#28047=CARTESIAN_POINT('Ctrl Pts',(-0.29378381590831,-0.000139877028472651,
-3.73358238829104));
#28048=CARTESIAN_POINT('Ctrl Pts',(-0.293811721941862,-0.000165168621852261,
-3.74801761170896));
#28049=CARTESIAN_POINT('Ctrl Pts',(-0.294007215104199,-0.0384821129819785,
-3.74595108799565));
#28050=CARTESIAN_POINT('Ctrl Pts',(-0.287049937609616,-0.0767308649180593,
-3.74388456428235));
#28051=CARTESIAN_POINT('Ctrl Pts',(-0.272609541015007,-0.111907800977432,
-3.74181804056904));
#28052=CARTESIAN_POINT('Ctrl Pts',(-0.235607924533802,-0.202044071717994,
-3.73652284542754));
#28053=CARTESIAN_POINT('Ctrl Pts',(-0.149474153387738,-0.27201162260538,
-3.73122765028603));
#28054=CARTESIAN_POINT('Ctrl Pts',(-0.0536685951641096,-0.289756730929934,
-3.72593245514453));
#28055=CARTESIAN_POINT('Ctrl Pts',(0.0421369630595187,-0.307501839254488,
-3.72063726000303));
#28056=CARTESIAN_POINT('Ctrl Pts',(0.147614308360711,-0.27302450501621,
-3.71534206486152));
#28057=CARTESIAN_POINT('Ctrl Pts',(0.214444362295811,-0.20212011735872,
-3.71004686972002));
#28058=CARTESIAN_POINT('Ctrl Pts',(0.28127441623091,-0.131215729701233,
-3.70475167457852));
#28059=CARTESIAN_POINT('Ctrl Pts',(0.309457178799918,-0.023884288624536,
-3.69945647943702));
#28060=CARTESIAN_POINT('Ctrl Pts',(0.286077924579446,0.0707052133088147,
-3.69416128429552));
#28061=CARTESIAN_POINT('Ctrl Pts',(0.262698670358975,0.165294715242165,
-3.68886608915401));
#28062=CARTESIAN_POINT('Ctrl Pts',(0.187757399349022,0.24714227803217,-3.68357089401251));
#28063=CARTESIAN_POINT('Ctrl Pts',(0.0955931833176489,0.278749407497395,
-3.67827569887101));
#28064=CARTESIAN_POINT('Ctrl Pts',(0.00342896728627082,0.310356536962622,
-3.6729805037295));
#28065=CARTESIAN_POINT('Ctrl Pts',(-0.105958193766529,0.291723233103062,
-3.667685308588));
#28066=CARTESIAN_POINT('Ctrl Pts',(-0.182470015924895,0.231390967676254,
-3.6623901134465));
#28067=CARTESIAN_POINT('Ctrl Pts',(-0.251694175282413,0.17680528093544,
-3.65759927953399));
#28068=CARTESIAN_POINT('Ctrl Pts',(-0.294007415616088,0.0880858813310743,
-3.65280844562147));
#28069=CARTESIAN_POINT('Ctrl Pts',(-0.294584692827634,-0.000157098441292656,
-3.64801761170896));
#28070=CARTESIAN_POINT('Origin',(0.,0.,-6.1506589891905));
#28071=CARTESIAN_POINT('',(-0.237499741684084,-0.000139423369390631,-3.6006589891905));
#28072=CARTESIAN_POINT('',(-0.237175,1.98931295048561E-15,-3.6));
#28073=CARTESIAN_POINT('',(-0.237175,1.98931295048561E-15,-6.1506589891905));
#28074=CARTESIAN_POINT('',(-0.236971720686989,-0.00981754651873418,-3.6));
#28075=CARTESIAN_POINT('Ctrl Pts',(-0.237499741684084,-0.000139423369390674,
-3.6006589891905));
#28076=CARTESIAN_POINT('Ctrl Pts',(-0.237523051019196,-0.00340255298153232,
-3.600439326127));
#28077=CARTESIAN_POINT('Ctrl Pts',(-0.237475976012487,-0.00666480992888717,
-3.6002196630635));
#28078=CARTESIAN_POINT('Ctrl Pts',(-0.237357402024655,-0.00992348605843001,
-3.6));
#28079=CARTESIAN_POINT('Origin',(0.,0.,-3.6));
#28080=CARTESIAN_POINT('Origin',(0.,0.,-6.1506589891905));
#28081=CARTESIAN_POINT('',(-0.236839485173533,-0.000112764562290553,-3.7006589891905));
#28082=CARTESIAN_POINT('',(-0.237485127537029,-0.000126647936150415,-3.6809410108095));
#28083=CARTESIAN_POINT('',(-0.237175,1.98931295048561E-15,-6.1506589891905));
#28084=CARTESIAN_POINT('Ctrl Pts',(-0.236839485173533,-0.000112764562290573,
-3.7006589891905));
#28085=CARTESIAN_POINT('Ctrl Pts',(-0.236978961634416,-0.0324961117156111,
-3.69849308755884));
#28086=CARTESIAN_POINT('Ctrl Pts',(-0.215686539381533,-0.143875088998195,
-3.69103199078568));
#28087=CARTESIAN_POINT('Ctrl Pts',(-0.0458841718383633,-0.276602230999808,
-3.67827569887101));
#28088=CARTESIAN_POINT('Ctrl Pts',(0.207589749925143,-0.188451893574426,
-3.6623901134465));
#28089=CARTESIAN_POINT('Ctrl Pts',(0.27090907321563,0.0723554809013986,
-3.64650452802199));
#28090=CARTESIAN_POINT('Ctrl Pts',(0.0859225438163616,0.266885897640616,
-3.63061894259749));
#28091=CARTESIAN_POINT('Ctrl Pts',(-0.167599901511316,0.218753529908791,
-3.61533709632032));
#28092=CARTESIAN_POINT('Ctrl Pts',(-0.237001912334942,0.0695528987469263,
-3.60535044518466));
#28093=CARTESIAN_POINT('Ctrl Pts',(-0.237499741684084,-0.000139423369390674,
-3.6006589891905));
#28094=CARTESIAN_POINT('',(-0.0864920085589077,0.220841828194855,-3.6));
#28095=CARTESIAN_POINT('Origin',(0.,0.,-3.6));
#28096=CARTESIAN_POINT('Ctrl Pts',(-0.237485127537029,-0.000126647936150416,
-3.6809410108095));
#28097=CARTESIAN_POINT('Ctrl Pts',(-0.237534121349303,-0.00761587477375465,
-3.68043664958051));
#28098=CARTESIAN_POINT('Ctrl Pts',(-0.233809530212368,-0.093684159787474,
-3.67463709321002));
#28099=CARTESIAN_POINT('Ctrl Pts',(-0.12883195646667,-0.249024285245638,
-3.66354234169802));
#28100=CARTESIAN_POINT('Ctrl Pts',(0.139350939164339,-0.243214763219636,
-3.64765675627352));
#28101=CARTESIAN_POINT('Ctrl Pts',(0.280177793680504,-0.0146860234836151,
-3.63177117084901));
#28102=CARTESIAN_POINT('Ctrl Pts',(0.163650290907218,0.227552512000709,
-3.61588558542451));
#28103=CARTESIAN_POINT('Ctrl Pts',(-0.0130164034045845,0.24961831823673,
-3.6052951951415));
#28104=CARTESIAN_POINT('Ctrl Pts',(-0.0864920085589077,0.220841828194855,
-3.6));
#28105=CARTESIAN_POINT('Origin',(0.,0.,-6.1506589891905));
#28106=CARTESIAN_POINT('',(-0.237030797933384,0.000205195650219347,-3.8006589891905));
#28107=CARTESIAN_POINT('',(-0.236861982160303,-0.000133153867742014,-3.7809410108095));
#28108=CARTESIAN_POINT('',(-0.237175,1.98931295048561E-15,-6.1506589891905));
#28109=CARTESIAN_POINT('Ctrl Pts',(-0.237030797933384,0.000205195650219349,
-3.8006589891905));
#28110=CARTESIAN_POINT('Ctrl Pts',(-0.236571756466603,-0.0554211886518688,
-3.79693092507452));
#28111=CARTESIAN_POINT('Ctrl Pts',(-0.189261331157349,-0.190760199954121,
-3.78790766581703));
#28112=CARTESIAN_POINT('Ctrl Pts',(0.0363605403484637,-0.278014334385727,
-3.77358921141805));
#28113=CARTESIAN_POINT('Ctrl Pts',(0.253361103521349,-0.12009182855713,
-3.75770362599354));
#28114=CARTESIAN_POINT('Ctrl Pts',(0.238224329987279,0.147862798361475,
-3.74181804056903));
#28115=CARTESIAN_POINT('Ctrl Pts',(0.00481645089103148,0.280340742181402,
-3.72593245514453));
#28116=CARTESIAN_POINT('Ctrl Pts',(-0.200576150596734,0.17291865748255,
-3.71221277135168));
#28117=CARTESIAN_POINT('Ctrl Pts',(-0.236637969658038,0.0466746779477384,
-3.70378828270034));
#28118=CARTESIAN_POINT('Ctrl Pts',(-0.236839485173533,-0.000112764562290573,
-3.7006589891905));
#28119=CARTESIAN_POINT('Ctrl Pts',(-0.236861982160303,-0.000133153867742007,
-3.7809410108095));
#28120=CARTESIAN_POINT('Ctrl Pts',(-0.237019582740782,-0.0310230970309381,
-3.77887448709619));
#28121=CARTESIAN_POINT('Ctrl Pts',(-0.217039172494002,-0.140868615727758,
-3.77151276824138));
#28122=CARTESIAN_POINT('Ctrl Pts',(-0.0510630698782088,-0.275693101540268,
-3.75885585424507));
#28123=CARTESIAN_POINT('Ctrl Pts',(0.204034714334676,-0.192309399147709,
-3.74297026882056));
#28124=CARTESIAN_POINT('Ctrl Pts',(0.272194945935335,0.0672725301932114,
-3.72708468339606));
#28125=CARTESIAN_POINT('Ctrl Pts',(0.0909488961210605,0.265221500669614,
-3.71119909797155));
#28126=CARTESIAN_POINT('Ctrl Pts',(-0.165205329670506,0.221587499401578,
-3.69581787377603));
#28127=CARTESIAN_POINT('Ctrl Pts',(-0.237019744387309,0.0710121308793213,
-3.68573184472201));
#28128=CARTESIAN_POINT('Ctrl Pts',(-0.237485127537029,-0.000126647936150416,
-3.6809410108095));
#28129=CARTESIAN_POINT('Origin',(0.,0.,-6.1506589891905));
#28130=CARTESIAN_POINT('',(-0.237565997280583,1.38059634504043E-6,-3.9006589891905));
#28131=CARTESIAN_POINT('',(-0.236991354632969,0.000195559308326751,-3.8809410108095));
#28132=CARTESIAN_POINT('',(-0.237175,1.98931295048561E-15,-6.1506589891905));
#28133=CARTESIAN_POINT('Ctrl Pts',(-0.237565992246873,1.38057857121606E-6,
-3.9006589891905));
#28134=CARTESIAN_POINT('Ctrl Pts',(-0.237559231926505,-0.0784743142974118,
-3.8953687625902));
#28135=CARTESIAN_POINT('Ctrl Pts',(-0.152071038566501,-0.235512023820444,
-3.8847833408484));
#28136=CARTESIAN_POINT('Ctrl Pts',(0.115481785178347,-0.255495584003526,
-3.86890272396509));
#28137=CARTESIAN_POINT('Ctrl Pts',(0.277309894480033,-0.0413914846015558,
-3.85301713854059));
#28138=CARTESIAN_POINT('Ctrl Pts',(0.185057083358657,0.210636924353684,
-3.83713155311608));
#28139=CARTESIAN_POINT('Ctrl Pts',(-0.0767514749289204,0.269672488584438,
-3.82124596769156));
#28140=CARTESIAN_POINT('Ctrl Pts',(-0.223299221161425,0.125756213525167,
-3.80908844638305));
#28141=CARTESIAN_POINT('Ctrl Pts',(-0.23722376084985,0.023588332303802,
-3.80222612021602));
#28142=CARTESIAN_POINT('Ctrl Pts',(-0.237030797933384,0.000205195650219349,
-3.8006589891905));
#28143=CARTESIAN_POINT('Ctrl Pts',(-0.236991354632969,0.000195559308326754,
-3.8809410108095));
#28144=CARTESIAN_POINT('Ctrl Pts',(-0.236570557713568,-0.0539707800273571,
-3.87731232461187));
#28145=CARTESIAN_POINT('Ctrl Pts',(-0.191246924065396,-0.187816456780419,
-3.86838844327274));
#28146=CARTESIAN_POINT('Ctrl Pts',(0.0311465050672407,-0.278646601116737,
-3.85416936679211));
#28147=CARTESIAN_POINT('Ctrl Pts',(0.251067394679135,-0.124816552964098,
-3.83828378136761));
#28148=CARTESIAN_POINT('Ctrl Pts',(0.240951752322899,0.143374703072453,
-3.82239819594309));
#28149=CARTESIAN_POINT('Ctrl Pts',(0.0100675354129855,0.280201172186297,
-3.80651261051859));
#28150=CARTESIAN_POINT('Ctrl Pts',(-0.198805302366879,0.175895482421437,
-3.79269354880739));
#28151=CARTESIAN_POINT('Ctrl Pts',(-0.236615751987389,0.0481283184140897,
-3.78416968223769));
#28152=CARTESIAN_POINT('Ctrl Pts',(-0.236861982160303,-0.000133153867742007,
-3.7809410108095));
#28153=CARTESIAN_POINT('Origin',(0.,0.,-6.1506589891905));
#28154=CARTESIAN_POINT('',(-0.237034860401358,-0.000206013329817485,-4.0006589891905));
#28155=CARTESIAN_POINT('',(-0.237561645443886,2.88892589412493E-5,-3.9809410108095));
#28156=CARTESIAN_POINT('',(-0.237175,1.98931295048561E-15,-6.1506589891905));
#28157=CARTESIAN_POINT('Ctrl Pts',(-0.237034860401358,-0.000206013329817466,
-4.0006589891905));
#28158=CARTESIAN_POINT('Ctrl Pts',(-0.237227612547211,-0.0234398712075855,
-3.99910179524738));
#28159=CARTESIAN_POINT('Ctrl Pts',(-0.22341484328665,-0.125455592362394,
-3.99224940616276));
#28160=CARTESIAN_POINT('Ctrl Pts',(-0.0772564444343335,-0.269528249207591,
-3.98010182193664));
#28161=CARTESIAN_POINT('Ctrl Pts',(0.184662206520241,-0.210983186133545,
-3.96421623651213));
#28162=CARTESIAN_POINT('Ctrl Pts',(0.277386942916036,0.0408719852250892,
-3.94833065108763));
#28163=CARTESIAN_POINT('Ctrl Pts',(0.115960147730902,0.25527882694822,-3.93244506566312));
#28164=CARTESIAN_POINT('Ctrl Pts',(-0.151713354856548,0.235790359050968,
-3.91655948023861));
#28165=CARTESIAN_POINT('Ctrl Pts',(-0.237532576511483,0.0786981808764117,
-3.9059641214144));
#28166=CARTESIAN_POINT('Ctrl Pts',(-0.237565998596115,7.50843634444512E-5,
-3.9006639577317));
#28167=CARTESIAN_POINT('Ctrl Pts',(-0.237565992246873,1.38057857121606E-6,
-3.9006589891905));
#28168=CARTESIAN_POINT('Ctrl Pts',(-0.237561645443886,2.88892589412437E-5,
-3.9809410108095));
#28169=CARTESIAN_POINT('Ctrl Pts',(-0.237429395637666,-0.0769764098845311,
-3.97575016212755));
#28170=CARTESIAN_POINT('Ctrl Pts',(-0.154784114476735,-0.232778614358938,
-3.9652641183041));
#28171=CARTESIAN_POINT('Ctrl Pts',(0.110675778439994,-0.257613859497429,
-3.94948287933915));
#28172=CARTESIAN_POINT('Ctrl Pts',(0.276485921807596,-0.0465785687612247,
-3.93359729391465));
#28173=CARTESIAN_POINT('Ctrl Pts',(0.188970082294562,0.207133620332956,
-3.91771170849014));
#28174=CARTESIAN_POINT('Ctrl Pts',(-0.0716867010729343,0.271062808441053,
-3.90182612306563));
#28175=CARTESIAN_POINT('Ctrl Pts',(-0.222124224235629,0.128763056306054,
-3.88956922383875));
#28176=CARTESIAN_POINT('Ctrl Pts',(-0.237184609654634,0.025071970230525,
-3.88260751975337));
#28177=CARTESIAN_POINT('Ctrl Pts',(-0.236991354632969,0.000195559308326754,
-3.8809410108095));
#28178=CARTESIAN_POINT('Origin',(0.,0.,-6.1506589891905));
#28179=CARTESIAN_POINT('',(-0.236836491818845,0.000110831649961404,-4.1006589891905));
#28180=CARTESIAN_POINT('',(-0.237076567927639,-0.000212689822428169,-4.0809410108095));
#28181=CARTESIAN_POINT('',(-0.237175,1.98931295048561E-15,-6.1506589891905));
#28182=CARTESIAN_POINT('Ctrl Pts',(-0.236836491818845,0.000110831649961389,
-4.1006589891905));
#28183=CARTESIAN_POINT('Ctrl Pts',(-0.236639836850206,-0.0465291493340525,
-4.09753963276306));
#28184=CARTESIAN_POINT('Ctrl Pts',(-0.200752511647945,-0.172621020014775,
-4.08912508119413));
#28185=CARTESIAN_POINT('Ctrl Pts',(0.00429227712398719,-0.280349088964778,
-4.07541533448367));
#28186=CARTESIAN_POINT('Ctrl Pts',(0.237946464991633,-0.148308850460187,
-4.05952974905918));
#28187=CARTESIAN_POINT('Ctrl Pts',(0.253585853911662,0.11961709752968,-4.04364416363466));
#28188=CARTESIAN_POINT('Ctrl Pts',(0.0368810936713182,0.2779457145844,-4.02775857821017));
#28189=CARTESIAN_POINT('Ctrl Pts',(-0.189060335164718,0.191054117653322,
-4.01343018672877));
#28190=CARTESIAN_POINT('Ctrl Pts',(-0.23657216418078,0.0555662229892069,
-4.00439699038888));
#28191=CARTESIAN_POINT('Ctrl Pts',(-0.237034860401358,-0.000206013329817466,
-4.0006589891905));
#28192=CARTESIAN_POINT('Ctrl Pts',(-0.237076567927639,-0.000212689822428173,
-4.0809410108095));
#28193=CARTESIAN_POINT('Ctrl Pts',(-0.237265375825923,-0.0219540932160755,
-4.07948319478473));
#28194=CARTESIAN_POINT('Ctrl Pts',(-0.224552153366904,-0.122449579388927,
-4.07273018361847));
#28195=CARTESIAN_POINT('Ctrl Pts',(-0.0822914743374018,-0.268033844229383,
-4.0606819773107));
#28196=CARTESIAN_POINT('Ctrl Pts',(0.180677832160775,-0.214405105746405,
-4.04479639188619));
#28197=CARTESIAN_POINT('Ctrl Pts',(0.278103846141642,0.0356690223564828,
-4.02891080646169));
#28198=CARTESIAN_POINT('Ctrl Pts',(0.1207214766735,0.253061955797574,-4.01302522103717));
#28199=CARTESIAN_POINT('Ctrl Pts',(-0.14727009426389,0.238590753715125,
-3.99713963561268));
#28200=CARTESIAN_POINT('Ctrl Pts',(-0.236849170311852,0.081675548847311,
-3.98644489887011));
#28201=CARTESIAN_POINT('Ctrl Pts',(-0.237564303929984,0.00157685006938821,
-3.98104535726905));
#28202=CARTESIAN_POINT('Ctrl Pts',(-0.237561645443886,2.88892589412437E-5,
-3.9809410108095));
#28203=CARTESIAN_POINT('Origin',(0.,0.,-6.1506589891905));
#28204=CARTESIAN_POINT('',(-0.237440599831179,0.000151834494169013,-4.2006589891905));
#28205=CARTESIAN_POINT('',(-0.236817680733397,8.90465815239633E-5,-4.1809410108095));
#28206=CARTESIAN_POINT('',(-0.237175,1.98931295048561E-15,-6.1506589891905));
#28207=CARTESIAN_POINT('Ctrl Pts',(-0.237440599831179,0.000151834494169018,
-4.2006589891905));
#28208=CARTESIAN_POINT('Ctrl Pts',(-0.236922564689605,-0.0693914648962057,
-4.19597747027874));
#28209=CARTESIAN_POINT('Ctrl Pts',(-0.167933984931827,-0.218488341387412,
-4.18600075622548));
#28210=CARTESIAN_POINT('Ctrl Pts',(0.0854715091573248,-0.267036807292018,
-4.17072884703072));
#28211=CARTESIAN_POINT('Ctrl Pts',(0.270747721571937,-0.0728677335311189,
-4.15484326160622));
#28212=CARTESIAN_POINT('Ctrl Pts',(0.207955486803503,0.188065283438102,
-4.1389576761817));
#28213=CARTESIAN_POINT('Ctrl Pts',(-0.0453727731435854,0.276686368987695,
-4.12307209075721));
#28214=CARTESIAN_POINT('Ctrl Pts',(-0.215547649412793,0.144175982261373,
-4.11030586176013));
#28215=CARTESIAN_POINT('Ctrl Pts',(-0.23697366418245,0.0326435282522547,
-4.10283482790456));
#28216=CARTESIAN_POINT('Ctrl Pts',(-0.236836491818845,0.000110831649961389,
-4.1006589891905));
#28217=CARTESIAN_POINT('Ctrl Pts',(-0.236817680733397,8.90465815239772E-5,
-4.1809410108095));
#28218=CARTESIAN_POINT('Ctrl Pts',(-0.236665414212453,-0.0450740145522511,
-4.17792103230042));
#28219=CARTESIAN_POINT('Ctrl Pts',(-0.202479259262566,-0.169638983975812,
-4.16960585864983));
#28220=CARTESIAN_POINT('Ctrl Pts',(-0.000959750965527487,-0.280380290461363,
-4.15599548985773));
#28221=CARTESIAN_POINT('Ctrl Pts',(0.235126705419149,-0.152739846798193,
-4.14010990443324));
#28222=CARTESIAN_POINT('Ctrl Pts',(0.255781924318054,0.114846138782203,
-4.12422431900872));
#28223=CARTESIAN_POINT('Ctrl Pts',(0.0420808782244523,0.277206111204153,
-4.10833873358422));
#28224=CARTESIAN_POINT('Ctrl Pts',(-0.187026567625837,0.193988718634259,
-4.09391096418447));
#28225=CARTESIAN_POINT('Ctrl Pts',(-0.236579572783091,0.0570167588419758,
-4.08477838992624));
#28226=CARTESIAN_POINT('Ctrl Pts',(-0.237076567927639,-0.000212689822428173,
-4.0809410108095));
#28227=CARTESIAN_POINT('Origin',(0.,0.,-6.1506589891905));
#28228=CARTESIAN_POINT('',(-0.237304285819382,-0.000201120099325924,-4.3006589891905));
#28229=CARTESIAN_POINT('',(-0.237403111349647,0.000169659163617816,-4.2809410108095));
#28230=CARTESIAN_POINT('',(-0.237175,1.98931295048561E-15,-6.1506589891905));
#28231=CARTESIAN_POINT('Ctrl Pts',(-0.237304285819382,-0.000201120099325937,
-4.3006589891905));
#28232=CARTESIAN_POINT('Ctrl Pts',(-0.237431694732867,-0.0143118172002052,
-4.29971050293593));
#28233=CARTESIAN_POINT('Ctrl Pts',(-0.229859658596377,-0.107062981526376,
-4.29346682153985));
#28234=CARTESIAN_POINT('Ctrl Pts',(-0.107605972147853,-0.258911162533527,
-4.28192794500227));
#28235=CARTESIAN_POINT('Ctrl Pts',(0.159293148852347,-0.230737357302738,
-4.26604235957777));
#28236=CARTESIAN_POINT('Ctrl Pts',(0.2802423654424,0.00884601252520937,
-4.25015677415325));
#28237=CARTESIAN_POINT('Ctrl Pts',(0.144423813031258,0.240324359056379,
-4.23427118872875));
#28238=CARTESIAN_POINT('Ctrl Pts',(-0.123720842908662,0.251609197678298,
-4.21838560330425));
#28239=CARTESIAN_POINT('Ctrl Pts',(-0.232891988211843,0.096973930455177,
-4.20718153679149));
#28240=CARTESIAN_POINT('Ctrl Pts',(-0.23750850639282,0.0092679078409494,
-4.20127266542025));
#28241=CARTESIAN_POINT('Ctrl Pts',(-0.237440599831179,0.000151834494169018,
-4.2006589891905));
#28242=CARTESIAN_POINT('Ctrl Pts',(-0.237403111349647,0.000169659163617811,
-4.28094101080949));
#28243=CARTESIAN_POINT('Ctrl Pts',(-0.236852466100401,-0.0679255050907547,
-4.27635886981609));
#28244=CARTESIAN_POINT('Ctrl Pts',(-0.170354300778626,-0.21565114223581,
-4.26648153368119));
#28245=CARTESIAN_POINT('Ctrl Pts',(0.0804545900663122,-0.268590929367298,
-4.25130900240478));
#28246=CARTESIAN_POINT('Ctrl Pts',(0.269335308407912,-0.0779263758039853,
-4.23542341698027));
#28247=CARTESIAN_POINT('Ctrl Pts',(0.211441681464576,0.184137024361096,
-4.21953783155577));
#28248=CARTESIAN_POINT('Ctrl Pts',(-0.0401821430447466,0.277487700234545,
-4.20365224613126));
#28249=CARTESIAN_POINT('Ctrl Pts',(-0.214153039044315,0.14718162281968,
-4.19078663921584));
#28250=CARTESIAN_POINT('Ctrl Pts',(-0.236932396556695,0.0341143707861283,
-4.18321622744192));
#28251=CARTESIAN_POINT('Ctrl Pts',(-0.236817680733397,8.90465815239772E-5,
-4.1809410108095));
#28252=CARTESIAN_POINT('Origin',(0.,0.,-6.1506589891905));
#28253=CARTESIAN_POINT('',(-0.236790373551236,-3.35771274733464E-5,-4.4006589891905));
#28254=CARTESIAN_POINT('',(-0.23734735502029,-0.000189769014714958,-4.38094101080949));
#28255=CARTESIAN_POINT('',(-0.237175,1.98931295048561E-15,-6.1506589891905));
#28256=CARTESIAN_POINT('Ctrl Pts',(-0.236790373551236,-3.35771274733478E-5,
-4.4006589891905));
#28257=CARTESIAN_POINT('Ctrl Pts',(-0.236837795918825,-0.0375905476484022,
-4.39814834045161));
#28258=CARTESIAN_POINT('Ctrl Pts',(-0.210698941147542,-0.154296333752042,
-4.39034249657121));
#28259=CARTESIAN_POINT('Ctrl Pts',(-0.0278323017717629,-0.27899712956307,
-4.37724145754931));
#28260=CARTESIAN_POINT('Ctrl Pts',(0.219402452553475,-0.174575482642516,
-4.36135587212481));
#28261=CARTESIAN_POINT('Ctrl Pts',(0.265613074904189,0.0897982726241923,
-4.3454702867003));
#28262=CARTESIAN_POINT('Ctrl Pts',(0.0684597913264363,0.271895737917843,
-4.32958470127579));
#28263=CARTESIAN_POINT('Ctrl Pts',(-0.1759020676831,0.20887465967552,-4.31464760210586));
#28264=CARTESIAN_POINT('Ctrl Pts',(-0.23672039812059,0.0644651754777562,
-4.30500569807743));
#28265=CARTESIAN_POINT('Ctrl Pts',(-0.237304285819382,-0.000201120099325937,
-4.3006589891905));
#28266=CARTESIAN_POINT('Ctrl Pts',(-0.23734735502029,-0.000189769014714986,
-4.38094101080949));
#28267=CARTESIAN_POINT('Ctrl Pts',(-0.237457523554163,-0.0128160771384688,
-4.38009190247327));
#28268=CARTESIAN_POINT('Ctrl Pts',(-0.230796517221853,-0.104065922452244,
-4.37394759899555));
#28269=CARTESIAN_POINT('Ctrl Pts',(-0.112436805309618,-0.256850137654031,
-4.36250810037634));
#28270=CARTESIAN_POINT('Ctrl Pts',(0.154943207178462,-0.23368061740414,
-4.34662251495182));
#28271=CARTESIAN_POINT('Ctrl Pts',(0.280358882596026,0.00359518436732559,
-4.33073692952732));
#28272=CARTESIAN_POINT('Ctrl Pts',(0.14890003195752,0.237576953604884,-4.3148513441028));
#28273=CARTESIAN_POINT('Ctrl Pts',(-0.11898618914506,0.253882483038636,
-4.29896575867831));
#28274=CARTESIAN_POINT('Ctrl Pts',(-0.232028528892651,0.0999660525608262,
-4.2876623142472));
#28275=CARTESIAN_POINT('Ctrl Pts',(-0.237488800524134,0.0107663517156311,
-4.28165406495759));
#28276=CARTESIAN_POINT('Ctrl Pts',(-0.237403111349647,0.000169659163617811,
-4.28094101080949));
#28277=CARTESIAN_POINT('Origin',(0.,0.,-6.1506589891905));
#28278=CARTESIAN_POINT('',(-0.237180885702784,0.000217072097893513,-4.5006589891905));
#28279=CARTESIAN_POINT('',(-0.236798869759374,-5.74984565626796E-5,-4.4809410108095));
#28280=CARTESIAN_POINT('',(-0.237175,1.98931295048561E-15,-6.1506589891905));
#28281=CARTESIAN_POINT('Ctrl Pts',(-0.237180885702784,0.000217072097893506,
-4.5006589891905));
#28282=CARTESIAN_POINT('Ctrl Pts',(-0.236621983925057,-0.0604554976673563,
-4.49658617796729));
#28283=CARTESIAN_POINT('Ctrl Pts',(-0.182031586694785,-0.200904114215803,
-4.48721817160257));
#28284=CARTESIAN_POINT('Ctrl Pts',(0.0543372398400151,-0.275066355072582,
-4.47255497009635));
#28285=CARTESIAN_POINT('Ctrl Pts',(0.260625067348198,-0.103385732072151,
-4.45666938467185));
#28286=CARTESIAN_POINT('Ctrl Pts',(0.228119174345422,0.163020482217144,
-4.44078379924733));
#28287=CARTESIAN_POINT('Ctrl Pts',(-0.0133974132773538,0.280061680070342,
-4.42489821382283));
#28288=CARTESIAN_POINT('Ctrl Pts',(-0.206408202951183,0.16255768074852,
-4.41152327713722));
#28289=CARTESIAN_POINT('Ctrl Pts',(-0.23673777766993,0.0416206477494621,
-4.40344353559311));
#28290=CARTESIAN_POINT('Ctrl Pts',(-0.236790373551236,-3.35771274733478E-5,
-4.4006589891905));
#28291=CARTESIAN_POINT('Ctrl Pts',(-0.236798869759374,-5.74984565626727E-5,
-4.4809410108095));
#28292=CARTESIAN_POINT('Ctrl Pts',(-0.236877019742237,-0.0361246334101674,
-4.47852973998896));
#28293=CARTESIAN_POINT('Ctrl Pts',(-0.212182948306362,-0.151294347002612,
-4.47082327402691));
#28294=CARTESIAN_POINT('Ctrl Pts',(-0.0330533685498055,-0.278426836401662,
-4.45782161292337));
#28295=CARTESIAN_POINT('Ctrl Pts',(0.216093941700501,-0.178654517887089,
-4.44193602749886));
#28296=CARTESIAN_POINT('Ctrl Pts',(0.26724849229964,0.0848072624525569,
-4.42605044207435));
#28297=CARTESIAN_POINT('Ctrl Pts',(0.0735407108656338,0.270565689337182,
-4.41016485664985));
#28298=CARTESIAN_POINT('Ctrl Pts',(-0.173592056620874,0.211744102334454,
-4.39512837956156));
#28299=CARTESIAN_POINT('Ctrl Pts',(-0.236770492394035,0.0659238934636766,
-4.38538709761478));
#28300=CARTESIAN_POINT('Ctrl Pts',(-0.23734735502029,-0.000189769014714986,
-4.38094101080949));
#28301=CARTESIAN_POINT('Origin',(0.,0.,-6.1506589891905));
#28302=CARTESIAN_POINT('',(-0.237523476840667,-9.09874636312175E-5,-4.6006589891905));
#28303=CARTESIAN_POINT('',(-0.237136177256987,0.000217231692762283,-4.5809410108095));
#28304=CARTESIAN_POINT('',(-0.237175,1.98931295048561E-15,-6.1506589891905));
#28305=CARTESIAN_POINT('Ctrl Pts',(-0.237523476840667,-9.09874636312079E-5,
-4.6006589891905));
#28306=CARTESIAN_POINT('Ctrl Pts',(-0.237548180986008,-0.00513370532888432,
-4.60031921062447));
#28307=CARTESIAN_POINT('Ctrl Pts',(-0.235115874964421,-0.0887391407442366,
-4.59468423691694));
#28308=CARTESIAN_POINT('Ctrl Pts',(-0.13654042413847,-0.244889256404674,
-4.5837540680679));
#28309=CARTESIAN_POINT('Ctrl Pts',(0.131829301628996,-0.247457209550174,
-4.56786848264339));
#28310=CARTESIAN_POINT('Ctrl Pts',(0.279412451766375,-0.0232962899245847,
-4.55198289721889));
#28311=CARTESIAN_POINT('Ctrl Pts',(0.170988228579068,0.222209498027739,
-4.53609731179438));
#28312=CARTESIAN_POINT('Ctrl Pts',(-0.0941013364397791,0.264119241643986,
-4.52021172636988));
#28313=CARTESIAN_POINT('Ctrl Pts',(-0.227112405750096,0.115332508093694,
-4.50839895216858));
#28314=CARTESIAN_POINT('Ctrl Pts',(-0.237348630414619,0.0184268956074038,
-4.50188137310879));
#28315=CARTESIAN_POINT('Ctrl Pts',(-0.237180885702784,0.000217072097893506,
-4.5006589891905));
#28316=CARTESIAN_POINT('Ctrl Pts',(-0.237136177256987,0.000217231692762269,
-4.5809410108095));
#28317=CARTESIAN_POINT('Ctrl Pts',(-0.236599623077143,-0.0590033993122846,
-4.57696757750464));
#28318=CARTESIAN_POINT('Ctrl Pts',(-0.184170554683796,-0.197991731059171,
-4.56769894905828));
#28319=CARTESIAN_POINT('Ctrl Pts',(0.0491753813860615,-0.276035885831286,
-4.55313512547041));
#28320=CARTESIAN_POINT('Ctrl Pts',(0.258642791859093,-0.108249409330772,
-4.53724954004591));
#28321=CARTESIAN_POINT('Ctrl Pts',(0.231132711334074,0.158718928148119,
-4.5213639546214));
#28322=CARTESIAN_POINT('Ctrl Pts',(-0.00814917085540682,0.280263482129757,
-4.50547836919689));
#28323=CARTESIAN_POINT('Ctrl Pts',(-0.204777283366198,0.165549369232331,
-4.49200405459293));
#28324=CARTESIAN_POINT('Ctrl Pts',(-0.236705400940218,0.0430794593642273,
-4.48382493513046));
#28325=CARTESIAN_POINT('Ctrl Pts',(-0.236798869759374,-5.74984565626727E-5,
-4.4809410108095));
#28326=CARTESIAN_POINT('Origin',(0.,0.,-6.1506589891905));
#28327=CARTESIAN_POINT('',(-0.236908709036994,-0.00016298456995,-4.7006589891905));
#28328=CARTESIAN_POINT('',(-0.237543953866199,-6.55533299058764E-5,-4.6809410108095));
#28329=CARTESIAN_POINT('',(-0.237175,1.98931295048561E-15,-6.1506589891905));
#28330=CARTESIAN_POINT('Ctrl Pts',(-0.236908709036994,-0.000162984569950002,
-4.7006589891905));
#28331=CARTESIAN_POINT('Ctrl Pts',(-0.237088327609357,-0.0285786996968505,
-4.69875704814015));
#28332=CARTESIAN_POINT('Ctrl Pts',(-0.21920122513728,-0.135888036726437,
-4.6915599119483));
#28333=CARTESIAN_POINT('Ctrl Pts',(-0.0595908711013016,-0.273976209565238,
-4.67906758061494));
#28334=CARTESIAN_POINT('Ctrl Pts',(0.197973181209263,-0.198546354406802,
-4.66318199519043));
#28335=CARTESIAN_POINT('Ctrl Pts',(0.274147342733956,0.0587985526884655,
-4.64729640976593));
#28336=CARTESIAN_POINT('Ctrl Pts',(0.0991382063290872,0.262270187730513,
-4.63141082434142));
#28337=CARTESIAN_POINT('Ctrl Pts',(-0.161018645402043,0.226228534144202,
-4.61586501748294));
#28338=CARTESIAN_POINT('Ctrl Pts',(-0.237163185334549,0.0734532857575236,
-4.60561440576597));
#28339=CARTESIAN_POINT('Ctrl Pts',(-0.237523476840667,-9.09874636312079E-5,
-4.6006589891905));
#28340=CARTESIAN_POINT('Ctrl Pts',(-0.237543953866199,-6.55533299058803E-5,
-4.6809410108095));
#28341=CARTESIAN_POINT('Ctrl Pts',(-0.237557049209306,-0.00363256502421958,
-4.68070061016182));
#28342=CARTESIAN_POINT('Ctrl Pts',(-0.235867300532786,-0.0857558329936854,
-4.67516501437264));
#28343=CARTESIAN_POINT('Ctrl Pts',(-0.141103532512842,-0.242288715200532,
-4.66433422344196));
#28344=CARTESIAN_POINT('Ctrl Pts',(0.127170996645068,-0.249883104697832,
-4.64844863801745));
#28345=CARTESIAN_POINT('Ctrl Pts',(0.278927050665701,-0.0285259322031912,
-4.63256305259295));
#28346=CARTESIAN_POINT('Ctrl Pts',(0.175120472675097,0.218967688144114,
-4.61667746716844));
#28347=CARTESIAN_POINT('Ctrl Pts',(-0.0891375524199996,0.265835522738591,
-4.60079188174394));
#28348=CARTESIAN_POINT('Ctrl Pts',(-0.226054472369514,0.118335830510633,
-4.58887972962428));
#28349=CARTESIAN_POINT('Ctrl Pts',(-0.237314661903335,0.0199169633854095,
-4.58226277264614));
#28350=CARTESIAN_POINT('Ctrl Pts',(-0.237136177256987,0.000217231692762269,
-4.5809410108095));
#28351=CARTESIAN_POINT('Origin',(0.,0.,-6.1506589891905));
#28352=CARTESIAN_POINT('',(-0.236931796274552,0.000174130487424274,-4.8006589891905));
#28353=CARTESIAN_POINT('',(-0.236941539607102,-0.000178305245891713,-4.7809410108095));
#28354=CARTESIAN_POINT('',(-0.237175,1.98931295048561E-15,-6.1506589891905));
#28355=CARTESIAN_POINT('Ctrl Pts',(-0.236931796274552,0.000174130487424283,
-4.8006589891905));
#28356=CARTESIAN_POINT('Ctrl Pts',(-0.236580090821685,-0.0515682065233269,
-4.79719488565583));
#28357=CARTESIAN_POINT('Ctrl Pts',(-0.194440311842266,-0.18292465151328,
-4.78843558697966));
#28358=CARTESIAN_POINT('Ctrl Pts',(0.0224884069277866,-0.279478634031651,
-4.77438109316199));
#28359=CARTESIAN_POINT('Ctrl Pts',(0.247075054914963,-0.13254415326643,
-4.75849550773747));
#28360=CARTESIAN_POINT('Ctrl Pts',(0.245282973454107,0.135831874977338,
-4.74260992231297));
#28361=CARTESIAN_POINT('Ctrl Pts',(0.0187541296969196,0.279754031151758,
-4.72672433688846));
#28362=CARTESIAN_POINT('Ctrl Pts',(-0.19577887178785,0.180812998027858,
-4.71274069251431));
#28363=CARTESIAN_POINT('Ctrl Pts',(-0.23658825144163,0.0505335086728689,
-4.70405224328166));
#28364=CARTESIAN_POINT('Ctrl Pts',(-0.236908709036994,-0.000162984569950002,
-4.7006589891905));
#28365=CARTESIAN_POINT('Ctrl Pts',(-0.236941539607102,-0.000178305245891745,
-4.7809410108095));
#28366=CARTESIAN_POINT('Ctrl Pts',(-0.237129442313695,-0.0270998926955989,
-4.7791384476775));
#28367=CARTESIAN_POINT('Ctrl Pts',(-0.220459184495624,-0.132880385692709,
-4.772040689404));
#28368=CARTESIAN_POINT('Ctrl Pts',(-0.0647123167632992,-0.272811921404205,
-4.759647735989));
#28369=CARTESIAN_POINT('Ctrl Pts',(0.194219427751849,-0.202219787075528,
-4.7437621505645));
#28370=CARTESIAN_POINT('Ctrl Pts',(0.275200600511704,0.0536531255298783,
-4.72787656513998));
#28371=CARTESIAN_POINT('Ctrl Pts',(0.104033444057923,0.260367184795962,
-4.71199097971549));
#28372=CARTESIAN_POINT('Ctrl Pts',(-0.158419955632031,0.229005698543907,
-4.69634579493865));
#28373=CARTESIAN_POINT('Ctrl Pts',(-0.23726860407462,0.0749363705253955,
-4.68599580530332));
#28374=CARTESIAN_POINT('Ctrl Pts',(-0.237543953866199,-6.55533299058803E-5,
-4.6809410108095));
#28375=CARTESIAN_POINT('Origin',(0.,0.,-6.1506589891905));
#28376=CARTESIAN_POINT('',(-0.237538693477751,7.2995197219953E-5,-4.9006589891905));
#28377=CARTESIAN_POINT('',(-0.236899879648722,0.000158196596847071,-4.88094101080949));
#28378=CARTESIAN_POINT('',(-0.237175,1.98931295048561E-15,-6.1506589891905));
#28379=CARTESIAN_POINT('Ctrl Pts',(-0.237538693477751,7.29951972199385E-5,
-4.9006589891905));
#28380=CARTESIAN_POINT('Ctrl Pts',(-0.237237326520422,-0.0745100491991757,
-4.89563272317151));
#28381=CARTESIAN_POINT('Ctrl Pts',(-0.159170881587928,-0.228210259049412,
-4.88531126201102));
#28382=CARTESIAN_POINT('Ctrl Pts',(0.102631828995819,-0.260922867919469,
-4.86969460570902));
#28383=CARTESIAN_POINT('Ctrl Pts',(0.274908115786522,-0.0551322337752745,
-4.85380902028452));
#28384=CARTESIAN_POINT('Ctrl Pts',(0.195304058006928,0.201172463951639,
-4.83792343486001));
#28385=CARTESIAN_POINT('Ctrl Pts',(-0.0632443473631996,0.273155977150327,
-4.82203784943551));
#28386=CARTESIAN_POINT('Ctrl Pts',(-0.220101702028949,0.13374379324399,
-4.80961636754567));
#28387=CARTESIAN_POINT('Ctrl Pts',(-0.237117704373537,0.0275246291287032,
-4.80249008079733));
#28388=CARTESIAN_POINT('Ctrl Pts',(-0.236931796274552,0.000174130487424283,
-4.8006589891905));
#28389=CARTESIAN_POINT('Ctrl Pts',(-0.236899879648722,0.000158196596847054,
-4.88094101080949));
#28390=CARTESIAN_POINT('Ctrl Pts',(-0.236592171127761,-0.050116767091128,
-4.87757628519318));
#28391=CARTESIAN_POINT('Ctrl Pts',(-0.196311764217322,-0.179961785169845,
-4.86891636443536));
#28392=CARTESIAN_POINT('Ctrl Pts',(0.0172494902941208,-0.279850823628805,
-4.85496124853605));
#28393=CARTESIAN_POINT('Ctrl Pts',(0.244548985077421,-0.137148905568842,
-4.83907566311153));
#28394=CARTESIAN_POINT('Ctrl Pts',(0.247784223156673,0.131213593639424,
-4.82319007768704));
#28395=CARTESIAN_POINT('Ctrl Pts',(0.0239909672635905,0.279353650219367,
-4.80730449226251));
#28396=CARTESIAN_POINT('Ctrl Pts',(-0.193895200773842,0.183773975398,-4.79322146997002));
#28397=CARTESIAN_POINT('Ctrl Pts',(-0.236577460815037,0.0519847487989422,
-4.78443364281901));
#28398=CARTESIAN_POINT('Ctrl Pts',(-0.236941539607102,-0.000178305245891745,
-4.7809410108095));
#28399=CARTESIAN_POINT('Origin',(0.,0.,-6.1506589891905));
#28400=CARTESIAN_POINT('',(-0.237148948645665,-0.00021749005109032,-5.0006589891905));
#28401=CARTESIAN_POINT('',(-0.237516529348539,9.80111424561253E-5,-4.9809410108095));
#28402=CARTESIAN_POINT('',(-0.237175,1.98931295048561E-15,-6.1506589891905));
#28403=CARTESIAN_POINT('Ctrl Pts',(-0.237148948645665,-0.000217490051090299,
-5.0006589891905));
#28404=CARTESIAN_POINT('Ctrl Pts',(-0.237324608020506,-0.0194893848684046,
-4.99936575582869));
#28405=CARTESIAN_POINT('Ctrl Pts',(-0.226361561945563,-0.117473530672288,
-4.99277732732538));
#28406=CARTESIAN_POINT('Ctrl Pts',(-0.0905657887914961,-0.265352356738962,
-4.98089370368057));
#28407=CARTESIAN_POINT('Ctrl Pts',(0.173940457270164,-0.219906236043896,
-4.96500811825607));
#28408=CARTESIAN_POINT('Ctrl Pts',(0.279076427243118,0.0270256005218002,
-4.94912253283156));
#28409=CARTESIAN_POINT('Ctrl Pts',(0.128512901206904,0.249195645125937,
-4.93323694740706));
#28410=CARTESIAN_POINT('Ctrl Pts',(-0.139798599439343,0.243044002026681,
-4.91735136198254));
#28411=CARTESIAN_POINT('Ctrl Pts',(-0.235654574442953,0.0866120031589777,
-4.90649204257703));
#28412=CARTESIAN_POINT('Ctrl Pts',(-0.237554818042404,0.00406354257534346,
-4.90092791831301));
#28413=CARTESIAN_POINT('Ctrl Pts',(-0.237538693477751,7.29951972199385E-5,
-4.9006589891905));
#28414=CARTESIAN_POINT('Ctrl Pts',(-0.237516529348539,9.80111424561452E-5,
-4.9809410108095));
#28415=CARTESIAN_POINT('Ctrl Pts',(-0.237134737314428,-0.0730285328966137,
-4.97601412270886));
#28416=CARTESIAN_POINT('Ctrl Pts',(-0.161755788795796,-0.225428088374244,
-4.96579203946672));
#28417=CARTESIAN_POINT('Ctrl Pts',(0.0977264198891994,-0.262799496302347,
-4.95027476108308));
#28418=CARTESIAN_POINT('Ctrl Pts',(0.273827179714107,-0.0602719175980483,
-4.93438917565858));
#28419=CARTESIAN_POINT('Ctrl Pts',(0.199037986065754,0.197478881159522,
-4.91850359023406));
#28420=CARTESIAN_POINT('Ctrl Pts',(-0.0581167094863374,0.274292683970259,
-4.90261800480957));
#28421=CARTESIAN_POINT('Ctrl Pts',(-0.218833502316203,0.136751428414759,
-4.89009714500137));
#28422=CARTESIAN_POINT('Ctrl Pts',(-0.237076423590217,0.0290028324889566,
-4.88287148033468));
#28423=CARTESIAN_POINT('Ctrl Pts',(-0.236899879648722,0.000158196596847054,
-4.88094101080949));
#28424=CARTESIAN_POINT('Origin',(0.,0.,-6.1506589891905));
#28425=CARTESIAN_POINT('',(-0.236795980310558,5.06907052245788E-5,-5.1006589891905));
#28426=CARTESIAN_POINT('',(-0.237193800648222,-0.000216474445068449,-5.0809410108095));
#28427=CARTESIAN_POINT('',(-0.237175,1.98931295048561E-15,-6.1506589891905));
#28428=CARTESIAN_POINT('Ctrl Pts',(-0.236795980310558,5.06907052245723E-5,
-5.1006589891905));
#28429=CARTESIAN_POINT('Ctrl Pts',(-0.23671444927506,-0.0426608529623053,
-5.09780359334437));
#28430=CARTESIAN_POINT('Ctrl Pts',(-0.205249568998764,-0.164690913697368,
-5.08965300235675));
#28431=CARTESIAN_POINT('Ctrl Pts',(-0.00965616049258788,-0.280215620354914,
-5.07620721622762));
#28432=CARTESIAN_POINT('Ctrl Pts',(0.230275874140234,-0.159959548371763,
-5.0603216308031));
#28433=CARTESIAN_POINT('Ctrl Pts',(0.25922117104535,0.106857006360016,-5.04443604537861));
#28434=CARTESIAN_POINT('Ctrl Pts',(0.0506590458941416,0.275767467978807,
-5.02855045995409));
#28435=CARTESIAN_POINT('Ctrl Pts',(-0.183561113561564,0.198828830534759,
-5.0139581078914));
#28436=CARTESIAN_POINT('Ctrl Pts',(-0.23660536376368,0.0594201505781383,
-5.0046609509702));
#28437=CARTESIAN_POINT('Ctrl Pts',(-0.237148948645665,-0.000217490051090299,
-5.0006589891905));
#28438=CARTESIAN_POINT('Ctrl Pts',(-0.237193800648222,-0.000216474445068456,
-5.0809410108095));
#28439=CARTESIAN_POINT('Ctrl Pts',(-0.237358018819269,-0.0179988291517084,
-5.07974715536605));
#28440=CARTESIAN_POINT('Ctrl Pts',(-0.22741001665069,-0.11447059654328,
-5.07325810478109));
#28441=CARTESIAN_POINT('Ctrl Pts',(-0.0955202636039318,-0.26360938458667,
-5.06147385905463));
#28442=CARTESIAN_POINT('Ctrl Pts',(0.169790825062137,-0.223125758544025,
-5.04558827363013));
#28443=CARTESIAN_POINT('Ctrl Pts',(0.279533674503372,0.0217934214792116,
-5.02970268820562));
#28444=CARTESIAN_POINT('Ctrl Pts',(0.133158082146451,0.246744713337908,
-5.01381710278111));
#28445=CARTESIAN_POINT('Ctrl Pts',(-0.135221560608942,0.245619946151793,
-4.99793151735661));
#28446=CARTESIAN_POINT('Ctrl Pts',(-0.234894750020545,0.0895960082762632,
-4.98697282003273));
#28447=CARTESIAN_POINT('Ctrl Pts',(-0.23754507001994,0.00556454914650678,
-4.98130931785036));
#28448=CARTESIAN_POINT('Ctrl Pts',(-0.237516529348539,9.80111424561452E-5,
-4.9809410108095));
#28449=CARTESIAN_POINT('Origin',(0.,0.,-6.1506589891905));
#28450=CARTESIAN_POINT('',(-0.237335164775886,0.000193322802161542,-5.2006589891905));
#28451=CARTESIAN_POINT('',(-0.236788752274853,2.66210406855288E-5,-5.1809410108095));
#28452=CARTESIAN_POINT('',(-0.237175,1.98931295048561E-15,-6.1506589891905));
#28453=CARTESIAN_POINT('Ctrl Pts',(-0.237335164775886,0.00019332280216155,
-5.2006589891905));
#28454=CARTESIAN_POINT('Ctrl Pts',(-0.236755294092649,-0.0655048792155798,
-5.19624143086006));
#28455=CARTESIAN_POINT('Ctrl Pts',(-0.174259926607873,-0.210921685958696,
-5.18652867738811));
#28456=CARTESIAN_POINT('Ctrl Pts',(0.0720846932421861,-0.270957251843399,
-5.17152072877465));
#28457=CARTESIAN_POINT('Ctrl Pts',(0.266788591915922,-0.0862431594381096,
-5.15563514335015));
#28458=CARTESIAN_POINT('Ctrl Pts',(0.217051535229177,0.177489905011538,
-5.13974955792564));
#28459=CARTESIAN_POINT('Ctrl Pts',(-0.0315556614918893,0.278600566320595,
-5.12386397250114));
#28460=CARTESIAN_POINT('Ctrl Pts',(-0.211760853398221,0.152156333831052,
-5.11083378292275));
#28461=CARTESIAN_POINT('Ctrl Pts',(-0.236865644684144,0.0365456636476937,
-5.10309878848588));
#28462=CARTESIAN_POINT('Ctrl Pts',(-0.236795980310558,5.06907052245723E-5,
-5.1006589891905));
#28463=CARTESIAN_POINT('Ctrl Pts',(-0.236788752274853,2.66210406855358E-5,
-5.1809410108095));
#28464=CARTESIAN_POINT('Ctrl Pts',(-0.236747495401724,-0.0412015421027071,
-5.17818499288173));
#28465=CARTESIAN_POINT('Ctrl Pts',(-0.206869023211992,-0.161698214308556,
-5.17013377981245));
#28466=CARTESIAN_POINT('Ctrl Pts',(-0.0149032407667099,-0.279985574299422,
-5.15678737160167));
#28467=CARTESIAN_POINT('Ctrl Pts',(0.22723922911572,-0.164244820776854,
-5.14090178617716));
#28468=CARTESIAN_POINT('Ctrl Pts',(0.261177240698333,0.101982730608336,
-5.12501620075266));
#28469=CARTESIAN_POINT('Ctrl Pts',(0.0558156114071165,0.274770169276757,
-5.10913061532815));
#28470=CARTESIAN_POINT('Ctrl Pts',(-0.181409236364921,0.201738255249697,
-5.0944388853471));
#28471=CARTESIAN_POINT('Ctrl Pts',(-0.236629649847762,0.0608725608171928,
-5.08504235050755));
#28472=CARTESIAN_POINT('Ctrl Pts',(-0.237193800648222,-0.000216474445068456,
-5.0809410108095));
#28473=CARTESIAN_POINT('Origin',(0.,0.,-6.1506589891905));
#28474=CARTESIAN_POINT('',(-0.237414200045941,-0.000164802835073178,-5.3006589891905));
#28475=CARTESIAN_POINT('',(-0.237291647891957,0.000203839981857537,-5.2809410108095));
#28476=CARTESIAN_POINT('',(-0.237175,1.98931295048561E-15,-6.1506589891905));
#28477=CARTESIAN_POINT('Ctrl Pts',(-0.237414200045941,-0.000164802835073157,
-5.3006589891905));
#28478=CARTESIAN_POINT('Ctrl Pts',(-0.237494743202661,-0.0103362946657776,
-5.29997446351724));
#28479=CARTESIAN_POINT('Ctrl Pts',(-0.232279536649386,-0.0991068806287269,
-5.29399474270247));
#28480=CARTESIAN_POINT('Ctrl Pts',(-0.120349718205416,-0.253238979334194,
-5.28271982674621));
#28481=CARTESIAN_POINT('Ctrl Pts',(0.147620323834129,-0.23837423375326,
-5.2668342413217));
#28482=CARTESIAN_POINT('Ctrl Pts',(0.280335508349595,-0.00510275266119098,
-5.25094865589719));
#28483=CARTESIAN_POINT('Ctrl Pts',(0.156197583103769,0.232844047291076,
-5.23506307047268));
#28484=CARTESIAN_POINT('Ctrl Pts',(-0.111053981914616,0.257451060256615,
-5.21917748504818));
#28485=CARTESIAN_POINT('Ctrl Pts',(-0.230530796392364,0.104926093377206,
-5.20770945795412));
#28486=CARTESIAN_POINT('Ctrl Pts',(-0.237450367749835,0.0132455919965611,
-5.20153662600156));
#28487=CARTESIAN_POINT('Ctrl Pts',(-0.237335164775886,0.00019332280216155,
-5.2006589891905));
#28488=CARTESIAN_POINT('Ctrl Pts',(-0.237291647891957,0.000203839981857532,
-5.2809410108095));
#28489=CARTESIAN_POINT('Ctrl Pts',(-0.236707472807153,-0.0640468622466563,
-5.27662283039741));
#28490=CARTESIAN_POINT('Ctrl Pts',(-0.176556678251362,-0.20804859565348,
-5.26700945484381));
#28491=CARTESIAN_POINT('Ctrl Pts',(0.0669966887508262,-0.272259934800463,
-5.25210088414871));
#28492=CARTESIAN_POINT('Ctrl Pts',(0.265126335755849,-0.0912252952300192,
-5.23621529872421));
#28493=CARTESIAN_POINT('Ctrl Pts',(0.220338044111505,0.173393121888511,
-5.2203297132997));
#28494=CARTESIAN_POINT('Ctrl Pts',(-0.0263316009223782,0.279142750566788,
-5.2044441278752));
#28495=CARTESIAN_POINT('Ctrl Pts',(-0.210265822348046,0.155157722278446,
-5.19131456037846));
#28496=CARTESIAN_POINT('Ctrl Pts',(-0.236826763098768,0.0380109938427312,
-5.18348018802323));
#28497=CARTESIAN_POINT('Ctrl Pts',(-0.236788752274853,2.66210406855358E-5,
-5.1809410108095));
#28498=CARTESIAN_POINT('Origin',(0.,0.,-6.1506589891905));
#28499=CARTESIAN_POINT('',(-0.236822660016195,-9.54250159434449E-5,-5.4006589891905));
#28500=CARTESIAN_POINT('',(-0.237450728442205,-0.000146260240270479,-5.3809410108095));
#28501=CARTESIAN_POINT('',(-0.237175,1.98931295048561E-15,-6.1506589891905));
#28502=CARTESIAN_POINT('Ctrl Pts',(-0.236822660016195,-9.54250159434407E-5,
-5.4006589891905));
#28503=CARTESIAN_POINT('Ctrl Pts',(-0.236944197811255,-0.0336923528614689,
-5.39841230103292));
#28504=CARTESIAN_POINT('Ctrl Pts',(-0.214557208673931,-0.146318914545383,
-5.39087041773384));
#28505=CARTESIAN_POINT('Ctrl Pts',(-0.0416737442683253,-0.27726762228038,
-5.37803333929325));
#28506=CARTESIAN_POINT('Ctrl Pts',(0.21044844318329,-0.185271390365794,
-5.36214775386874));
#28507=CARTESIAN_POINT('Ctrl Pts',(0.269750472409913,0.0764769112933738,
-5.34626216844423));
#28508=CARTESIAN_POINT('Ctrl Pts',(0.0818977687025324,0.268154415976868,
-5.33037658301972));
#28509=CARTESIAN_POINT('Ctrl Pts',(-0.169664305922363,0.216467104244653,
-5.31517552326848));
#28510=CARTESIAN_POINT('Ctrl Pts',(-0.236871696107715,0.0683459757405056,
-5.30526965865874));
#28511=CARTESIAN_POINT('Ctrl Pts',(-0.237414200045941,-0.000164802835073157,
-5.3006589891905));
#28512=CARTESIAN_POINT('Ctrl Pts',(-0.237450728442205,-0.000146260240270466,
-5.3809410108095));
#28513=CARTESIAN_POINT('Ctrl Pts',(-0.237513641523012,-0.0088375729951032,
-5.38035586305459));
#28514=CARTESIAN_POINT('Ctrl Pts',(-0.233134227691199,-0.0961153864525537,
-5.37447552015817));
#28515=CARTESIAN_POINT('Ctrl Pts',(-0.125072068190222,-0.250940244201183,
-5.36329998212027));
#28516=CARTESIAN_POINT('Ctrl Pts',(0.143129382745379,-0.241097507652099,
-5.34741439669575));
#28517=CARTESIAN_POINT('Ctrl Pts',(0.280190732047764,-0.0103528776514324,
-5.33152881127125));
#28518=CARTESIAN_POINT('Ctrl Pts',(0.160531620654842,0.229877417705736,
-5.31564322584674));
#28519=CARTESIAN_POINT('Ctrl Pts',(-0.10621212594168,0.259486054931813,
-5.29975764042223));
#28520=CARTESIAN_POINT('Ctrl Pts',(-0.229584869499672,0.107923695599517,
-5.28819023540982));
#28521=CARTESIAN_POINT('Ctrl Pts',(-0.237423821077868,0.0147409543359568,
-5.28191802553891));
#28522=CARTESIAN_POINT('Ctrl Pts',(-0.237291647891957,0.000203839981857532,
-5.2809410108095));
#28523=CARTESIAN_POINT('Origin',(0.,0.,-6.1506589891905));
#28524=CARTESIAN_POINT('',(-0.237064417961372,0.000211057165585043,-5.5006589891905));
#28525=CARTESIAN_POINT('',(-0.236842640230931,-0.000116843745555151,-5.4809410108095));
#28526=CARTESIAN_POINT('',(-0.237175,1.98931295048561E-15,-6.1506589891905));
#28527=CARTESIAN_POINT('Ctrl Pts',(-0.237064417961372,0.000211057165585036,
-5.5006589891905));
#28528=CARTESIAN_POINT('Ctrl Pts',(-0.236576849557631,-0.0566003236648596,
-5.4968501385486));
#28529=CARTESIAN_POINT('Ctrl Pts',(-0.187614909420263,-0.193147175570037,
-5.48774609276519));
#28530=CARTESIAN_POINT('Ctrl Pts',(0.040589605444914,-0.277428403839015,
-5.47334685184029));
#28531=CARTESIAN_POINT('Ctrl Pts',(0.255160656210713,-0.116219941698528,
-5.45746126641578));
#28532=CARTESIAN_POINT('Ctrl Pts',(0.235944669357195,0.151473259449223,
-5.44157568099128));
#28533=CARTESIAN_POINT('Ctrl Pts',(0.000547998106158669,0.280381409912451,
-5.42569009556676));
#28534=CARTESIAN_POINT('Ctrl Pts',(-0.201987756818871,0.170495515579157,
-5.41205119829984));
#28535=CARTESIAN_POINT('Ctrl Pts',(-0.236657746689972,0.0454918848337113,
-5.40370749617442));
#28536=CARTESIAN_POINT('Ctrl Pts',(-0.236822660016195,-9.54250159434407E-5,
-5.4006589891905));
#28537=CARTESIAN_POINT('Ctrl Pts',(-0.236842640230931,-0.000116843745555185,
-5.4809410108095));
#28538=CARTESIAN_POINT('Ctrl Pts',(-0.236985574897071,-0.0322208987592947,
-5.47879370057027));
#28539=CARTESIAN_POINT('Ctrl Pts',(-0.21594113561778,-0.143312950842703,
-5.47135119518954));
#28540=CARTESIAN_POINT('Ctrl Pts',(-0.0468599862874815,-0.276438365800292,
-5.45861349466731));
#28541=CARTESIAN_POINT('Ctrl Pts',(0.206941156468481,-0.189180829262909,
-5.4427279092428));
#28542=CARTESIAN_POINT('Ctrl Pts',(0.271135638657325,0.0714107404456813,
-5.42684232381829));
#28543=CARTESIAN_POINT('Ctrl Pts',(0.0869062505835863,0.266573314513364,
-5.41095673839378));
#28544=CARTESIAN_POINT('Ctrl Pts',(-0.167230487480177,0.219300088354176,
-5.39565630072419));
#28545=CARTESIAN_POINT('Ctrl Pts',(-0.236944320292551,0.0698129843838412,
-5.38565105819609));
#28546=CARTESIAN_POINT('Ctrl Pts',(-0.237450728442205,-0.000146260240270466,
-5.3809410108095));
#28547=CARTESIAN_POINT('Origin',(0.,0.,-6.1506589891905));
#28548=CARTESIAN_POINT('',(-0.237563686191593,-2.10269292758361E-5,-5.6006589891905));
#28549=CARTESIAN_POINT('',(-0.237023234876043,0.000203592057815866,-5.5809410108095));
#28550=CARTESIAN_POINT('',(-0.237175,1.98931295048561E-15,-6.1506589891905));
#28551=CARTESIAN_POINT('Ctrl Pts',(-0.237563686191593,-2.10269292758463E-5,
-5.6006589891905));
#28552=CARTESIAN_POINT('Ctrl Pts',(-0.237565111147283,-0.00114574716038694,
-5.60058317120578));
#28553=CARTESIAN_POINT('Ctrl Pts',(-0.237048263617325,-0.080820577600737,
-5.59521215807956));
#28554=CARTESIAN_POINT('Ctrl Pts',(-0.14855098481485,-0.237795374612464,
-5.58454594981183));
#28555=CARTESIAN_POINT('Ctrl Pts',(0.119358904639683,-0.253707483593214,
-5.56866036438733));
#28556=CARTESIAN_POINT('Ctrl Pts',(0.277908028472834,-0.0371640019089366,
-5.55277477896282));
#28557=CARTESIAN_POINT('Ctrl Pts',(0.181828183730025,0.21343042641883,-5.53688919353832));
#28558=CARTESIAN_POINT('Ctrl Pts',(-0.0808489454790468,0.268472500164499,
-5.52100360811381));
#28559=CARTESIAN_POINT('Ctrl Pts',(-0.224229150548578,0.123312428819558,
-5.5089268733312));
#28560=CARTESIAN_POINT('Ctrl Pts',(-0.237254683919062,0.0223808116009525,
-5.5021453336901));
#28561=CARTESIAN_POINT('Ctrl Pts',(-0.237064417961372,0.000211057165585036,
-5.5006589891905));
#28562=CARTESIAN_POINT('Ctrl Pts',(-0.237023234876043,0.000203592057815862,
-5.5809410108095));
#28563=CARTESIAN_POINT('Ctrl Pts',(-0.236571091847558,-0.0551498509335718,
-5.57723153808595));
#28564=CARTESIAN_POINT('Ctrl Pts',(-0.189636057293001,-0.190210103257596,
-5.56822687022089));
#28565=CARTESIAN_POINT('Ctrl Pts',(0.0353859155308252,-0.278140010402117,
-5.55392700721436));
#28566=CARTESIAN_POINT('Ctrl Pts',(0.252938939516514,-0.120979011722138,
-5.53804142178983));
#28567=CARTESIAN_POINT('Ctrl Pts',(0.238740539723166,0.147027150870172,
-5.52215583636534));
#28568=CARTESIAN_POINT('Ctrl Pts',(0.0057997821945244,0.280321941574533,
-5.50627025094082));
#28569=CARTESIAN_POINT('Ctrl Pts',(-0.200249211686888,0.173476183501598,
-5.49253197575555));
#28570=CARTESIAN_POINT('Ctrl Pts',(-0.23663310279692,0.0469466258142949,
-5.48408889571177));
#28571=CARTESIAN_POINT('Ctrl Pts',(-0.236842640230931,-0.000116843745555185,
-5.4809410108095));
#28572=CARTESIAN_POINT('Origin',(0.,0.,-6.1506589891905));
#28573=CARTESIAN_POINT('',(-0.237002443247224,-0.000198590235900253,-5.7006589891905));
#28574=CARTESIAN_POINT('',(-0.237565764759064,6.5451087111932E-6,-5.6809410108095));
#28575=CARTESIAN_POINT('',(-0.237175,1.98931295048561E-15,-6.1506589891905));
#28576=CARTESIAN_POINT('Ctrl Pts',(-0.237002443247224,-0.00019859023590026,
-5.7006589891905));
#28577=CARTESIAN_POINT('Ctrl Pts',(-0.237195969987065,-0.0246462657790171,
-5.69902100872146));
#28578=CARTESIAN_POINT('Ctrl Pts',(-0.222465081710047,-0.127899829220746,
-5.69208783311092));
#28579=CARTESIAN_POINT('Ctrl Pts',(-0.0731432950877003,-0.270673402752768,
-5.67985946235888));
#28580=CARTESIAN_POINT('Ctrl Pts',(0.187853502754299,-0.208146817550068,
-5.66397387693437));
#28581=CARTESIAN_POINT('Ctrl Pts',(0.276732411920541,0.0450911054647064,
-5.64808829150987));
#28582=CARTESIAN_POINT('Ctrl Pts',(0.112059492160603,0.257014990163246,
-5.63220270608536));
#28583=CARTESIAN_POINT('Ctrl Pts',(-0.154010242816776,0.23356529091088,
-5.61639293864557));
#28584=CARTESIAN_POINT('Ctrl Pts',(-0.237465590980955,0.0774057090053768,
-5.60587836634729));
#28585=CARTESIAN_POINT('Ctrl Pts',(-0.237563686191593,-2.10269292758463E-5,
-5.6006589891905));
#28586=CARTESIAN_POINT('Ctrl Pts',(-0.237565764759064,6.54510871119022E-6,
-5.6809410108095));
#28587=CARTESIAN_POINT('Ctrl Pts',(-0.2375341250678,-0.0781935536318626,
-5.67566937560163));
#28588=CARTESIAN_POINT('Ctrl Pts',(-0.152582282569065,-0.235002143286345,
-5.66510254525225));
#28589=CARTESIAN_POINT('Ctrl Pts',(0.114585712811833,-0.255898696670898,
-5.6492405197614));
#28590=CARTESIAN_POINT('Ctrl Pts',(0.277163132557144,-0.0423630307669099,
-5.63335493433687));
#28591=CARTESIAN_POINT('Ctrl Pts',(0.18579408296189,0.209987111717646,-5.61746934891238));
#28592=CARTESIAN_POINT('Ctrl Pts',(-0.0758059453271951,0.269939784166574,
-5.60158376348786));
#28593=CARTESIAN_POINT('Ctrl Pts',(-0.223082036136281,0.126318675930788,
-5.58940765078691));
#28594=CARTESIAN_POINT('Ctrl Pts',(-0.237216516614399,0.0238660373711741,
-5.58252673322745));
#28595=CARTESIAN_POINT('Ctrl Pts',(-0.237023234876043,0.000203592057815862,
-5.5809410108095));
#28596=CARTESIAN_POINT('Origin',(0.,0.,-6.1506589891905));
#28597=CARTESIAN_POINT('',(-0.236854733944756,0.000127784916100184,-5.8006589891905));
#28598=CARTESIAN_POINT('',(-0.237042509219701,-0.000207466451680183,-5.7809410108095));
#28599=CARTESIAN_POINT('',(-0.237175,1.98931295048561E-15,-6.1506589891905));
#28600=CARTESIAN_POINT('Ctrl Pts',(-0.236854733944756,0.000127784916100174,
-5.8006589891905));
#28601=CARTESIAN_POINT('Ctrl Pts',(-0.236621530291177,-0.0477109510420727,
-5.79745884623714));
#28602=CARTESIAN_POINT('Ctrl Pts',(-0.199318547468919,-0.175041983926161,
-5.78896350814228));
#28603=CARTESIAN_POINT('Ctrl Pts',(0.00856079809868226,-0.280250974663184,
-5.77517297490592));
#28604=CARTESIAN_POINT('Ctrl Pts',(0.240177193574594,-0.144668499352843,
-5.75928738948141));
#28605=CARTESIAN_POINT('Ctrl Pts',(0.251735020445761,0.123464726945526,
-5.74340180405691));
#28606=CARTESIAN_POINT('Ctrl Pts',(0.0326444435734673,0.278475054243476,
-5.72751621863239));
#28607=CARTESIAN_POINT('Ctrl Pts',(-0.190681354952407,0.188662352749473,
-5.71326861367693));
#28608=CARTESIAN_POINT('Ctrl Pts',(-0.236570344790718,0.0543871630095648,
-5.70431620386297));
#28609=CARTESIAN_POINT('Ctrl Pts',(-0.237002443247224,-0.00019859023590026,
-5.7006589891905));
#28610=CARTESIAN_POINT('Ctrl Pts',(-0.237042509219701,-0.000207466451680186,
-5.7809410108095));
#28611=CARTESIAN_POINT('Ctrl Pts',(-0.23723477238687,-0.0231620637174002,
-5.77940240825881));
#28612=CARTESIAN_POINT('Ctrl Pts',(-0.223630207594125,-0.12489320512256,
-5.77256861056662));
#28613=CARTESIAN_POINT('Ctrl Pts',(-0.0782004847763744,-0.269255812835206,
-5.76043961773294));
#28614=CARTESIAN_POINT('Ctrl Pts',(0.183921690703183,-0.211629026318924,
-5.74455403230843));
#28615=CARTESIAN_POINT('Ctrl Pts',(0.277528462365728,0.0398996699056295,
-5.72866844688392));
#28616=CARTESIAN_POINT('Ctrl Pts',(0.116854024514864,0.254870874359421,
-5.71278286145941));
#28617=CARTESIAN_POINT('Ctrl Pts',(-0.150886114490242,0.236320565513686,
-5.69689727603491));
#28618=CARTESIAN_POINT('Ctrl Pts',(-0.237406868651535,0.0792549843919946,
-5.68628332581827));
#28619=CARTESIAN_POINT('Ctrl Pts',(-0.237565906162821,0.000356036123144353,
-5.68096457074313));
#28620=CARTESIAN_POINT('Ctrl Pts',(-0.237565764759064,6.54510871119022E-6,
-5.6809410108095));
#28621=CARTESIAN_POINT('Origin',(0.,0.,-6.1506589891905));
#28622=CARTESIAN_POINT('',(-0.237465179907044,0.000150546841787672,-5.9006589891905));
#28623=CARTESIAN_POINT('',(-0.23683200269258,0.000108453577955928,-5.8809410108095));
#28624=CARTESIAN_POINT('',(-0.237175,1.98931295048561E-15,-6.1506589891905));
#28625=CARTESIAN_POINT('Ctrl Pts',(-0.237465179907043,0.000150546841787677,
-5.9006589891905));
#28626=CARTESIAN_POINT('Ctrl Pts',(-0.236981875220679,-0.0705666565561128,
-5.89589668375282));
#28627=CARTESIAN_POINT('Ctrl Pts',(-0.165937056871875,-0.220807750888229,
-5.88583918317364));
#28628=CARTESIAN_POINT('Ctrl Pts',(0.0895307381976737,-0.265691300918094,
-5.87048648745296));
#28629=CARTESIAN_POINT('Ctrl Pts',(0.271824417221856,-0.0687432732808278,
-5.85460090202845));
#28630=CARTESIAN_POINT('Ctrl Pts',(0.205068419513521,0.191213573408882,
-5.83871531660395));
#28631=CARTESIAN_POINT('Ctrl Pts',(-0.0495811020651061,0.275961577584089,
-5.82282973117944));
#28632=CARTESIAN_POINT('Ctrl Pts',(-0.216653989164255,0.141732282719992,
-5.81014428870829));
#28633=CARTESIAN_POINT('Ctrl Pts',(-0.237007406444652,0.0314465884532806,
-5.80275404137865));
#28634=CARTESIAN_POINT('Ctrl Pts',(-0.236854733944756,0.000127784916100174,
-5.8006589891905));
#28635=CARTESIAN_POINT('Ctrl Pts',(-0.23683200269258,0.000108453577955931,
-5.8809410108095));
#28636=CARTESIAN_POINT('Ctrl Pts',(-0.23664399711632,-0.0462561242652418,
-5.87784024577449));
#28637=CARTESIAN_POINT('Ctrl Pts',(-0.201079717648982,-0.172066122555996,
-5.86944428559799));
#28638=CARTESIAN_POINT('Ctrl Pts',(0.00331049150882867,-0.28036067894795,
-5.85575313027998));
#28639=CARTESIAN_POINT('Ctrl Pts',(0.237424903254865,-0.149142678857182,
-5.83986754485547));
#28640=CARTESIAN_POINT('Ctrl Pts',(0.254003655790197,0.118728154629452,
-5.82398195943097));
#28641=CARTESIAN_POINT('Ctrl Pts',(0.0378547991123291,0.277814511990848,
-5.80809637400645));
#28642=CARTESIAN_POINT('Ctrl Pts',(-0.188683159783408,0.191603849320789,
-5.79374939113264));
#28643=CARTESIAN_POINT('Ctrl Pts',(-0.236573086892959,0.0558375920822262,
-5.78469760340032));
#28644=CARTESIAN_POINT('Ctrl Pts',(-0.237042509219701,-0.000207466451680186,
-5.7809410108095));
#28645=CARTESIAN_POINT('Ctrl Pts',(-0.103908919352507,0.213201587949045,
-5.99872339910054));
#28646=CARTESIAN_POINT('Ctrl Pts',(-0.174842563682769,0.178630371106822,
-5.99342820395904));
#28647=CARTESIAN_POINT('Ctrl Pts',(-0.278254691691039,0.0337029669877049,
-5.98283781367603));
#28648=CARTESIAN_POINT('Ctrl Pts',(-0.178944516740793,-0.216088258093402,
-5.96695222825153));
#28649=CARTESIAN_POINT('Ctrl Pts',(0.0845713142691825,-0.267244828007485,
-5.95106664282702));
#28650=CARTESIAN_POINT('Ctrl Pts',(0.270472008799548,-0.0738624404218237,
-5.93518105740252));
#28651=CARTESIAN_POINT('Ctrl Pts',(0.208622919271946,0.187359333710957,
-5.91929547197799));
#28652=CARTESIAN_POINT('Ctrl Pts',(-0.0444078770673998,0.276831260195588,
-5.90340988655351));
#28653=CARTESIAN_POINT('Ctrl Pts',(-0.256732964979994,0.112704617543663,
-5.88752430112898));
#28654=CARTESIAN_POINT('Ctrl Pts',(-0.233839555517391,-0.154708578258498,
-5.87163871570449));
#28655=CARTESIAN_POINT('Ctrl Pts',(0.00331049150882867,-0.28036067894795,
-5.85575313027998));
#28656=CARTESIAN_POINT('Ctrl Pts',(0.237424903254865,-0.149142678857182,
-5.83986754485547));
#28657=CARTESIAN_POINT('Ctrl Pts',(0.254003655790197,0.118728154629452,
-5.82398195943097));
#28658=CARTESIAN_POINT('Ctrl Pts',(0.0378547991123291,0.277814511990848,
-5.80809637400645));
#28659=CARTESIAN_POINT('Ctrl Pts',(-0.212977597467589,0.182358424924104,
-5.79221078858196));
#28660=CARTESIAN_POINT('Ctrl Pts',(-0.268672712500568,-0.0801812071883245,
-5.77632520315744));
#28661=CARTESIAN_POINT('Ctrl Pts',(-0.0782004847763744,-0.269255812835206,
-5.76043961773294));
#28662=CARTESIAN_POINT('Ctrl Pts',(0.183921690703183,-0.211629026318924,
-5.74455403230843));
#28663=CARTESIAN_POINT('Ctrl Pts',(0.277528462365728,0.0398996699056295,
-5.72866844688392));
#28664=CARTESIAN_POINT('Ctrl Pts',(0.116854024514864,0.254870874359421,
-5.71278286145941));
#28665=CARTESIAN_POINT('Ctrl Pts',(-0.150886114490242,0.236320565513686,
-5.69689727603491));
#28666=CARTESIAN_POINT('Ctrl Pts',(-0.280379168741369,0.00124515482944624,
-5.6810116906104));
#28667=CARTESIAN_POINT('Ctrl Pts',(-0.15297910832401,-0.23497110554711,
-5.66512610518589));
#28668=CARTESIAN_POINT('Ctrl Pts',(0.114585712811833,-0.255898696670898,
-5.6492405197614));
#28669=CARTESIAN_POINT('Ctrl Pts',(0.277163132557144,-0.0423630307669099,
-5.63335493433687));
#28670=CARTESIAN_POINT('Ctrl Pts',(0.18579408296189,0.209987111717646,-5.61746934891238));
#28671=CARTESIAN_POINT('Ctrl Pts',(-0.0758059453271951,0.269939784166574,
-5.60158376348786));
#28672=CARTESIAN_POINT('Ctrl Pts',(-0.267949938980526,0.0825642695277862,
-5.58569817806337));
#28673=CARTESIAN_POINT('Ctrl Pts',(-0.214588910804631,-0.180459490618597,
-5.56981259263885));
#28674=CARTESIAN_POINT('Ctrl Pts',(0.0353859155308252,-0.278140010402117,
-5.55392700721436));
#28675=CARTESIAN_POINT('Ctrl Pts',(0.252938939516514,-0.120979011722138,
-5.53804142178983));
#28676=CARTESIAN_POINT('Ctrl Pts',(0.238740539723166,0.147027150870172,
-5.52215583636534));
#28677=CARTESIAN_POINT('Ctrl Pts',(0.0057997821945244,0.280321941574533,
-5.50627025094082));
#28678=CARTESIAN_POINT('Ctrl Pts',(-0.232454936814486,0.15677605286409,
-5.49038466551632));
#28679=CARTESIAN_POINT('Ctrl Pts',(-0.257726385342159,-0.110413489662689,
-5.47449908009181));
#28680=CARTESIAN_POINT('Ctrl Pts',(-0.0468599862874815,-0.276438365800292,
-5.45861349466731));
#28681=CARTESIAN_POINT('Ctrl Pts',(0.206941156468481,-0.189180829262909,
-5.4427279092428));
#28682=CARTESIAN_POINT('Ctrl Pts',(0.271135638657325,0.0714107404456813,
-5.42684232381829));
#28683=CARTESIAN_POINT('Ctrl Pts',(0.0869062505835863,0.266573314513364,
-5.41095673839378));
#28684=CARTESIAN_POINT('Ctrl Pts',(-0.176949656626137,0.217492177838692,
-5.39507115296928));
#28685=CARTESIAN_POINT('Ctrl Pts',(-0.278678154992094,-0.0308628309026957,
-5.37918556754476));
#28686=CARTESIAN_POINT('Ctrl Pts',(-0.125072068190222,-0.250940244201183,
-5.36329998212027));
#28687=CARTESIAN_POINT('Ctrl Pts',(0.143129382745379,-0.241097507652099,
-5.34741439669575));
#28688=CARTESIAN_POINT('Ctrl Pts',(0.280190732047764,-0.0103528776514324,
-5.33152881127125));
#28689=CARTESIAN_POINT('Ctrl Pts',(0.160531620654842,0.229877417705736,
-5.31564322584674));
#28690=CARTESIAN_POINT('Ctrl Pts',(-0.10621212594168,0.259486054931813,
-5.29975764042223));
#28691=CARTESIAN_POINT('Ctrl Pts',(-0.27564064121739,0.0513445743033626,
-5.28387205499773));
#28692=CARTESIAN_POINT('Ctrl Pts',(-0.192517646732188,-0.203840585011494,
-5.26798646957322));
#28693=CARTESIAN_POINT('Ctrl Pts',(0.0669966887508262,-0.272259934800463,
-5.25210088414871));
#28694=CARTESIAN_POINT('Ctrl Pts',(0.265126335755849,-0.0912252952300192,
-5.23621529872421));
#28695=CARTESIAN_POINT('Ctrl Pts',(0.220338044111505,0.173393121888511,
-5.2203297132997));
#28696=CARTESIAN_POINT('Ctrl Pts',(-0.0263316009223782,0.279142750566788,
-5.2044441278752));
#28697=CARTESIAN_POINT('Ctrl Pts',(-0.248875320483161,0.129132115507845,
-5.18855854245069));
#28698=CARTESIAN_POINT('Ctrl Pts',(-0.24339084488138,-0.139193839766909,
-5.17267295702618));
#28699=CARTESIAN_POINT('Ctrl Pts',(-0.0149032407667099,-0.279985574299422,
-5.15678737160167));
#28700=CARTESIAN_POINT('Ctrl Pts',(0.22723922911572,-0.164244820776854,
-5.14090178617716));
#28701=CARTESIAN_POINT('Ctrl Pts',(0.261177240698333,0.101982730608336,
-5.12501620075266));
#28702=CARTESIAN_POINT('Ctrl Pts',(0.0558156114071165,0.274770169276757,
-5.10913061532815));
#28703=CARTESIAN_POINT('Ctrl Pts',(-0.200686215740403,0.195803654748638,
-5.09324502990364));
#28704=CARTESIAN_POINT('Ctrl Pts',(-0.273312375825205,-0.0625649552218312,
-5.07735944447914));
#28705=CARTESIAN_POINT('Ctrl Pts',(-0.0955202636039318,-0.26360938458667,
-5.06147385905463));
#28706=CARTESIAN_POINT('Ctrl Pts',(0.169790825062137,-0.223125758544025,
-5.04558827363013));
#28707=CARTESIAN_POINT('Ctrl Pts',(0.279533674503372,0.0217934214792116,
-5.02970268820562));
#28708=CARTESIAN_POINT('Ctrl Pts',(0.133158082146451,0.246744713337908,
-5.01381710278111));
#28709=CARTESIAN_POINT('Ctrl Pts',(-0.135221560608942,0.245619946151793,
-4.99793151735661));
#28710=CARTESIAN_POINT('Ctrl Pts',(-0.279706522474076,0.0194496706035552,
-4.9820459319321));
#28711=CARTESIAN_POINT('Ctrl Pts',(-0.167914673239027,-0.224541067317669,
-4.96616034650759));
#28712=CARTESIAN_POINT('Ctrl Pts',(0.0977264198891994,-0.262799496302347,
-4.95027476108308));
#28713=CARTESIAN_POINT('Ctrl Pts',(0.273827179714107,-0.0602719175980483,
-4.93438917565858));
#28714=CARTESIAN_POINT('Ctrl Pts',(0.199037986065754,0.197478881159522,
-4.91850359023406));
#28715=CARTESIAN_POINT('Ctrl Pts',(-0.0581167094863374,0.274292683970259,
-4.90261800480957));
#28716=CARTESIAN_POINT('Ctrl Pts',(-0.262022861361101,0.0997900221729051,
-4.88673241938505));
#28717=CARTESIAN_POINT('Ctrl Pts',(-0.225854585399838,-0.166143716868844,
-4.87084683396055));
#28718=CARTESIAN_POINT('Ctrl Pts',(0.0172494902941208,-0.279850823628805,
-4.85496124853605));
#28719=CARTESIAN_POINT('Ctrl Pts',(0.244548985077421,-0.137148905568842,
-4.83907566311153));
#28720=CARTESIAN_POINT('Ctrl Pts',(0.247784223156673,0.131213593639424,
-4.82319007768704));
#28721=CARTESIAN_POINT('Ctrl Pts',(0.0239909672635905,0.279353650219367,
-4.80730449226251));
#28722=CARTESIAN_POINT('Ctrl Pts',(-0.221783644413183,0.171540209490179,
-4.79141890683803));
#28723=CARTESIAN_POINT('Ctrl Pts',(-0.264352393596509,-0.093444317114117,
-4.77553332141351));
#28724=CARTESIAN_POINT('Ctrl Pts',(-0.0647123167632992,-0.272811921404205,
-4.759647735989));
#28725=CARTESIAN_POINT('Ctrl Pts',(0.194219427751849,-0.202219787075528,
-4.7437621505645));
#28726=CARTESIAN_POINT('Ctrl Pts',(0.275200600511704,0.0536531255298783,
-4.72787656513998));
#28727=CARTESIAN_POINT('Ctrl Pts',(0.104033444057923,0.260367184795962,
-4.71199097971549));
#28728=CARTESIAN_POINT('Ctrl Pts',(-0.162452759857131,0.228523804484191,
-4.69610539429097));
#28729=CARTESIAN_POINT('Ctrl Pts',(-0.280094114240769,-0.0127010066060424,
-4.68021980886647));
#28730=CARTESIAN_POINT('Ctrl Pts',(-0.141103532512842,-0.242288715200532,
-4.66433422344196));
#28731=CARTESIAN_POINT('Ctrl Pts',(0.127170996645068,-0.249883104697832,
-4.64844863801745));
#28732=CARTESIAN_POINT('Ctrl Pts',(0.278927050665701,-0.0285259322031912,
-4.63256305259295));
#28733=CARTESIAN_POINT('Ctrl Pts',(0.175120472675097,0.218967688144114,
-4.61667746716844));
#28734=CARTESIAN_POINT('Ctrl Pts',(-0.0891375524199996,0.265835522738591,
-4.60079188174394));
#28735=CARTESIAN_POINT('Ctrl Pts',(-0.271724662295054,0.0691356369882154,
-4.58490629631942));
#28736=CARTESIAN_POINT('Ctrl Pts',(-0.205348218033809,-0.190908715755637,
-4.56902071089492));
#28737=CARTESIAN_POINT('Ctrl Pts',(0.0491753813860615,-0.276035885831286,
-4.55313512547041));
#28738=CARTESIAN_POINT('Ctrl Pts',(0.258642791859093,-0.108249409330772,
-4.53724954004591));
#28739=CARTESIAN_POINT('Ctrl Pts',(0.231132711334074,0.158718928148119,
-4.5213639546214));
#28740=CARTESIAN_POINT('Ctrl Pts',(-0.00814917085540682,0.280263482129757,
-4.50547836919689));
#28741=CARTESIAN_POINT('Ctrl Pts',(-0.239964500239963,0.145020919269299,
-4.48959278377239));
#28742=CARTESIAN_POINT('Ctrl Pts',(-0.251916036836325,-0.123094836552177,
-4.47370719834787));
#28743=CARTESIAN_POINT('Ctrl Pts',(-0.0330533685498055,-0.278426836401662,
-4.45782161292337));
#28744=CARTESIAN_POINT('Ctrl Pts',(0.216093941700501,-0.178654517887089,
-4.44193602749886));
#28745=CARTESIAN_POINT('Ctrl Pts',(0.26724849229964,0.0848072624525569,
-4.42605044207435));
#28746=CARTESIAN_POINT('Ctrl Pts',(0.0735407108656338,0.270565689337182,
-4.41016485664985));
#28747=CARTESIAN_POINT('Ctrl Pts',(-0.187547618937357,0.208422453281923,
-4.39427927122535));
#28748=CARTESIAN_POINT('Ctrl Pts',(-0.276798319479655,-0.0446846588256681,
-4.37839368580083));
#28749=CARTESIAN_POINT('Ctrl Pts',(-0.112436805309618,-0.256850137654031,
-4.36250810037634));
#28750=CARTESIAN_POINT('Ctrl Pts',(0.154943207178462,-0.23368061740414,
-4.34662251495182));
#28751=CARTESIAN_POINT('Ctrl Pts',(0.280358882596026,0.00359518436732559,
-4.33073692952732));
#28752=CARTESIAN_POINT('Ctrl Pts',(0.14890003195752,0.237576953604884,-4.3148513441028));
#28753=CARTESIAN_POINT('Ctrl Pts',(-0.11898618914506,0.253882483038636,
-4.29896575867831));
#28754=CARTESIAN_POINT('Ctrl Pts',(-0.27785313944431,0.0375720814178366,
-4.28308017325379));
#28755=CARTESIAN_POINT('Ctrl Pts',(-0.182141412417354,-0.21316316352442,
-4.26719458782929));
#28756=CARTESIAN_POINT('Ctrl Pts',(0.0804545900663122,-0.268590929367298,
-4.25130900240478));
#28757=CARTESIAN_POINT('Ctrl Pts',(0.269335308407912,-0.0779263758039853,
-4.23542341698027));
#28758=CARTESIAN_POINT('Ctrl Pts',(0.211441681464576,0.184137024361096,
-4.21953783155577));
#28759=CARTESIAN_POINT('Ctrl Pts',(-0.0401821430447466,0.277487700234545,
-4.20365224613126));
#28760=CARTESIAN_POINT('Ctrl Pts',(-0.254989695299907,0.11659452685267,
-4.18776666070675));
#28761=CARTESIAN_POINT('Ctrl Pts',(-0.236166850248402,-0.151126593440284,
-4.17188107528225));
#28762=CARTESIAN_POINT('Ctrl Pts',(-0.000959750965527487,-0.280380290461363,
-4.15599548985773));
#28763=CARTESIAN_POINT('Ctrl Pts',(0.235126705419149,-0.152739846798193,
-4.14010990443324));
#28764=CARTESIAN_POINT('Ctrl Pts',(0.255781924318054,0.114846138782203,
-4.12422431900872));
#28765=CARTESIAN_POINT('Ctrl Pts',(0.0420808782244523,0.277206111204153,
-4.10833873358422));
#28766=CARTESIAN_POINT('Ctrl Pts',(-0.210176127110702,0.185580236001482,
-4.09245314815971));
#28767=CARTESIAN_POINT('Ctrl Pts',(-0.269862479642514,-0.076080684023625,
-4.07656756273521));
#28768=CARTESIAN_POINT('Ctrl Pts',(-0.0822914743374018,-0.268033844229383,
-4.0606819773107));
#28769=CARTESIAN_POINT('Ctrl Pts',(0.180677832160775,-0.214405105746405,
-4.04479639188619));
#28770=CARTESIAN_POINT('Ctrl Pts',(0.278103846141642,0.0356690223564828,
-4.02891080646169));
#28771=CARTESIAN_POINT('Ctrl Pts',(0.1207214766735,0.253061955797574,-4.01302522103717));
#28772=CARTESIAN_POINT('Ctrl Pts',(-0.14727009426389,0.238590753715125,
-3.99713963561268));
#28773=CARTESIAN_POINT('Ctrl Pts',(-0.280327699987403,0.00551443296643659,
-3.98125405018816));
#28774=CARTESIAN_POINT('Ctrl Pts',(-0.156539350554289,-0.232614402289902,
-3.96536846476366));
#28775=CARTESIAN_POINT('Ctrl Pts',(0.110675778439994,-0.257613859497429,
-3.94948287933915));
#28776=CARTESIAN_POINT('Ctrl Pts',(0.276485921807596,-0.0465785687612247,
-3.93359729391465));
#28777=CARTESIAN_POINT('Ctrl Pts',(0.188970082294562,0.207133620332956,
-3.91771170849014));
#28778=CARTESIAN_POINT('Ctrl Pts',(-0.0716867010729343,0.271062808441053,
-3.90182612306563));
#28779=CARTESIAN_POINT('Ctrl Pts',(-0.266661635680487,0.0866348526764077,
-3.88594053764112));
#28780=CARTESIAN_POINT('Ctrl Pts',(-0.217311952916841,-0.17717095191123,
-3.87005495221662));
#28781=CARTESIAN_POINT('Ctrl Pts',(0.0311465050672407,-0.278646601116737,
-3.85416936679211));
#28782=CARTESIAN_POINT('Ctrl Pts',(0.251067394679135,-0.124816552964098,
-3.83828378136761));
#28783=CARTESIAN_POINT('Ctrl Pts',(0.240951752322899,0.143374703072453,
-3.82239819594309));
#28784=CARTESIAN_POINT('Ctrl Pts',(0.0100675354129855,0.280201172186297,
-3.80651261051859));
#28785=CARTESIAN_POINT('Ctrl Pts',(-0.230040467341084,0.160297449368488,
-3.79062702509408));
#28786=CARTESIAN_POINT('Ctrl Pts',(-0.25937826877251,-0.106476032726035,
-3.77474143966958));
#28787=CARTESIAN_POINT('Ctrl Pts',(-0.0510630698782088,-0.275693101540268,
-3.75885585424507));
#28788=CARTESIAN_POINT('Ctrl Pts',(0.204034714334676,-0.192309399147709,
-3.74297026882056));
#28789=CARTESIAN_POINT('Ctrl Pts',(0.272194945935335,0.0672725301932114,
-3.72708468339606));
#28790=CARTESIAN_POINT('Ctrl Pts',(0.0909488961210605,0.265221500669614,
-3.71119909797155));
#28791=CARTESIAN_POINT('Ctrl Pts',(-0.173604808053276,0.220156709613621,
-3.69531351254704));
#28792=CARTESIAN_POINT('Ctrl Pts',(-0.279139983968874,-0.0266066105323439,
-3.67942792712253));
#28793=CARTESIAN_POINT('Ctrl Pts',(-0.12883195646667,-0.249024285245638,
-3.66354234169802));
#28794=CARTESIAN_POINT('Ctrl Pts',(0.139350939164339,-0.243214763219636,
-3.64765675627352));
#28795=CARTESIAN_POINT('Ctrl Pts',(0.280177793680504,-0.0146860234836151,
-3.63177117084901));
#28796=CARTESIAN_POINT('Ctrl Pts',(0.163650290907218,0.227552512000709,
-3.61588558542451));
#28797=CARTESIAN_POINT('Ctrl Pts',(-0.0130164034045845,0.24961831823673,
-3.6052951951415));
#28798=CARTESIAN_POINT('Ctrl Pts',(-0.0864920085589077,0.220841828194855,
-3.6));
#28799=CARTESIAN_POINT('Ctrl Pts',(-0.112236674703446,0.230288577939269,
-5.98774893273369));
#28800=CARTESIAN_POINT('Ctrl Pts',(-0.188855278898692,0.192946659237761,
-5.98245373759219));
#28801=CARTESIAN_POINT('Ctrl Pts',(-0.300555347035098,0.0364040831712175,
-5.97186334730918));
#28802=CARTESIAN_POINT('Ctrl Pts',(-0.193285981998013,-0.233406599568089,
-5.95597776188468));
#28803=CARTESIAN_POINT('Ctrl Pts',(0.0913492619115004,-0.288663100474548,
-5.94009217646017));
#28804=CARTESIAN_POINT('Ctrl Pts',(0.292148922895039,-0.0797821279451774,
-5.92420659103567));
#28805=CARTESIAN_POINT('Ctrl Pts',(0.225342952962235,0.202375202450449,
-5.90832100561115));
#28806=CARTESIAN_POINT('Ctrl Pts',(-0.0479669356946704,0.299017834964786,
-5.89243542018666));
#28807=CARTESIAN_POINT('Ctrl Pts',(-0.277308766712869,0.121737302010726,
-5.87654983476215));
#28808=CARTESIAN_POINT('Ctrl Pts',(-0.252580570454855,-0.167107660054908,
-5.86066424933764));
#28809=CARTESIAN_POINT('Ctrl Pts',(0.00357581005461561,-0.302830118134215,
-5.84477866391314));
#28810=CARTESIAN_POINT('Ctrl Pts',(0.256453265024457,-0.161095682984698,
-5.82889307848862));
#28811=CARTESIAN_POINT('Ctrl Pts',(0.274360717694467,0.128243594027568,
-5.81300749306412));
#28812=CARTESIAN_POINT('Ctrl Pts',(0.040888662882935,0.300079889238701,
-5.79712190763961));
#28813=CARTESIAN_POINT('Ctrl Pts',(-0.230046635794548,0.196973497031616,
-5.7812363222151));
#28814=CARTESIAN_POINT('Ctrl Pts',(-0.290205422426916,-0.0866073107544878,
-5.7653507367906));
#28815=CARTESIAN_POINT('Ctrl Pts',(-0.0844678438212043,-0.290835255197635,
-5.74946515136609));
#28816=CARTESIAN_POINT('Ctrl Pts',(0.198662050370586,-0.22858998373551,
-5.73357956594158));
#28817=CARTESIAN_POINT('Ctrl Pts',(0.299770914235171,0.0430974193541643,
-5.71769398051708));
#28818=CARTESIAN_POINT('Ctrl Pts',(0.126219262205683,0.275297439287351,
-5.70180839509257));
#28819=CARTESIAN_POINT('Ctrl Pts',(-0.162978845847265,0.255260420400609,
-5.68592280966807));
#28820=CARTESIAN_POINT('Ctrl Pts',(-0.30285008978768,0.0013449474637867,
-5.67003722424355));
#28821=CARTESIAN_POINT('Ctrl Pts',(-0.165239582168466,-0.253802808289563,
-5.65415163881905));
#28822=CARTESIAN_POINT('Ctrl Pts',(0.123769157206752,-0.276407636170786,
-5.63826605339454));
#28823=CARTESIAN_POINT('Ctrl Pts',(0.299376305156942,-0.0457582056792222,
-5.62238046797004));
#28824=CARTESIAN_POINT('Ctrl Pts',(0.200684505056548,0.226816478283401,
-5.60649488254552));
#28825=CARTESIAN_POINT('Ctrl Pts',(-0.0818813945837688,0.291574043246857,
-5.59060929712102));
#28826=CARTESIAN_POINT('Ctrl Pts',(-0.28942472239694,0.0891813630520081,
-5.57472371169651));
#28827=CARTESIAN_POINT('Ctrl Pts',(-0.231787087451459,-0.194922373092896,
-5.55883812627201));
#28828=CARTESIAN_POINT('Ctrl Pts',(0.0382219112205695,-0.300431474641856,
-5.5429525408475));
#28829=CARTESIAN_POINT('Ctrl Pts',(0.2732106699911,-0.130674845520605,-5.52706695542299));
#28830=CARTESIAN_POINT('Ctrl Pts',(0.257874342861093,0.158810606515963,
-5.51118136999849));
#28831=CARTESIAN_POINT('Ctrl Pts',(0.00626460434363062,0.302788276163322,
-5.49529578457398));
#28832=CARTESIAN_POINT('Ctrl Pts',(-0.251084981819014,0.169340831915528,
-5.47941019914947));
#28833=CARTESIAN_POINT('Ctrl Pts',(-0.278381804511037,-0.119262552236759,
-5.46352461372497));
#28834=CARTESIAN_POINT('Ctrl Pts',(-0.0506155686184515,-0.298593452142671,
-5.44763902830046));
#28835=CARTESIAN_POINT('Ctrl Pts',(0.223526405683357,-0.204342681325335,
-5.43175344287595));
#28836=CARTESIAN_POINT('Ctrl Pts',(0.292865739208162,0.0771339370640931,
-5.41586785745144));
#28837=CARTESIAN_POINT('Ctrl Pts',(0.0938713311352587,0.287937768692942,
-5.39998227202694));
#28838=CARTESIAN_POINT('Ctrl Pts',(-0.191131244299241,0.234923036123716,
-5.38409668660243));
#28839=CARTESIAN_POINT('Ctrl Pts',(-0.301012748700572,-0.0333363250627414,
-5.36821110117793));
#28840=CARTESIAN_POINT('Ctrl Pts',(-0.135095939014926,-0.271051789720416,
-5.35232551575341));
#28841=CARTESIAN_POINT('Ctrl Pts',(0.15460045270224,-0.260420209417829,
-5.33643993032891));
#28842=CARTESIAN_POINT('Ctrl Pts',(0.302646550880586,-0.011182606540892,
-5.3205543449044));
#28843=CARTESIAN_POINT('Ctrl Pts',(0.173397388783639,0.248300888061197,
-5.3046687594799));
#28844=CARTESIAN_POINT('Ctrl Pts',(-0.114724471230777,0.280282502396747,
-5.28878317405539));
#28845=CARTESIAN_POINT('Ctrl Pts',(-0.29773179411493,0.0554595728623016,
-5.27289758863089));
#28846=CARTESIAN_POINT('Ctrl Pts',(-0.207946927228169,-0.220177339672652,
-5.25701200320637));
#28847=CARTESIAN_POINT('Ctrl Pts',(0.0723661222577529,-0.294080141795293,
-5.24112641778187));
#28848=CARTESIAN_POINT('Ctrl Pts',(0.286374822170912,-0.0985365245761303,
-5.22524083235736));
#28849=CARTESIAN_POINT('Ctrl Pts',(0.237996983664519,0.187289671940431,
-5.20935524693285));
#28850=CARTESIAN_POINT('Ctrl Pts',(-0.0284419407454325,0.301514579175862,
-5.19346966150835));
#28851=CARTESIAN_POINT('Ctrl Pts',(-0.268821373187637,0.13948137784836,
-5.17758407608384));
#28852=CARTESIAN_POINT('Ctrl Pts',(-0.262897345607792,-0.150349496578276,
-5.16169849065933));
#28853=CARTESIAN_POINT('Ctrl Pts',(-0.0160976574136605,-0.302424950813844,
-5.14581290523482));
#28854=CARTESIAN_POINT('Ctrl Pts',(0.245451262481131,-0.177408182436388,
-5.12992731981032));
#28855=CARTESIAN_POINT('Ctrl Pts',(0.282109227839787,0.110156112025631,
-5.11404173438581));
#28856=CARTESIAN_POINT('Ctrl Pts',(0.0602889401594312,0.296791558409967,
-5.09815614896131));
#28857=CARTESIAN_POINT('Ctrl Pts',(-0.21677016423497,0.211496291566797,
-5.0822705635368));
#28858=CARTESIAN_POINT('Ctrl Pts',(-0.295216930452845,-0.0675792085109285,
-5.06638497811229));
#28859=CARTESIAN_POINT('Ctrl Pts',(-0.103175712157411,-0.284736295315112,
-5.05049939268779));
#28860=CARTESIAN_POINT('Ctrl Pts',(0.183398669901276,-0.241008118799775,
-5.03461380726328));
#28861=CARTESIAN_POINT('Ctrl Pts',(0.301936833617324,0.0235400500022461,
-5.01872822183878));
#28862=CARTESIAN_POINT('Ctrl Pts',(0.143830004614954,0.266520009045148,
-5.00284263641426));
#28863=CARTESIAN_POINT('Ctrl Pts',(-0.146058860062545,0.265305097663414,
-4.98695705098977));
#28864=CARTESIAN_POINT('Ctrl Pts',(-0.302123534447069,0.0210084597763427,
-4.97107146556525));
#28865=CARTESIAN_POINT('Ctrl Pts',(-0.181372154341526,-0.242536857154696,
-4.95518588014075));
#28866=CARTESIAN_POINT('Ctrl Pts',(0.105558680307571,-0.283861498729024,
-4.93930029471624));
#28867=CARTESIAN_POINT('Ctrl Pts',(0.295772993175611,-0.0651023959382731,
-4.92341470929173));
#28868=CARTESIAN_POINT('Ctrl Pts',(0.214989837589453,0.213305778595482,
-4.90752912386722));
#28869=CARTESIAN_POINT('Ctrl Pts',(-0.0627744591907873,0.296275805158416,
-4.89164353844272));
#28870=CARTESIAN_POINT('Ctrl Pts',(-0.283022620567196,0.107787669499998,
-4.87575795301821));
#28871=CARTESIAN_POINT('Ctrl Pts',(-0.243955646827653,-0.179459265098978,
-4.8598723675937));
#28872=CARTESIAN_POINT('Ctrl Pts',(0.0186319465451625,-0.302279400583139,
-4.8439867821692));
#28873=CARTESIAN_POINT('Ctrl Pts',(0.264148304671307,-0.148140671620721,
-4.82810119674469));
#28874=CARTESIAN_POINT('Ctrl Pts',(0.267642830128331,0.141729675544189,
-4.81221561132019));
#28875=CARTESIAN_POINT('Ctrl Pts',(0.025913717564994,0.301742381330375,
-4.79633002589567));
#28876=CARTESIAN_POINT('Ctrl Pts',(-0.239558441254702,0.185288258323568,
-4.78044444047117));
#28877=CARTESIAN_POINT('Ctrl Pts',(-0.285538852603348,-0.100933389435444,
-4.76455885504666));
#28878=CARTESIAN_POINT('Ctrl Pts',(-0.069898669826687,-0.294676367232637,
-4.74867326962215));
#28879=CARTESIAN_POINT('Ctrl Pts',(0.209785097078365,-0.218426643275917,
-4.73278768419765));
#28880=CARTESIAN_POINT('Ctrl Pts',(0.297256486452718,0.0579531423716499,
-4.71690209877314));
#28881=CARTESIAN_POINT('Ctrl Pts',(0.112371179411428,0.281234250201941,
-4.70101651334864));
#28882=CARTESIAN_POINT('Ctrl Pts',(-0.175472497225253,0.246838789833562,
-4.68513092792412));
#28883=CARTESIAN_POINT('Ctrl Pts',(-0.302542189662687,-0.0137189257258342,
-4.66924534249962));
#28884=CARTESIAN_POINT('Ctrl Pts',(-0.152412241190043,-0.261706886008741,
-4.65335975707511));
#28885=CARTESIAN_POINT('Ctrl Pts',(0.137363085585984,-0.269909926025816,
-4.63747417165061));
#28886=CARTESIAN_POINT('Ctrl Pts',(0.301281592058078,-0.0308121361789995,
-4.6215885862261));
#28887=CARTESIAN_POINT('Ctrl Pts',(0.189155460840372,0.236516800847699,
-4.60570300080159));
#28888=CARTESIAN_POINT('Ctrl Pts',(-0.0962814601207137,0.287140846773822,
-4.58981741537709));
#28889=CARTESIAN_POINT('Ctrl Pts',(-0.293501970003673,0.0746764959872007,
-4.57393182995257));
#28890=CARTESIAN_POINT('Ctrl Pts',(-0.221805801580948,-0.206209048865458,
-4.55804624452808));
#28891=CARTESIAN_POINT('Ctrl Pts',(0.0531165305003444,-0.298158715513348,
-4.54216065910356));
#28892=CARTESIAN_POINT('Ctrl Pts',(0.279371656207873,-0.116925032207111,
-4.52627507367906));
#28893=CARTESIAN_POINT('Ctrl Pts',(0.249656786895474,0.171439418471925,
-4.51038948825455));
#28894=CARTESIAN_POINT('Ctrl Pts',(-0.00880228419370061,0.302725131500404,
-4.49450390283004));
#28895=CARTESIAN_POINT('Ctrl Pts',(-0.259196397399141,0.156643585965945,
-4.47861831740554));
#28896=CARTESIAN_POINT('Ctrl Pts',(-0.272105787021618,-0.132960242622783,
-4.46273273198103));
#28897=CARTESIAN_POINT('Ctrl Pts',(-0.035702422822744,-0.300741288242153,
-4.44684714655653));
#28898=CARTESIAN_POINT('Ctrl Pts',(0.233412738686511,-0.192972741255926,
-4.43096156113201));
#28899=CARTESIAN_POINT('Ctrl Pts',(0.288667058440516,0.0916041201052846,
-4.41507597570751));
#28900=CARTESIAN_POINT('Ctrl Pts',(0.0794346134510843,0.292250111436831,
-4.399190390283));
#28901=CARTESIAN_POINT('Ctrl Pts',(-0.202578577751036,0.225126420673654,
-4.3833048048585));
#28902=CARTESIAN_POINT('Ctrl Pts',(-0.298982254223097,-0.0482659000603877,
-4.36741921943399));
#28903=CARTESIAN_POINT('Ctrl Pts',(-0.121448026029594,-0.277435330162687,
-4.35153363400948));
#28904=CARTESIAN_POINT('Ctrl Pts',(0.167361093253233,-0.252408894284742,
-4.33564804858498));
#28905=CARTESIAN_POINT('Ctrl Pts',(0.302828177814098,0.00388331955378666,
-4.31976246316047));
#28906=CARTESIAN_POINT('Ctrl Pts',(0.16083358920762,0.256617501413209,-4.30387687773596));
#28907=CARTESIAN_POINT('Ctrl Pts',(-0.128522308657371,0.274229833581875,
-4.28799129231146));
#28908=CARTESIAN_POINT('Ctrl Pts',(-0.30012161248013,0.0405832868468127,
-4.27210570688694));
#28909=CARTESIAN_POINT('Ctrl Pts',(-0.196739092109704,-0.230247073998374,
-4.25622012146245));
#28910=CARTESIAN_POINT('Ctrl Pts',(0.0869026038374818,-0.290117084804099,
-4.24033453603793));
#28911=CARTESIAN_POINT('Ctrl Pts',(0.290921121923897,-0.0841717664511477,
-4.22444895061343));
#28912=CARTESIAN_POINT('Ctrl Pts',(0.228387624172868,0.198894641892724,
-4.20856336518892));
#28913=CARTESIAN_POINT('Ctrl Pts',(-0.0434025312350796,0.299726885232788,
-4.19267777976441));
#28914=CARTESIAN_POINT('Ctrl Pts',(-0.275425783103537,0.125938967165763,
-4.17679219433991));
#28915=CARTESIAN_POINT('Ctrl Pts',(-0.255094385662357,-0.163238597924922,
-4.1609066089154));
#28916=CARTESIAN_POINT('Ctrl Pts',(-0.00103666997583505,-0.302851301407654,
-4.1450210234909));
#28917=CARTESIAN_POINT('Ctrl Pts',(0.253970878675925,-0.164981145085206,
-4.12913543806639));
#28918=CARTESIAN_POINT('Ctrl Pts',(0.276281505125808,0.124050454953884,
-4.11324985264188));
#28919=CARTESIAN_POINT('Ctrl Pts',(0.0454534400891082,0.299422728317279,
-4.09736426721737));
#28920=CARTESIAN_POINT('Ctrl Pts',(-0.227020642269675,0.200453519382929,
-4.08147868179287));
#28921=CARTESIAN_POINT('Ctrl Pts',(-0.291490543170309,-0.0821781521469477,
-4.06559309636836));
#28922=CARTESIAN_POINT('Ctrl Pts',(-0.0888867047566989,-0.289515352211788,
-4.04970751094385));
#28923=CARTESIAN_POINT('Ctrl Pts',(0.19515821356546,-0.231588551381047,
-4.03382192551934));
#28924=CARTESIAN_POINT('Ctrl Pts',(0.300392412005423,0.0385277075746812,
-4.01793634009484));
#28925=CARTESIAN_POINT('Ctrl Pts',(0.130396670387433,0.273343545382419,
-4.00205075467033));
#28926=CARTESIAN_POINT('Ctrl Pts',(-0.159073020549541,0.257712552289462,
-3.98616516924583));
#28927=CARTESIAN_POINT('Ctrl Pts',(-0.302794496082807,0.00595638587028517,
-3.97027958382131));
#28928=CARTESIAN_POINT('Ctrl Pts',(-0.169085159156036,-0.251257227616604,
-3.95439399839681));
#28929=CARTESIAN_POINT('Ctrl Pts',(0.119545862085038,-0.278260260309545,
-3.9385084129723));
#28930=CARTESIAN_POINT('Ctrl Pts',(0.298644819514743,-0.0503115969522353,
-3.9226228275478));
#28931=CARTESIAN_POINT('Ctrl Pts',(0.204115044091895,0.223734294517963,
-3.90673724212329));
#28932=CARTESIAN_POINT('Ctrl Pts',(-0.0774320144894472,0.292787072031722,
-3.89085165669878));
#28933=CARTESIAN_POINT('Ctrl Pts',(-0.288033168338763,0.0935781821080819,
-3.87496607127428));
#28934=CARTESIAN_POINT('Ctrl Pts',(-0.234728367118847,-0.191370275241736,
-3.85908048584977));
#28935=CARTESIAN_POINT('Ctrl Pts',(0.0336427342249789,-0.300978665947462,
-3.84319490042527));
#28936=CARTESIAN_POINT('Ctrl Pts',(0.271189130642844,-0.134819945582456,
-3.82730931500076));
#28937=CARTESIAN_POINT('Ctrl Pts',(0.260262772562825,0.154865434167926,
-3.81142372957625));
#28938=CARTESIAN_POINT('Ctrl Pts',(0.0108743956173709,0.302657827741511,
-3.79553814415174));
#28939=CARTESIAN_POINT('Ctrl Pts',(-0.248477005270357,0.173144449895859,
-3.77965255872723));
#28940=CARTESIAN_POINT('Ctrl Pts',(-0.280166077741629,-0.115009528760893,
-3.76376697330273));
#28941=CARTESIAN_POINT('Ctrl Pts',(-0.0551555073326973,-0.297788458857768,
-3.74788138787822));
#28942=CARTESIAN_POINT('Ctrl Pts',(0.220387027443752,-0.207721989691116,
-3.73199580245372));
#28943=CARTESIAN_POINT('Ctrl Pts',(0.294009944413199,0.0726640709461968,
-3.71611021702921));
#28944=CARTESIAN_POINT('Ctrl Pts',(0.0982379735270597,0.286477614053803,
-3.7002246316047));
#28945=CARTESIAN_POINT('Ctrl Pts',(-0.18751832364196,0.237801116156914,
-3.68433904618019));
#28946=CARTESIAN_POINT('Ctrl Pts',(-0.301511590849623,-0.0287389909344478,
-3.66845346075569));
#28947=CARTESIAN_POINT('Ctrl Pts',(-0.139157162633019,-0.268982276695176,
-3.65256787533117));
#28948=CARTESIAN_POINT('Ctrl Pts',(0.15051918666913,-0.262707151923616,
-3.63668228990668));
#28949=CARTESIAN_POINT('Ctrl Pts',(0.302632575570994,-0.0158630313036537,
-3.62079670448216));
#28950=CARTESIAN_POINT('Ctrl Pts',(0.176766004113337,0.245789653347592,
-3.60491111905766));
#28951=CARTESIAN_POINT('Ctrl Pts',(-0.0140595999249409,0.269623918317471,
-3.59432072877466));
#28952=CARTESIAN_POINT('Ctrl Pts',(-0.0934238897831399,0.238541143402067,
-3.58902553363315));
#28953=CARTESIAN_POINT('Ctrl Pts',(-0.120564430054385,0.247375567929493,
-5.97677446636685));
#28954=CARTESIAN_POINT('Ctrl Pts',(-0.202867994114616,0.2072629473687,-5.97147927122534));
#28955=CARTESIAN_POINT('Ctrl Pts',(-0.322856002379157,0.0391051993547299,
-5.96088888094234));
#28956=CARTESIAN_POINT('Ctrl Pts',(-0.207627447255233,-0.250724941042775,
-5.94500329551783));
#28957=CARTESIAN_POINT('Ctrl Pts',(0.0981272095538185,-0.31008137294161,
-5.92911771009333));
#28958=CARTESIAN_POINT('Ctrl Pts',(0.31382583699053,-0.0857018154685313,
-5.91323212466882));
#28959=CARTESIAN_POINT('Ctrl Pts',(0.242062986652523,0.217391071189942,
-5.89734653924431));
#28960=CARTESIAN_POINT('Ctrl Pts',(-0.0515259943219408,0.321204409733984,
-5.88146095381981));
#28961=CARTESIAN_POINT('Ctrl Pts',(-0.297884568445745,0.13076998647779,
-5.8655753683953));
#28962=CARTESIAN_POINT('Ctrl Pts',(-0.271321585392319,-0.179506741851318,
-5.84968978297079));
#28963=CARTESIAN_POINT('Ctrl Pts',(0.0038411286004027,-0.32529955732048,
-5.83380419754628));
#28964=CARTESIAN_POINT('Ctrl Pts',(0.275481626794049,-0.173048687112214,
-5.81791861212178));
#28965=CARTESIAN_POINT('Ctrl Pts',(0.294717779598738,0.137759033425684,
-5.80203302669727));
#28966=CARTESIAN_POINT('Ctrl Pts',(0.0439225266535408,0.322345266486553,
-5.78614744127277));
#28967=CARTESIAN_POINT('Ctrl Pts',(-0.247115674121507,0.211588569139127,
-5.77026185584825));
#28968=CARTESIAN_POINT('Ctrl Pts',(-0.311738132353264,-0.093033414320651,
-5.75437627042376));
#28969=CARTESIAN_POINT('Ctrl Pts',(-0.0907352028660341,-0.312414697560065,
-5.73849068499924));
#28970=CARTESIAN_POINT('Ctrl Pts',(0.21340241003799,-0.245550941152097,
-5.72260509957474));
#28971=CARTESIAN_POINT('Ctrl Pts',(0.322013366104615,0.046295168802699,
-5.70671951415023));
#28972=CARTESIAN_POINT('Ctrl Pts',(0.135584499896502,0.295724004215282,
-5.69083392872572));
#28973=CARTESIAN_POINT('Ctrl Pts',(-0.175071577204289,0.274200275287532,
-5.67494834330122));
#28974=CARTESIAN_POINT('Ctrl Pts',(-0.325321010833992,0.00144474009812678,
-5.6590627578767));
#28975=CARTESIAN_POINT('Ctrl Pts',(-0.177500056012922,-0.272634511032016,
-5.64317717245221));
#28976=CARTESIAN_POINT('Ctrl Pts',(0.132952601601671,-0.296916575670675,
-5.62729158702769));
#28977=CARTESIAN_POINT('Ctrl Pts',(0.321589477756739,-0.049153380591534,
-5.61140600160319));
#28978=CARTESIAN_POINT('Ctrl Pts',(0.215574927151207,0.243645844849156,
-5.59552041617868));
#28979=CARTESIAN_POINT('Ctrl Pts',(-0.0879568438403424,0.313208302327141,
-5.57963483075418));
#28980=CARTESIAN_POINT('Ctrl Pts',(-0.310899505813355,0.0957984565762295,
-5.56374924532966));
#28981=CARTESIAN_POINT('Ctrl Pts',(-0.248985264098286,-0.209385255567195,
-5.54786365990517));
#28982=CARTESIAN_POINT('Ctrl Pts',(0.0410579069103138,-0.322722938881596,
-5.53197807448065));
#28983=CARTESIAN_POINT('Ctrl Pts',(0.293482400465685,-0.140370679319073,
-5.51609248905615));
#28984=CARTESIAN_POINT('Ctrl Pts',(0.27700814599902,0.170594062161754,-5.50020690363163));
#28985=CARTESIAN_POINT('Ctrl Pts',(0.0067294264927366,0.32525461075211,
-5.48432131820714));
#28986=CARTESIAN_POINT('Ctrl Pts',(-0.269715026823541,0.181905610966966,
-5.46843573278263));
#28987=CARTESIAN_POINT('Ctrl Pts',(-0.299037223679916,-0.128111614810828,
-5.45255014735812));
#28988=CARTESIAN_POINT('Ctrl Pts',(-0.0543711509494218,-0.320748538485051,
-5.43666456193362));
#28989=CARTESIAN_POINT('Ctrl Pts',(0.240111654898234,-0.219504533387761,
-5.4207789765091));
#28990=CARTESIAN_POINT('Ctrl Pts',(0.314595839758998,0.0828571336825043,
-5.4048933910846));
#28991=CARTESIAN_POINT('Ctrl Pts',(0.100836411686931,0.30930222287252,-5.38900780566009));
#28992=CARTESIAN_POINT('Ctrl Pts',(-0.205312831972345,0.252353894408739,
-5.37312222023558));
#28993=CARTESIAN_POINT('Ctrl Pts',(-0.323347342409049,-0.0358098192227868,
-5.35723663481108));
#28994=CARTESIAN_POINT('Ctrl Pts',(-0.145119809839629,-0.29116333523965,
-5.34135104938657));
#28995=CARTESIAN_POINT('Ctrl Pts',(0.166071522659101,-0.279742911183559,
-5.32546546396207));
#28996=CARTESIAN_POINT('Ctrl Pts',(0.325102369713409,-0.0120123354303517,
-5.30957987853755));
#28997=CARTESIAN_POINT('Ctrl Pts',(0.186263156912436,0.266724358416659,
-5.29369429311305));
#28998=CARTESIAN_POINT('Ctrl Pts',(-0.123236816519873,0.30107894986168,
-5.27780870768855));
#28999=CARTESIAN_POINT('Ctrl Pts',(-0.319822947012469,0.0595745714212406,
-5.26192312226403));
#29000=CARTESIAN_POINT('Ctrl Pts',(-0.22337620772415,-0.23651409433381,
-5.24603753683954));
#29001=CARTESIAN_POINT('Ctrl Pts',(0.0777355557646795,-0.315900348790123,
-5.23015195141502));
#29002=CARTESIAN_POINT('Ctrl Pts',(0.307623308585974,-0.105847753922241,
-5.21426636599052));
#29003=CARTESIAN_POINT('Ctrl Pts',(0.255655923217533,0.201186221992351,
-5.198380780566));
#29004=CARTESIAN_POINT('Ctrl Pts',(-0.0305522805684868,0.323886407784935,
-5.1824951951415));
#29005=CARTESIAN_POINT('Ctrl Pts',(-0.288767425892113,0.149830640188875,
-5.166609609717));
#29006=CARTESIAN_POINT('Ctrl Pts',(-0.282403846334204,-0.161505153389643,
-5.15072402429249));
#29007=CARTESIAN_POINT('Ctrl Pts',(-0.0172920740606111,-0.324864327328267,
-5.13483843886798));
#29008=CARTESIAN_POINT('Ctrl Pts',(0.263663295846542,-0.190571544095922,
-5.11895285344348));
#29009=CARTESIAN_POINT('Ctrl Pts',(0.30304121498124,0.118329493442925,-5.10306726801897));
#29010=CARTESIAN_POINT('Ctrl Pts',(0.0647622689117458,0.318812947543176,
-5.08718168259446));
#29011=CARTESIAN_POINT('Ctrl Pts',(-0.232854112729537,0.227188928384957,
-5.07129609716995));
#29012=CARTESIAN_POINT('Ctrl Pts',(-0.317121485080486,-0.072593461800026,
-5.05541051174545));
#29013=CARTESIAN_POINT('Ctrl Pts',(-0.11083116071089,-0.305863206043554,
-5.03952492632094));
#29014=CARTESIAN_POINT('Ctrl Pts',(0.197006514740415,-0.258890479055526,
-5.02363934089643));
#29015=CARTESIAN_POINT('Ctrl Pts',(0.324339992731277,0.0252866785252807,
-5.00775375547193));
#29016=CARTESIAN_POINT('Ctrl Pts',(0.154501927083457,0.286295304752389,
-4.99186817004741));
#29017=CARTESIAN_POINT('Ctrl Pts',(-0.156896159516148,0.284990249175035,
-4.97598258462292));
#29018=CARTESIAN_POINT('Ctrl Pts',(-0.324540546420063,0.0225672489491302,
-4.9600969991984));
#29019=CARTESIAN_POINT('Ctrl Pts',(-0.194829635444025,-0.260532646991722,
-4.9442114137739));
#29020=CARTESIAN_POINT('Ctrl Pts',(0.113390940725942,-0.304923501155701,
-4.92832582834939));
#29021=CARTESIAN_POINT('Ctrl Pts',(0.317718806637116,-0.0699328742784981,
-4.91244024292489));
#29022=CARTESIAN_POINT('Ctrl Pts',(0.230941689113151,0.229132676031443,
-4.89655465750038));
#29023=CARTESIAN_POINT('Ctrl Pts',(-0.0674322088952368,0.318258926346574,
-4.88066907207587));
#29024=CARTESIAN_POINT('Ctrl Pts',(-0.304022379773291,0.115785316827091,
-4.86478348665136));
#29025=CARTESIAN_POINT('Ctrl Pts',(-0.262056708255467,-0.192774813329111,
-4.84889790122685));
#29026=CARTESIAN_POINT('Ctrl Pts',(0.020014402796204,-0.324707977537473,
-4.83301231580236));
#29027=CARTESIAN_POINT('Ctrl Pts',(0.283747624265194,-0.1591324376726,-4.81712673037784));
#29028=CARTESIAN_POINT('Ctrl Pts',(0.287501437099989,0.152245757448955,
-4.80124114495334));
#29029=CARTESIAN_POINT('Ctrl Pts',(0.0278364678663976,0.324131112441382,
-4.78535555952883));
#29030=CARTESIAN_POINT('Ctrl Pts',(-0.257333238096221,0.199036307156957,
-4.76946997410432));
#29031=CARTESIAN_POINT('Ctrl Pts',(-0.306725311610187,-0.108422461756772,
-4.75358438867982));
#29032=CARTESIAN_POINT('Ctrl Pts',(-0.0750850228900749,-0.316540813061068,
-4.73769880325531));
#29033=CARTESIAN_POINT('Ctrl Pts',(0.225350766404881,-0.234633499476306,
-4.7218132178308));
#29034=CARTESIAN_POINT('Ctrl Pts',(0.319312372393732,0.0622531592134212,
-4.7059276324063));
#29035=CARTESIAN_POINT('Ctrl Pts',(0.120708914764934,0.302101315607921,
-4.69004204698178));
#29036=CARTESIAN_POINT('Ctrl Pts',(-0.188492234593375,0.265153775182933,
-4.67415646155729));
#29037=CARTESIAN_POINT('Ctrl Pts',(-0.324990265084604,-0.0147368448456257,
-4.65827087613277));
#29038=CARTESIAN_POINT('Ctrl Pts',(-0.163720949867243,-0.281125056816949,
-4.64238529070827));
#29039=CARTESIAN_POINT('Ctrl Pts',(0.1475551745269,-0.2899367473538,-4.62649970528376));
#29040=CARTESIAN_POINT('Ctrl Pts',(0.323636133450456,-0.0330983401548074,
-4.61061411985925));
#29041=CARTESIAN_POINT('Ctrl Pts',(0.203190449005647,0.254065913551284,
-4.59472853443475));
#29042=CARTESIAN_POINT('Ctrl Pts',(-0.103425367821428,0.308446170809053,
-4.57884294901024));
#29043=CARTESIAN_POINT('Ctrl Pts',(-0.315279277712293,0.0802173549861858,
-4.56295736358573));
#29044=CARTESIAN_POINT('Ctrl Pts',(-0.238263385128086,-0.221509381975279,
-4.54707177816123));
#29045=CARTESIAN_POINT('Ctrl Pts',(0.0570576796146275,-0.32028154519541,
-4.53118619273672));
#29046=CARTESIAN_POINT('Ctrl Pts',(0.300100520556651,-0.12560065508345,
-4.51530060731221));
#29047=CARTESIAN_POINT('Ctrl Pts',(0.268180862456874,0.184159908795732,
-4.4994150218877));
#29048=CARTESIAN_POINT('Ctrl Pts',(-0.00945539753199466,0.325186780871051,
-4.4835294364632));
#29049=CARTESIAN_POINT('Ctrl Pts',(-0.278428294558318,0.168266252662592,
-4.46764385103869));
#29050=CARTESIAN_POINT('Ctrl Pts',(-0.292295537206912,-0.142825648693389,
-4.45175826561419));
#29051=CARTESIAN_POINT('Ctrl Pts',(-0.0383514770956826,-0.323055740082643,
-4.43587268018968));
#29052=CARTESIAN_POINT('Ctrl Pts',(0.250731535672522,-0.207290964624762,
-4.41998709476517));
#29053=CARTESIAN_POINT('Ctrl Pts',(0.310085624581392,0.0984009777580124,
-4.40410150934067));
#29054=CARTESIAN_POINT('Ctrl Pts',(0.0853285160365348,0.313934533536481,
-4.38821592391616));
#29055=CARTESIAN_POINT('Ctrl Pts',(-0.217609536564715,0.241830388065385,
-4.37233033849165));
#29056=CARTESIAN_POINT('Ctrl Pts',(-0.321166188966538,-0.0518471412951069,
-4.35644475306714));
#29057=CARTESIAN_POINT('Ctrl Pts',(-0.13045924674957,-0.298020522671343,
-4.34055916764264));
#29058=CARTESIAN_POINT('Ctrl Pts',(0.179778979328005,-0.271137171165345,
-4.32467358221813));
#29059=CARTESIAN_POINT('Ctrl Pts',(0.325297473032169,0.00417145474024782,
-4.30878799679362));
#29060=CARTESIAN_POINT('Ctrl Pts',(0.17276714645772,0.275658049221534,-4.29290241136911));
#29061=CARTESIAN_POINT('Ctrl Pts',(-0.138058428169682,0.294577184125114,
-4.27701682594462));
#29062=CARTESIAN_POINT('Ctrl Pts',(-0.322390085515951,0.0435944922757886,
-4.2611312405201));
#29063=CARTESIAN_POINT('Ctrl Pts',(-0.211336771802054,-0.247330984472329,
-4.2452456550956));
#29064=CARTESIAN_POINT('Ctrl Pts',(0.0933506176086514,-0.3116432402409,
-4.22936006967109));
#29065=CARTESIAN_POINT('Ctrl Pts',(0.312506935439882,-0.0904171570983101,
-4.21347448424658));
#29066=CARTESIAN_POINT('Ctrl Pts',(0.24533356688116,0.213652259424352,-4.19758889882208));
#29067=CARTESIAN_POINT('Ctrl Pts',(-0.0466229194254129,0.321966070231031,
-4.18170331339757));
#29068=CARTESIAN_POINT('Ctrl Pts',(-0.295861870907166,0.135283407478856,
-4.16581772797306));
#29069=CARTESIAN_POINT('Ctrl Pts',(-0.274021921076313,-0.17535060240956,
-4.14993214254855));
#29070=CARTESIAN_POINT('Ctrl Pts',(-0.00111358898614249,-0.325322312353944,
-4.13404655712405));
#29071=CARTESIAN_POINT('Ctrl Pts',(0.2728150519327,-0.177222443372218,-4.11816097169954));
#29072=CARTESIAN_POINT('Ctrl Pts',(0.296781085933562,0.133254771125564,
-4.10227538627503));
#29073=CARTESIAN_POINT('Ctrl Pts',(0.0488260019537641,0.321639345430405,
-4.08638980085053));
#29074=CARTESIAN_POINT('Ctrl Pts',(-0.243865157428648,0.215326802764376,
-4.07050421542601));
#29075=CARTESIAN_POINT('Ctrl Pts',(-0.313118606698104,-0.0882756202702708,
-4.05461863000152));
#29076=CARTESIAN_POINT('Ctrl Pts',(-0.0954819351759957,-0.310996860194193,
-4.038733044577));
#29077=CARTESIAN_POINT('Ctrl Pts',(0.209638594970145,-0.24877199701569,
-4.0228474591525));
#29078=CARTESIAN_POINT('Ctrl Pts',(0.322680977869204,0.0413863927928797,
-4.00696187372799));
#29079=CARTESIAN_POINT('Ctrl Pts',(0.140071864101366,0.293625134967264,
-3.99107628830348));
#29080=CARTESIAN_POINT('Ctrl Pts',(-0.170875946835193,0.276834350863799,
-3.97519070287898));
#29081=CARTESIAN_POINT('Ctrl Pts',(-0.32526129217821,0.00639833877413384,
-3.95930511745447));
#29082=CARTESIAN_POINT('Ctrl Pts',(-0.181630967757783,-0.269900052943306,
-3.94341953202997));
#29083=CARTESIAN_POINT('Ctrl Pts',(0.128415945730084,-0.298906661121661,
-3.92753394660546));
#29084=CARTESIAN_POINT('Ctrl Pts',(0.320803717221891,-0.0540446251432457,
-3.91164836118095));
#29085=CARTESIAN_POINT('Ctrl Pts',(0.219260005889228,0.24033496870297,-3.89576277575645));
#29086=CARTESIAN_POINT('Ctrl Pts',(-0.0831773279059596,0.314511335622391,
-3.87987719033193));
#29087=CARTESIAN_POINT('Ctrl Pts',(-0.309404700997039,0.100521511539756,
-3.86399160490743));
#29088=CARTESIAN_POINT('Ctrl Pts',(-0.252144781320854,-0.205569598572242,
-3.84810601948292));
#29089=CARTESIAN_POINT('Ctrl Pts',(0.0361389633827169,-0.323310730778187,
-3.83222043405842));
#29090=CARTESIAN_POINT('Ctrl Pts',(0.291310866606552,-0.144823338200814,
-3.81633484863391));
#29091=CARTESIAN_POINT('Ctrl Pts',(0.279573792802751,0.1663561652634,-3.8004492632094));
#29092=CARTESIAN_POINT('Ctrl Pts',(0.0116812558217563,0.325114483296725,
-3.7845636777849));
#29093=CARTESIAN_POINT('Ctrl Pts',(-0.266913543199629,0.185991450423231,
-3.76867809236039));
#29094=CARTESIAN_POINT('Ctrl Pts',(-0.300953886710748,-0.123543024795751,
-3.75279250693588));
#29095=CARTESIAN_POINT('Ctrl Pts',(-0.0592479447871856,-0.319883816175267,
-3.73690692151138));
#29096=CARTESIAN_POINT('Ctrl Pts',(0.236739340552828,-0.223134580234524,
-3.72102133608687));
#29097=CARTESIAN_POINT('Ctrl Pts',(0.315824942891063,0.0780556116991824,
-3.70513575066236));
#29098=CARTESIAN_POINT('Ctrl Pts',(0.105527050933059,0.307733727437991,
-3.68925016523785));
#29099=CARTESIAN_POINT('Ctrl Pts',(-0.201431839230644,0.255445522700207,
-3.67336457981334));
#29100=CARTESIAN_POINT('Ctrl Pts',(-0.323883197730372,-0.0308713713365518,
-3.65747899438885));
#29101=CARTESIAN_POINT('Ctrl Pts',(-0.149482368799369,-0.288940268144714,
-3.64159340896433));
#29102=CARTESIAN_POINT('Ctrl Pts',(0.161687434173921,-0.282199540627596,
-3.62570782353983));
#29103=CARTESIAN_POINT('Ctrl Pts',(0.325087357461483,-0.0170400391236926,
-3.60982223811532));
#29104=CARTESIAN_POINT('Ctrl Pts',(0.189881717319456,0.264026794694474,
-3.59393665269081));
#29105=CARTESIAN_POINT('Ctrl Pts',(-0.0151027964452971,0.289629518398212,
-3.58334626240781));
#29106=CARTESIAN_POINT('Ctrl Pts',(-0.100355771007372,0.256240458609279,
-3.57805106726631));
#29107=CARTESIAN_POINT('Ctrl Pts',(-0.128892185405323,0.264462557919717,
-5.9658));
#29108=CARTESIAN_POINT('Ctrl Pts',(-0.216880709330539,0.22157923549964,
-5.9605048048585));
#29109=CARTESIAN_POINT('Ctrl Pts',(-0.345156657723216,0.0418063155382426,
-5.94991441457549));
#29110=CARTESIAN_POINT('Ctrl Pts',(-0.221968912512454,-0.268043282517462,
-5.93402882915099));
#29111=CARTESIAN_POINT('Ctrl Pts',(0.104905157196136,-0.331499645408673,
-5.91814324372647));
#29112=CARTESIAN_POINT('Ctrl Pts',(0.335502751086021,-0.0916215029918852,
-5.90225765830198));
#29113=CARTESIAN_POINT('Ctrl Pts',(0.258783020342812,0.232406939929434,
-5.88637207287745));
#29114=CARTESIAN_POINT('Ctrl Pts',(-0.0550850529492111,0.343390984503182,
-5.87048648745297));
#29115=CARTESIAN_POINT('Ctrl Pts',(-0.318460370178621,0.139802670944853,
-5.85460090202845));
#29116=CARTESIAN_POINT('Ctrl Pts',(-0.290062600329783,-0.191905823647729,
-5.83871531660395));
#29117=CARTESIAN_POINT('Ctrl Pts',(0.00410644714618952,-0.347768996506744,
-5.82282973117944));
#29118=CARTESIAN_POINT('Ctrl Pts',(0.294509988563641,-0.18500169123973,
-5.80694414575493));
#29119=CARTESIAN_POINT('Ctrl Pts',(0.315074841503008,0.1472744728238,-5.79105856033042));
#29120=CARTESIAN_POINT('Ctrl Pts',(0.046956390424147,0.344610643734406,
-5.77517297490592));
#29121=CARTESIAN_POINT('Ctrl Pts',(-0.264184712448466,0.226203641246638,
-5.75928738948141));
#29122=CARTESIAN_POINT('Ctrl Pts',(-0.333270842279612,-0.0994595178868144,
-5.7434018040569));
#29123=CARTESIAN_POINT('Ctrl Pts',(-0.097002561910864,-0.333994139922494,
-5.7275162186324));
#29124=CARTESIAN_POINT('Ctrl Pts',(0.228142769705393,-0.262511898568683,
-5.71163063320788));
#29125=CARTESIAN_POINT('Ctrl Pts',(0.344255817974058,0.0494929182512338,
-5.69574504778339));
#29126=CARTESIAN_POINT('Ctrl Pts',(0.144949737587321,0.316150569143213,
-5.67985946235887));
#29127=CARTESIAN_POINT('Ctrl Pts',(-0.187164308561312,0.293140130174455,
-5.66397387693438));
#29128=CARTESIAN_POINT('Ctrl Pts',(-0.347791931880303,0.00154453273246722,
-5.64808829150985));
#29129=CARTESIAN_POINT('Ctrl Pts',(-0.189760529857378,-0.291466213774469,
-5.63220270608536));
#29130=CARTESIAN_POINT('Ctrl Pts',(0.14213604599659,-0.317425515170563,
-5.61631712066084));
#29131=CARTESIAN_POINT('Ctrl Pts',(0.343802650356538,-0.0525485555038461,
-5.60043153523635));
#29132=CARTESIAN_POINT('Ctrl Pts',(0.230465349245865,0.260475211414911,
-5.58454594981184));
#29133=CARTESIAN_POINT('Ctrl Pts',(-0.0940322930969158,0.334842561407425,
-5.56866036438732));
#29134=CARTESIAN_POINT('Ctrl Pts',(-0.33237428922977,0.102415550100451,
-5.55277477896283));
#29135=CARTESIAN_POINT('Ctrl Pts',(-0.266183440745114,-0.223848138041494,
-5.53688919353831));
#29136=CARTESIAN_POINT('Ctrl Pts',(0.0438939026000584,-0.345014403121335,
-5.52100360811381));
#29137=CARTESIAN_POINT('Ctrl Pts',(0.31375413094027,-0.150066513117541,
-5.5051180226893));
#29138=CARTESIAN_POINT('Ctrl Pts',(0.296141949136947,0.182377517807546,
-5.4892324372648));
#29139=CARTESIAN_POINT('Ctrl Pts',(0.00719424864184242,0.347720945340898,
-5.47334685184028));
#29140=CARTESIAN_POINT('Ctrl Pts',(-0.288345071828068,0.194470390018404,
-5.45746126641578));
#29141=CARTESIAN_POINT('Ctrl Pts',(-0.319692642848795,-0.136960677384898,
-5.44157568099127));
#29142=CARTESIAN_POINT('Ctrl Pts',(-0.0581267332803917,-0.34290362482743,
-5.42569009556676));
#29143=CARTESIAN_POINT('Ctrl Pts',(0.256696904113111,-0.234666385450186,
-5.40980451014226));
#29144=CARTESIAN_POINT('Ctrl Pts',(0.336325940309834,0.0885803303009154,
-5.39391892471776));
#29145=CARTESIAN_POINT('Ctrl Pts',(0.107801492238604,0.330666677052099,
-5.37803333929324));
#29146=CARTESIAN_POINT('Ctrl Pts',(-0.219494419645449,0.269784752693763,
-5.36214775386874));
#29147=CARTESIAN_POINT('Ctrl Pts',(-0.345681936117525,-0.0382833133828322,
-5.34626216844423));
#29148=CARTESIAN_POINT('Ctrl Pts',(-0.155143680664333,-0.311274880758883,
-5.33037658301973));
#29149=CARTESIAN_POINT('Ctrl Pts',(0.177542592615962,-0.299065612949288,
-5.31449099759522));
#29150=CARTESIAN_POINT('Ctrl Pts',(0.34755818854623,-0.0128420643198113,
-5.29860541217071));
#29151=CARTESIAN_POINT('Ctrl Pts',(0.199128925041234,0.28514782877212,-5.28271982674621));
#29152=CARTESIAN_POINT('Ctrl Pts',(-0.13174916180897,0.321875397326613,
-5.26683424132169));
#29153=CARTESIAN_POINT('Ctrl Pts',(-0.341914099910008,0.0636895699801798,
-5.25094865589719));
#29154=CARTESIAN_POINT('Ctrl Pts',(-0.238805488220131,-0.252850848994968,
-5.23506307047268));
#29155=CARTESIAN_POINT('Ctrl Pts',(0.0831049892716063,-0.337720555784953,
-5.21917748504817));
#29156=CARTESIAN_POINT('Ctrl Pts',(0.328871795001037,-0.113158983268353,
-5.20329189962367));
#29157=CARTESIAN_POINT('Ctrl Pts',(0.273314862770547,0.215082772044271,
-5.18740631419916));
#29158=CARTESIAN_POINT('Ctrl Pts',(-0.0326626203915411,0.346258236394009,
-5.17152072877465));
#29159=CARTESIAN_POINT('Ctrl Pts',(-0.308713478596589,0.16017990252939,
-5.15563514335015));
#29160=CARTESIAN_POINT('Ctrl Pts',(-0.301910347060617,-0.17266081020101,
-5.13974955792564));
#29161=CARTESIAN_POINT('Ctrl Pts',(-0.0184864907075617,-0.347303703842689,
-5.12386397250114));
#29162=CARTESIAN_POINT('Ctrl Pts',(0.281875329211953,-0.203734905755456,
-5.10797838707663));
#29163=CARTESIAN_POINT('Ctrl Pts',(0.323973202122692,0.12650287486022,-5.09209280165213));
#29164=CARTESIAN_POINT('Ctrl Pts',(0.0692355976640608,0.340834336676386,
-5.07620721622761));
#29165=CARTESIAN_POINT('Ctrl Pts',(-0.248938061224104,0.242881565203116,
-5.06032163080311));
#29166=CARTESIAN_POINT('Ctrl Pts',(-0.339026039708127,-0.0776077150891233,
-5.0444360453786));
#29167=CARTESIAN_POINT('Ctrl Pts',(-0.118486609264369,-0.326990116771997,
-5.02855045995409));
#29168=CARTESIAN_POINT('Ctrl Pts',(0.210614359579554,-0.276772839311276,
-5.01266487452959));
#29169=CARTESIAN_POINT('Ctrl Pts',(0.346743151845229,0.027033307048315,
-4.99677928910507));
#29170=CARTESIAN_POINT('Ctrl Pts',(0.165173849551959,0.306070600459629,
-4.98089370368058));
#29171=CARTESIAN_POINT('Ctrl Pts',(-0.167733458969751,0.304675400686655,
-4.96500811825607));
#29172=CARTESIAN_POINT('Ctrl Pts',(-0.346957558393056,0.0241260381219176,
-4.94912253283156));
#29173=CARTESIAN_POINT('Ctrl Pts',(-0.208287116546523,-0.278528436828748,
-4.93323694740706));
#29174=CARTESIAN_POINT('Ctrl Pts',(0.121223201144314,-0.325985503582378,
-4.91735136198254));
#29175=CARTESIAN_POINT('Ctrl Pts',(0.33966462009862,-0.074763352618723,
-4.90146577655805));
#29176=CARTESIAN_POINT('Ctrl Pts',(0.24689354063685,0.244959573467403,-4.88558019113352));
#29177=CARTESIAN_POINT('Ctrl Pts',(-0.0720899585996865,0.340242047534732,
-4.86969460570903));
#29178=CARTESIAN_POINT('Ctrl Pts',(-0.325022138979386,0.123782964154184,
-4.85380902028452));
#29179=CARTESIAN_POINT('Ctrl Pts',(-0.280157769683282,-0.206090361559246,
-4.83792343486001));
#29180=CARTESIAN_POINT('Ctrl Pts',(0.0213968590472457,-0.347136554491807,
-4.82203784943551));
#29181=CARTESIAN_POINT('Ctrl Pts',(0.30334694385908,-0.170124203724479,
-4.80615226401099));
#29182=CARTESIAN_POINT('Ctrl Pts',(0.307360044071647,0.16276183935372,-4.7902666785865));
#29183=CARTESIAN_POINT('Ctrl Pts',(0.0297592181678009,0.346519843552389,
-4.77438109316198));
#29184=CARTESIAN_POINT('Ctrl Pts',(-0.27510803493774,0.212784355990346,
-4.75849550773748));
#29185=CARTESIAN_POINT('Ctrl Pts',(-0.327911770617026,-0.1159115340781,
-4.74260992231297));
#29186=CARTESIAN_POINT('Ctrl Pts',(-0.0802713759534626,-0.3384052588895,
-4.72672433688846));
#29187=CARTESIAN_POINT('Ctrl Pts',(0.240916435731397,-0.250840355676695,
-4.71083875146396));
#29188=CARTESIAN_POINT('Ctrl Pts',(0.341368258334745,0.0665531760551926,
-4.69495316603944));
#29189=CARTESIAN_POINT('Ctrl Pts',(0.129046650118439,0.322968381013901,
-4.67906758061495));
#29190=CARTESIAN_POINT('Ctrl Pts',(-0.201511971961497,0.283468760532303,
-4.66318199519044));
#29191=CARTESIAN_POINT('Ctrl Pts',(-0.347438340506522,-0.0157547639654172,
-4.64729640976592));
#29192=CARTESIAN_POINT('Ctrl Pts',(-0.175029658544443,-0.300543227625157,
-4.63141082434143));
#29193=CARTESIAN_POINT('Ctrl Pts',(0.157747263467816,-0.309963568681783,
-4.61552523891691));
#29194=CARTESIAN_POINT('Ctrl Pts',(0.345990674842834,-0.0353845441306157,
-4.59963965349241));
#29195=CARTESIAN_POINT('Ctrl Pts',(0.217225437170922,0.271615026254869,
-4.5837540680679));
#29196=CARTESIAN_POINT('Ctrl Pts',(-0.110569275522142,0.329751494844285,
-4.5678684826434));
#29197=CARTESIAN_POINT('Ctrl Pts',(-0.337056585420913,0.085758213985171,
-4.55198289721889));
#29198=CARTESIAN_POINT('Ctrl Pts',(-0.254720968675225,-0.2368097150851,
-4.53609731179438));
#29199=CARTESIAN_POINT('Ctrl Pts',(0.0609988287289104,-0.342404374877472,
-4.52021172636987));
#29200=CARTESIAN_POINT('Ctrl Pts',(0.32082938490543,-0.134276277959789,
-4.50432614094537));
#29201=CARTESIAN_POINT('Ctrl Pts',(0.286704938018275,0.196880399119539,
-4.48844055552086));
#29202=CARTESIAN_POINT('Ctrl Pts',(-0.0101085108702889,0.347648430241697,
-4.47255497009635));
#29203=CARTESIAN_POINT('Ctrl Pts',(-0.297660191717496,0.179888919359239,
-4.45666938467184));
#29204=CARTESIAN_POINT('Ctrl Pts',(-0.312485287392206,-0.152691054763995,
-4.44078379924734));
#29205=CARTESIAN_POINT('Ctrl Pts',(-0.0410005313686208,-0.345370191923133,
-4.42489821382283));
#29206=CARTESIAN_POINT('Ctrl Pts',(0.268050332658533,-0.221609187993598,
-4.40901262839833));
#29207=CARTESIAN_POINT('Ctrl Pts',(0.331504190722268,0.10519783541074,-4.39312704297382));
#29208=CARTESIAN_POINT('Ctrl Pts',(0.0912224186219852,0.33561895563613,
-4.37724145754931));
#29209=CARTESIAN_POINT('Ctrl Pts',(-0.232640495378394,0.258534355457117,
-4.36135587212481));
#29210=CARTESIAN_POINT('Ctrl Pts',(-0.34335012370998,-0.0554283825298268,
-4.3454702867003));
#29211=CARTESIAN_POINT('Ctrl Pts',(-0.139470467469546,-0.318605715179998,
-4.32958470127579));
#29212=CARTESIAN_POINT('Ctrl Pts',(0.192196865402776,-0.289865448045948,
-4.31369911585128));
#29213=CARTESIAN_POINT('Ctrl Pts',(0.347766768250241,0.00445958992670925,
-4.29781353042678));
#29214=CARTESIAN_POINT('Ctrl Pts',(0.18470070370782,0.294698597029859,-4.28192794500227));
#29215=CARTESIAN_POINT('Ctrl Pts',(-0.147594547681994,0.314924534668353,
-4.26604235957776));
#29216=CARTESIAN_POINT('Ctrl Pts',(-0.34465855855177,0.0466056977047642,
-4.25015677415325));
#29217=CARTESIAN_POINT('Ctrl Pts',(-0.225934451494405,-0.264414894946282,
-4.23427118872876));
#29218=CARTESIAN_POINT('Ctrl Pts',(0.0997986313798216,-0.333169395677702,
-4.21838560330424));
#29219=CARTESIAN_POINT('Ctrl Pts',(0.334092748955866,-0.0966625477454723,
-4.20250001787973));
#29220=CARTESIAN_POINT('Ctrl Pts',(0.262279509589452,0.22840987695598,-4.18661443245523));
#29221=CARTESIAN_POINT('Ctrl Pts',(-0.0498433076157462,0.344205255229274,
-4.17072884703072));
#29222=CARTESIAN_POINT('Ctrl Pts',(-0.316297958710795,0.144627847791949,
-4.15484326160621));
#29223=CARTESIAN_POINT('Ctrl Pts',(-0.29294945649027,-0.187462606894199,
-4.13895767618171));
#29224=CARTESIAN_POINT('Ctrl Pts',(-0.00119050799645002,-0.347793323300234,
-4.1230720907572));
#29225=CARTESIAN_POINT('Ctrl Pts',(0.291659225189475,-0.189463741659231,
-4.1071865053327));
#29226=CARTESIAN_POINT('Ctrl Pts',(0.317280666741316,0.142459087297245,
-4.09130091990818));
#29227=CARTESIAN_POINT('Ctrl Pts',(0.0521985638184197,0.343855962543531,
-4.07541533448368));
#29228=CARTESIAN_POINT('Ctrl Pts',(-0.26070967258762,0.230200086145824,
-4.05952974905918));
#29229=CARTESIAN_POINT('Ctrl Pts',(-0.334746670225899,-0.0943730883935936,
-4.04364416363466));
#29230=CARTESIAN_POINT('Ctrl Pts',(-0.102077165595292,-0.332478368176598,
-4.02775857821017));
#29231=CARTESIAN_POINT('Ctrl Pts',(0.224118976374829,-0.265955442650332,
-4.01187299278565));
#29232=CARTESIAN_POINT('Ctrl Pts',(0.344969543732986,0.0442450780110779,
-3.99598740736115));
#29233=CARTESIAN_POINT('Ctrl Pts',(0.149747057815299,0.313906724552109,
-3.98010182193664));
#29234=CARTESIAN_POINT('Ctrl Pts',(-0.182678873120845,0.295956149438136,
-3.96421623651213));
#29235=CARTESIAN_POINT('Ctrl Pts',(-0.347728088273613,0.00684029167798261,
-3.94833065108763));
#29236=CARTESIAN_POINT('Ctrl Pts',(-0.19417677635953,-0.288542878270008,
-3.93244506566312));
#29237=CARTESIAN_POINT('Ctrl Pts',(0.137286029375129,-0.319553061933777,
-3.91655948023861));
#29238=CARTESIAN_POINT('Ctrl Pts',(0.342962614929039,-0.0577776533342563,
-3.9006738948141));
#29239=CARTESIAN_POINT('Ctrl Pts',(0.234404967686561,0.256935642887977,
-3.8847883093896));
#29240=CARTESIAN_POINT('Ctrl Pts',(-0.0889226413224721,0.33623559921306,
-3.86890272396509));
#29241=CARTESIAN_POINT('Ctrl Pts',(-0.330776233655315,0.107464840971431,
-3.85301713854058));
#29242=CARTESIAN_POINT('Ctrl Pts',(-0.26956119552286,-0.219768921902748,
-3.83713155311608));
#29243=CARTESIAN_POINT('Ctrl Pts',(0.0386351925404547,-0.345642795608912,
-3.82124596769157));
#29244=CARTESIAN_POINT('Ctrl Pts',(0.311432602570261,-0.154826730819173,
-3.80536038226707));
#29245=CARTESIAN_POINT('Ctrl Pts',(0.298884813042677,0.177846896358873,
-3.78947479684255));
#29246=CARTESIAN_POINT('Ctrl Pts',(0.0124881160261418,0.347571138851938,
-3.77358921141805));
#29247=CARTESIAN_POINT('Ctrl Pts',(-0.285350081128901,0.198838450950602,
-3.75770362599354));
#29248=CARTESIAN_POINT('Ctrl Pts',(-0.321741695679867,-0.132076520830608,
-3.74181804056904));
#29249=CARTESIAN_POINT('Ctrl Pts',(-0.0633403822416737,-0.341979173492766,
-3.72593245514453));
#29250=CARTESIAN_POINT('Ctrl Pts',(0.253091653661904,-0.238547170777931,
-3.71004686972002));
#29251=CARTESIAN_POINT('Ctrl Pts',(0.337639941368927,0.0834471524521679,
-3.69416128429552));
#29252=CARTESIAN_POINT('Ctrl Pts',(0.112816128339058,0.32898984082218,-3.678275698871));
#29253=CARTESIAN_POINT('Ctrl Pts',(-0.215345354819328,0.2730899292435,-3.66239011344651));
#29254=CARTESIAN_POINT('Ctrl Pts',(-0.346254804611121,-0.0330037517386558,
-3.64650452802199));
#29255=CARTESIAN_POINT('Ctrl Pts',(-0.159807574965718,-0.308898259594252,
-3.63061894259749));
#29256=CARTESIAN_POINT('Ctrl Pts',(0.172855681678712,-0.301691929331577,
-3.61473335717298));
#29257=CARTESIAN_POINT('Ctrl Pts',(0.347542139351973,-0.0182170469437311,
-3.59884777174848));
#29258=CARTESIAN_POINT('Ctrl Pts',(0.202997430525575,0.282263936041357,
-3.58296218632397));
#29259=CARTESIAN_POINT('Ctrl Pts',(-0.0161459929656535,0.309635118478954,
-3.57237179604096));
#29260=CARTESIAN_POINT('Ctrl Pts',(-0.107287652231604,0.273939773816491,
-3.56707660089946));
#29261=CARTESIAN_POINT('',(0.29192076924273,-0.0365500271509186,-3.6));
#29262=CARTESIAN_POINT('Ctrl Pts',(0.292414323780515,-0.0364994916172054,
-3.6));
#29263=CARTESIAN_POINT('Ctrl Pts',(0.292666487654641,-0.0294203594636345,
-3.6));
#29264=CARTESIAN_POINT('Ctrl Pts',(0.292644719912668,-0.0223426691634168,
-3.6));
#29265=CARTESIAN_POINT('Ctrl Pts',(0.292340298090172,-0.0152783476836462,
-3.6));
#29266=CARTESIAN_POINT('Ctrl Pts',(0.291819266745405,-0.00318745061757684,
-3.6));
#29267=CARTESIAN_POINT('Ctrl Pts',(0.290470817834819,0.0088645857384901,
-3.6));
#29268=CARTESIAN_POINT('Ctrl Pts',(0.288335912431399,0.020809913429241,
-3.6));
#29269=CARTESIAN_POINT('Ctrl Pts',(0.287324186550805,0.0264707718249139,
-3.6));
#29270=CARTESIAN_POINT('Ctrl Pts',(0.286135672242458,0.0321076021086892,
-3.6));
#29271=CARTESIAN_POINT('Ctrl Pts',(0.284773910663568,0.0377127213804415,
-3.6));
#29272=CARTESIAN_POINT('Ctrl Pts',(0.283356850440654,0.0435454542815746,
-3.6));
#29273=CARTESIAN_POINT('Ctrl Pts',(0.281753731857198,0.0493368411209126,
-3.6));
#29274=CARTESIAN_POINT('Ctrl Pts',(0.279972018733966,0.055071055872317,
-3.6));
#29275=CARTESIAN_POINT('Ctrl Pts',(0.274848939028037,0.0715590296315548,
-3.6));
#29276=CARTESIAN_POINT('Ctrl Pts',(0.268247408855639,0.0875967881401878,
-3.6));
#29277=CARTESIAN_POINT('Ctrl Pts',(0.260271123750079,0.102974430970234,
-3.6));
#29278=CARTESIAN_POINT('Ctrl Pts',(0.257522628682807,0.108273310699995,
-3.6));
#29279=CARTESIAN_POINT('Ctrl Pts',(0.254608896221931,0.113495680260488,
-3.6));
#29280=CARTESIAN_POINT('Ctrl Pts',(0.251546120022716,0.118612125015772,
-3.6));
#29281=CARTESIAN_POINT('Ctrl Pts',(0.242945994386678,0.132978851424501,
-3.6));
#29282=CARTESIAN_POINT('Ctrl Pts',(0.233156507997209,0.146548580458849,
-3.6));
#29283=CARTESIAN_POINT('Ctrl Pts',(0.222274509229499,0.159129353049593,
-3.6));
#29284=CARTESIAN_POINT('Ctrl Pts',(0.215201410731259,0.167306623201684,
-3.6));
#29285=CARTESIAN_POINT('Ctrl Pts',(0.207665946000832,0.175065453049953,
-3.6));
#29286=CARTESIAN_POINT('Ctrl Pts',(0.199688444759937,0.182342711212395,
-3.6));
#29287=CARTESIAN_POINT('Ctrl Pts',(0.196404264508349,0.185338615170426,
-3.6));
#29288=CARTESIAN_POINT('Ctrl Pts',(0.193045123181327,0.188252788830684,
-3.6));
#29289=CARTESIAN_POINT('Ctrl Pts',(0.189612281823844,0.191080315392676,
-3.6));
#29290=CARTESIAN_POINT('Ctrl Pts',(0.186193494325361,0.193896266220318,
-3.6));
#29291=CARTESIAN_POINT('Ctrl Pts',(0.182708690605058,0.19662039211184,-3.6));
#29292=CARTESIAN_POINT('Ctrl Pts',(0.179161622624937,0.199247529650452,
-3.6));
#29293=CARTESIAN_POINT('Ctrl Pts',(0.171408656339104,0.204989767712777,
-3.6));
#29294=CARTESIAN_POINT('Ctrl Pts',(0.163355483608744,0.210271516086989,
-3.6));
#29295=CARTESIAN_POINT('Ctrl Pts',(0.155019203531841,0.215050497759424,
-3.6));
#29296=CARTESIAN_POINT('Ctrl Pts',(0.140808457822457,0.223197164218598,
-3.6));
#29297=CARTESIAN_POINT('Ctrl Pts',(0.125774643211521,0.22988578386622,-3.6));
#29298=CARTESIAN_POINT('Ctrl Pts',(0.11014676513074,0.235093491948397,-3.6));
#29299=CARTESIAN_POINT('Ctrl Pts',(0.106087966374167,0.236446013319454,
-3.6));
#29300=CARTESIAN_POINT('Ctrl Pts',(0.101986598043523,0.237699037569938,
-3.6));
#29301=CARTESIAN_POINT('Ctrl Pts',(0.0978550841807309,0.23884928488335,
-3.6));
#29302=CARTESIAN_POINT('Ctrl Pts',(0.0826054374270896,0.243094911496596,
-3.6));
#29303=CARTESIAN_POINT('Ctrl Pts',(0.0670045393815982,0.245930050485186,
-3.6));
#29304=CARTESIAN_POINT('Ctrl Pts',(0.051262317664912,0.247351840499526,
-3.6));
#29305=CARTESIAN_POINT('Ctrl Pts',(0.039125047109517,0.248448042191229,
-3.6));
#29306=CARTESIAN_POINT('Ctrl Pts',(0.026903246465002,0.248702971880079,
-3.6));
#29307=CARTESIAN_POINT('Ctrl Pts',(0.0146976872519464,0.248094407813563,
-3.6));
#29308=CARTESIAN_POINT('Ctrl Pts',(0.0102876623740829,0.247874525821574,
-3.6));
#29309=CARTESIAN_POINT('Ctrl Pts',(0.00587781616497291,0.247541537797545,
-3.6));
#29310=CARTESIAN_POINT('Ctrl Pts',(0.00147967530992972,0.247094507554182,
-3.6));
#29311=CARTESIAN_POINT('Ctrl Pts',(-0.0139171193363565,0.245529566119927,
-3.6));
#29312=CARTESIAN_POINT('Ctrl Pts',(-0.0290846126574327,0.242581300092628,
-3.6));
#29313=CARTESIAN_POINT('Ctrl Pts',(-0.0438193177938728,0.238223133415296,
-3.6));
#29314=CARTESIAN_POINT('Ctrl Pts',(-0.0576495230985568,0.234132495744477,
-3.6));
#29315=CARTESIAN_POINT('Ctrl Pts',(-0.0710995093010162,0.228799086735258,
-3.6));
#29316=CARTESIAN_POINT('Ctrl Pts',(-0.0839735920665051,0.222161024970596,
-3.6));
#29317=CARTESIAN_POINT('Ctrl Pts',(-0.084815561179679,0.221726893617008,
-3.6));
#29318=CARTESIAN_POINT('Ctrl Pts',(-0.0856550535821104,0.221287168938323,
-3.6));
#29319=CARTESIAN_POINT('Ctrl Pts',(-0.0864920085589077,0.220841828194855,
-3.6));
#29320=CARTESIAN_POINT('Ctrl Pts',(-0.294584692827634,-0.000157098441292656,
-3.64801761170896));
#29321=CARTESIAN_POINT('Ctrl Pts',(-0.294645466431812,-0.00944699213001965,
-3.64751325047997));
#29322=CARTESIAN_POINT('Ctrl Pts',(-0.294243676282554,-0.0187316056112418,
-3.64700888925098));
#29323=CARTESIAN_POINT('Ctrl Pts',(-0.293362024704922,-0.0279705562175625,
-3.64650452802199));
#29324=CARTESIAN_POINT('Ctrl Pts',(-0.284105728062653,-0.124968587690521,
-3.64120933288049));
#29325=CARTESIAN_POINT('Ctrl Pts',(-0.221956651514186,-0.216933423642387,
-3.63591413773899));
#29326=CARTESIAN_POINT('Ctrl Pts',(-0.135438237132546,-0.26171478657454,
-3.63061894259749));
#29327=CARTESIAN_POINT('Ctrl Pts',(-0.048919822750907,-0.306496149506694,
-3.62532374745599));
#29328=CARTESIAN_POINT('Ctrl Pts',(0.0619679294639041,-0.304094039419135,
-3.62002855231448));
#29329=CARTESIAN_POINT('Ctrl Pts',(0.14652621518352,-0.255647170644047,
-3.61473335717298));
#29330=CARTESIAN_POINT('Ctrl Pts',(0.224951239641238,-0.210714295808048,
-3.60982223811532));
#29331=CARTESIAN_POINT('Ctrl Pts',(0.280727784900505,-0.126173943185802,
-3.60491111905766));
#29332=CARTESIAN_POINT('Ctrl Pts',(0.292414323780514,-0.0364994916172137,
-3.6));
#29333=CARTESIAN_POINT('',(-0.137702479013098,-0.193106208855768,-5.9658));
#29334=CARTESIAN_POINT('Ctrl Pts',(-0.138001922973978,-0.193371366051279,
-5.9658));
#29335=CARTESIAN_POINT('Ctrl Pts',(-0.143073358296614,-0.190612953673137,
-5.9658));
#29336=CARTESIAN_POINT('Ctrl Pts',(-0.148027594123821,-0.187662423150088,
-5.9658));
#29337=CARTESIAN_POINT('Ctrl Pts',(-0.152852356931864,-0.184522195146066,
-5.9658));
#29338=CARTESIAN_POINT('Ctrl Pts',(-0.162997379060741,-0.177919242035622,
-5.9658));
#29339=CARTESIAN_POINT('Ctrl Pts',(-0.172570666260329,-0.17047916665888,
-5.9658));
#29340=CARTESIAN_POINT('Ctrl Pts',(-0.181542838702178,-0.162315875140337,
-5.9658));
#29341=CARTESIAN_POINT('Ctrl Pts',(-0.186610812592755,-0.15770480145163,
-5.9658));
#29342=CARTESIAN_POINT('Ctrl Pts',(-0.191489654388371,-0.152858842458079,
-5.9658));
#29343=CARTESIAN_POINT('Ctrl Pts',(-0.19615336760798,-0.147818230112143,
-5.9658));
#29344=CARTESIAN_POINT('Ctrl Pts',(-0.203092451016376,-0.140318362978212,
-5.9658));
#29345=CARTESIAN_POINT('Ctrl Pts',(-0.209564344127366,-0.132381113357134,
-5.9658));
#29346=CARTESIAN_POINT('Ctrl Pts',(-0.215551335673081,-0.124070288249604,
-5.9658));
#29347=CARTESIAN_POINT('Ctrl Pts',(-0.219342144904121,-0.118808087310347,
-5.9658));
#29348=CARTESIAN_POINT('Ctrl Pts',(-0.222938463172683,-0.113395908629678,
-5.9658));
#29349=CARTESIAN_POINT('Ctrl Pts',(-0.226334587133058,-0.107848190686934,
-5.9658));
#29350=CARTESIAN_POINT('Ctrl Pts',(-0.228858498148498,-0.103725270973279,
-5.9658));
#29351=CARTESIAN_POINT('Ctrl Pts',(-0.231271645540891,-0.0995272197569029,
-5.9658));
#29352=CARTESIAN_POINT('Ctrl Pts',(-0.233564764998697,-0.0952733717887619,
-5.9658));
#29353=CARTESIAN_POINT('Ctrl Pts',(-0.241164174912553,-0.0811760973048323,
-5.9658));
#29354=CARTESIAN_POINT('Ctrl Pts',(-0.247469655098504,-0.0664351633284274,
-5.9658));
#29355=CARTESIAN_POINT('Ctrl Pts',(-0.252411117523312,-0.051269455660209,
-5.9658));
#29356=CARTESIAN_POINT('Ctrl Pts',(-0.255809694565027,-0.0408389754760835,
-5.9658));
#29357=CARTESIAN_POINT('Ctrl Pts',(-0.258562495027418,-0.0302064884413545,
-5.9658));
#29358=CARTESIAN_POINT('Ctrl Pts',(-0.260635400953148,-0.0194347400518625,
-5.9658));
#29359=CARTESIAN_POINT('Ctrl Pts',(-0.261801443193027,-0.0133754618841457,
-5.9658));
#29360=CARTESIAN_POINT('Ctrl Pts',(-0.262752444669097,-0.00726639468052522,
-5.9658));
#29361=CARTESIAN_POINT('Ctrl Pts',(-0.263478002042444,-0.00115090105513363,
-5.9658));
#29362=CARTESIAN_POINT('Ctrl Pts',(-0.264780382498361,0.0098264518993917,
-5.9658));
#29363=CARTESIAN_POINT('Ctrl Pts',(-0.265361291178618,0.0208402687922307,
-5.9658));
#29364=CARTESIAN_POINT('Ctrl Pts',(-0.265195455964071,0.0318245246133395,
-5.9658));
#29365=CARTESIAN_POINT('Ctrl Pts',(-0.26502005174603,0.0434425926354643,
-5.9658));
#29366=CARTESIAN_POINT('Ctrl Pts',(-0.26400964329553,0.0550278502294863,
-5.9658));
#29367=CARTESIAN_POINT('Ctrl Pts',(-0.262217575180139,0.0665215726485518,
-5.9658));
#29368=CARTESIAN_POINT('Ctrl Pts',(-0.261084137053752,0.0737910637421093,
-5.9658));
#29369=CARTESIAN_POINT('Ctrl Pts',(-0.259637700833268,0.0810240070529162,
-5.9658));
#29370=CARTESIAN_POINT('Ctrl Pts',(-0.257888733163235,0.0882056483398937,
-5.9658));
#29371=CARTESIAN_POINT('Ctrl Pts',(-0.256841146357813,0.0925072673934748,
-5.9658));
#29372=CARTESIAN_POINT('Ctrl Pts',(-0.2556849101705,0.0967898034443975,
-5.9658));
#29373=CARTESIAN_POINT('Ctrl Pts',(-0.254426565527262,0.10103697054799,
-5.9658));
#29374=CARTESIAN_POINT('Ctrl Pts',(-0.249729836042933,0.116889380352809,
-5.9658));
#29375=CARTESIAN_POINT('Ctrl Pts',(-0.243603775465189,0.132296506950611,
-5.9658));
#29376=CARTESIAN_POINT('Ctrl Pts',(-0.236195443982762,0.147098364696853,
-5.9658));
#29377=CARTESIAN_POINT('Ctrl Pts',(-0.229442030401605,0.160591695464646,
-5.9658));
#29378=CARTESIAN_POINT('Ctrl Pts',(-0.221622050217669,0.173582952148739,
-5.9658));
#29379=CARTESIAN_POINT('Ctrl Pts',(-0.212811980334952,0.185945226493148,
-5.9658));
#29380=CARTESIAN_POINT('Ctrl Pts',(-0.210205025895605,0.189603300312268,
-5.9658));
#29381=CARTESIAN_POINT('Ctrl Pts',(-0.207511908992761,0.193204856844324,
-5.9658));
#29382=CARTESIAN_POINT('Ctrl Pts',(-0.204742504452648,0.196736924240536,
-5.9658));
#29383=CARTESIAN_POINT('Ctrl Pts',(-0.193966565401581,0.210480435682992,
-5.9658));
#29384=CARTESIAN_POINT('Ctrl Pts',(-0.182010459766652,0.223214646370377,
-5.9658));
#29385=CARTESIAN_POINT('Ctrl Pts',(-0.169008886945702,0.234760544715186,
-5.9658));
#29386=CARTESIAN_POINT('Ctrl Pts',(-0.156567866754381,0.245808650695352,
-5.9658));
#29387=CARTESIAN_POINT('Ctrl Pts',(-0.143168667892983,0.255769903558261,
-5.9658));
#29388=CARTESIAN_POINT('Ctrl Pts',(-0.128892185405323,0.264462557919717,
-5.9658));
#29389=CARTESIAN_POINT('Ctrl Pts',(-0.138001922973973,-0.193371366051283,
-5.9658));
#29390=CARTESIAN_POINT('Ctrl Pts',(-0.0784315765852419,-0.235399718049311,
-5.96088888094234));
#29391=CARTESIAN_POINT('Ctrl Pts',(0.0890659557212074,-0.262569296818482,
-5.95068256674318));
#29392=CARTESIAN_POINT('Ctrl Pts',(0.270472008799548,-0.0738624404218237,
-5.93518105740252));
#29393=CARTESIAN_POINT('Ctrl Pts',(0.208622919271946,0.187359333710957,
-5.91929547197799));
#29394=CARTESIAN_POINT('Ctrl Pts',(-0.0444078770673998,0.276831260195588,
-5.90340988655351));
#29395=CARTESIAN_POINT('Ctrl Pts',(-0.215288460980913,0.144741092199657,
-5.89062506616399));
#29396=CARTESIAN_POINT('Ctrl Pts',(-0.236965055372185,0.0329209448004622,
-5.88313544091599));
#29397=CARTESIAN_POINT('Ctrl Pts',(-0.23683200269258,0.000108453577955931,
-5.8809410108095));
#29398=CARTESIAN_POINT('Origin',(-3.51939854619125E-17,0.,-5.9658));
#29399=CARTESIAN_POINT('',(-0.2942,-3.60291088309151E-17,-5.9658));
#29400=CARTESIAN_POINT('Origin',(0.,0.,-5.9658));
#29401=CARTESIAN_POINT('Origin',(0.,0.,-5.9658));
#29402=CARTESIAN_POINT('',(0.137702479013101,-0.193106208855765,-5.9658));
#29403=CARTESIAN_POINT('Ctrl Pts',(0.129204211840496,0.264848286765706,
-5.9658));
#29404=CARTESIAN_POINT('Ctrl Pts',(0.135270963946878,0.261191483925809,
-5.9658));
#29405=CARTESIAN_POINT('Ctrl Pts',(0.141186833539423,0.257306043876668,
-5.9658));
#29406=CARTESIAN_POINT('Ctrl Pts',(0.14693706551556,0.253191178187327,-5.9658));
#29407=CARTESIAN_POINT('Ctrl Pts',(0.156778842106654,0.246148403394085,
-5.9658));
#29408=CARTESIAN_POINT('Ctrl Pts',(0.166135974562664,0.23843387751087,-5.9658));
#29409=CARTESIAN_POINT('Ctrl Pts',(0.174974019412259,0.230118978005656,
-5.9658));
#29410=CARTESIAN_POINT('Ctrl Pts',(0.179162346603656,0.22617856807517,-5.9658));
#29411=CARTESIAN_POINT('Ctrl Pts',(0.183233953121907,0.22210322175818,-5.9658));
#29412=CARTESIAN_POINT('Ctrl Pts',(0.187184339205463,0.217900102741158,
-5.9658));
#29413=CARTESIAN_POINT('Ctrl Pts',(0.191295138666803,0.213526307616919,
-5.9658));
#29414=CARTESIAN_POINT('Ctrl Pts',(0.195269648419525,0.20901927500812,-5.9658));
#29415=CARTESIAN_POINT('Ctrl Pts',(0.199098691984892,0.204393903223475,
-5.9658));
#29416=CARTESIAN_POINT('Ctrl Pts',(0.210108605301767,0.191094252399997,
-5.9658));
#29417=CARTESIAN_POINT('Ctrl Pts',(0.219933632950231,0.176802353940203,
-5.9658));
#29418=CARTESIAN_POINT('Ctrl Pts',(0.228454636692493,0.1617197431557,-5.9658));
#29419=CARTESIAN_POINT('Ctrl Pts',(0.231390832132516,0.156522527622341,
-5.9658));
#29420=CARTESIAN_POINT('Ctrl Pts',(0.234172663418191,0.151228725911185,
-5.9658));
#29421=CARTESIAN_POINT('Ctrl Pts',(0.236784343132879,0.145867972582067,
-5.9658));
#29422=CARTESIAN_POINT('Ctrl Pts',(0.244117814256368,0.130815234867661,
-5.9658));
#29423=CARTESIAN_POINT('Ctrl Pts',(0.250133917516935,0.115201848504892,
-5.9658));
#29424=CARTESIAN_POINT('Ctrl Pts',(0.254724799740319,0.0992138111912858,
-5.9658));
#29425=CARTESIAN_POINT('Ctrl Pts',(0.257708789856447,0.0888218771361952,
-5.9658));
#29426=CARTESIAN_POINT('Ctrl Pts',(0.260089689774926,0.0782713310743704,
-5.9658));
#29427=CARTESIAN_POINT('Ctrl Pts',(0.261825733325987,0.0676136941592587,
-5.9658));
#29428=CARTESIAN_POINT('Ctrl Pts',(0.262540428182012,0.0632261554503647,
-5.9658));
#29429=CARTESIAN_POINT('Ctrl Pts',(0.263145713290975,0.0588204915595365,
-5.9658));
#29430=CARTESIAN_POINT('Ctrl Pts',(0.263638159729527,0.0544004451437594,
-5.9658));
#29431=CARTESIAN_POINT('Ctrl Pts',(0.264128588802814,0.0499985059725725,
-5.9658));
#29432=CARTESIAN_POINT('Ctrl Pts',(0.26450604161011,0.0455914489729751,
-5.9658));
#29433=CARTESIAN_POINT('Ctrl Pts',(0.264768243741406,0.0411852375561797,
-5.9658));
#29434=CARTESIAN_POINT('Ctrl Pts',(0.265341350360721,0.031554389337699,
-5.9658));
#29435=CARTESIAN_POINT('Ctrl Pts',(0.265364753733676,0.0219237178920483,
-5.9658));
#29436=CARTESIAN_POINT('Ctrl Pts',(0.26481238867451,0.0123306438726335,
-5.9658));
#29437=CARTESIAN_POINT('Ctrl Pts',(0.263870782204104,-0.00402249146400645,
-5.9658));
#29438=CARTESIAN_POINT('Ctrl Pts',(0.261258313698482,-0.020268305434637,
-5.9658));
#29439=CARTESIAN_POINT('Ctrl Pts',(0.257080958864981,-0.0362025073647849,
-5.9658));
#29440=CARTESIAN_POINT('Ctrl Pts',(0.255996044923037,-0.0403408289861939,
-5.9658));
#29441=CARTESIAN_POINT('Ctrl Pts',(0.254804542204504,-0.0444604395475238,
-5.9658));
#29442=CARTESIAN_POINT('Ctrl Pts',(0.253510491762343,-0.0485491427174342,
-5.9658));
#29443=CARTESIAN_POINT('Ctrl Pts',(0.248734016185539,-0.0636409739131856,
-5.9658));
#29444=CARTESIAN_POINT('Ctrl Pts',(0.242584291373476,-0.078256306454302,
-5.9658));
#29445=CARTESIAN_POINT('Ctrl Pts',(0.235173624314207,-0.0922177548230339,
-5.9658));
#29446=CARTESIAN_POINT('Ctrl Pts',(0.229460014360973,-0.10298200448142,
-5.9658));
#29447=CARTESIAN_POINT('Ctrl Pts',(0.222995632074016,-0.113357386780667,
-5.9658));
#29448=CARTESIAN_POINT('Ctrl Pts',(0.215816926629553,-0.123247361184162,
-5.9658));
#29449=CARTESIAN_POINT('Ctrl Pts',(0.213223159570887,-0.126820747781132,
-5.9658));
#29450=CARTESIAN_POINT('Ctrl Pts',(0.210534760635697,-0.130332183901753,
-5.9658));
#29451=CARTESIAN_POINT('Ctrl Pts',(0.207757243033476,-0.133771505040915,
-5.9658));
#29452=CARTESIAN_POINT('Ctrl Pts',(0.198033824944794,-0.145811737423448,
-5.9658));
#29453=CARTESIAN_POINT('Ctrl Pts',(0.187277114682385,-0.156904076768832,
-5.9658));
#29454=CARTESIAN_POINT('Ctrl Pts',(0.175576038540493,-0.166863573434083,
-5.9658));
#29455=CARTESIAN_POINT('Ctrl Pts',(0.164593283736169,-0.176211663175789,
-5.9658));
#29456=CARTESIAN_POINT('Ctrl Pts',(0.152777422469776,-0.18456226563307,
-5.9658));
#29457=CARTESIAN_POINT('Ctrl Pts',(0.140183547508633,-0.191717677594505,
-5.9658));
#29458=CARTESIAN_POINT('Ctrl Pts',(0.139359851699299,-0.19218567357389,
-5.9658));
#29459=CARTESIAN_POINT('Ctrl Pts',(0.138532824156898,-0.192648538423476,
-5.9658));
#29460=CARTESIAN_POINT('Ctrl Pts',(0.137702479013101,-0.193106208855765,
-5.9658));
#29461=CARTESIAN_POINT('Origin',(0.,0.,-5.9658));
#29462=CARTESIAN_POINT('Origin',(0.,0.,-6.1506589891905));
#29463=CARTESIAN_POINT('Ctrl Pts',(0.137702479013101,-0.193106208855765,
-5.9658));
#29464=CARTESIAN_POINT('Ctrl Pts',(0.201950251596361,-0.147291640757684,
-5.9605048048585));
#29465=CARTESIAN_POINT('Ctrl Pts',(0.279999109649734,0.0127284642187734,
-5.9499144145755));
#29466=CARTESIAN_POINT('Ctrl Pts',(0.140787666388597,0.242681034292982,
-5.93402882915098));
#29467=CARTESIAN_POINT('Ctrl Pts',(-0.127558649843965,0.249601560230261,
-5.91814324372648));
#29468=CARTESIAN_POINT('Ctrl Pts',(-0.233570227134833,0.0945490249099159,
-5.90701996373965));
#29469=CARTESIAN_POINT('Ctrl Pts',(-0.237519260455749,0.00806361963123399,
-5.90119187889433));
#29470=CARTESIAN_POINT('Ctrl Pts',(-0.237465179907043,0.000150546841787677,
-5.9006589891905));
#29471=CARTESIAN_POINT('Ctrl Pts',(0.170810875200398,-0.239535560853235,
-5.99872339910054));
#29472=CARTESIAN_POINT('Ctrl Pts',(0.250506014629069,-0.182705600130328,
-5.99342820395904));
#29473=CARTESIAN_POINT('Ctrl Pts',(0.347320493555188,0.0157888233294544,
-5.98283781367603));
#29474=CARTESIAN_POINT('Ctrl Pts',(0.174637847376516,0.301029873675537,
-5.96695222825153));
#29475=CARTESIAN_POINT('Ctrl Pts',(-0.158228121783892,0.309614331273291,
-5.95106664282702));
#29476=CARTESIAN_POINT('Ctrl Pts',(-0.346028909939958,0.0349368943093817,
-5.93518105740251));
#29477=CARTESIAN_POINT('Ctrl Pts',(-0.216833251566021,-0.271965029219739,
-5.919295471978));
#29478=CARTESIAN_POINT('Ctrl Pts',(0.111056996638582,-0.329572597154436,
-5.9034098865535));
#29479=CARTESIAN_POINT('Ctrl Pts',(0.337180324851565,-0.0852715125928928,
-5.88752430112899));
#29480=CARTESIAN_POINT('Ctrl Pts',(0.25437389699959,0.237187870968243,-5.87163871570449));
#29481=CARTESIAN_POINT('Ctrl Pts',(-0.0615020985666884,0.342312200380475,
-5.85575313027997));
#29482=CARTESIAN_POINT('Ctrl Pts',(-0.321025987744245,0.133806145032197,
-5.83986754485548));
#29483=CARTESIAN_POINT('Ctrl Pts',(-0.286415645896083,-0.197301835163802,
-5.82398195943096));
#29484=CARTESIAN_POINT('Ctrl Pts',(0.0106191074128067,-0.347632915551424,
-5.80809637400646));
#29485=CARTESIAN_POINT('Ctrl Pts',(0.297924023820578,-0.179451765614445,
-5.79221078858195));
#29486=CARTESIAN_POINT('Ctrl Pts',(0.312260748456384,0.153149879487187,
-5.77632520315744));
#29487=CARTESIAN_POINT('Ctrl Pts',(0.0404932868106416,0.345430002986954,
-5.76043961773294));
#29488=CARTESIAN_POINT('Ctrl Pts',(-0.26837549419498,0.221215336287527,
-5.74455403230843));
#29489=CARTESIAN_POINT('Ctrl Pts',(-0.331349362349014,-0.105684567869114,
-5.72866844688393));
#29490=CARTESIAN_POINT('Ctrl Pts',(-0.0907294504682248,-0.335752567049075,
-5.71278286145941));
#29491=CARTESIAN_POINT('Ctrl Pts',(0.233019924150162,-0.258192447446947,
-5.69689727603491));
#29492=CARTESIAN_POINT('Ctrl Pts',(0.343268369714444,0.0559325528732654,
-5.6810116906104));
#29493=CARTESIAN_POINT('Ctrl Pts',(0.139002435305783,0.318810203883323,
-5.66512610518591));
#29494=CARTESIAN_POINT('Ctrl Pts',(-0.192622347799029,0.289582898383506,
-5.64924051976138));
#29495=CARTESIAN_POINT('Ctrl Pts',(-0.347759859492789,-0.00497029766718102,
-5.63335493433689));
#29496=CARTESIAN_POINT('Ctrl Pts',(-0.184267733667245,-0.294969533934804,
-5.61746934891237));
#29497=CARTESIAN_POINT('Ctrl Pts',(0.148056876757647,-0.314707459357535,
-5.60158376348787));
#29498=CARTESIAN_POINT('Ctrl Pts',(0.344726644784264,-0.0460995018935765,
-5.58569817806336));
#29499=CARTESIAN_POINT('Ctrl Pts',(0.225545911893637,0.264746417001876,
-5.56981259263886));
#29500=CARTESIAN_POINT('Ctrl Pts',(-0.100287803351684,0.333022492034977,
-5.55392700721435));
#29501=CARTESIAN_POINT('Ctrl Pts',(-0.334234356988874,0.0961718165849793,
-5.53804142178984));
#29502=CARTESIAN_POINT('Ctrl Pts',(-0.261943807492036,-0.228794810720281,
-5.52215583636533));
#29503=CARTESIAN_POINT('Ctrl Pts',(0.0503487379441082,-0.344131701947668,
-5.50627025094083));
#29504=CARTESIAN_POINT('Ctrl Pts',(0.31651002448484,-0.144163199526538,
-5.49038466551631));
#29505=CARTESIAN_POINT('Ctrl Pts',(0.292673855696793,0.187892623294873,
-5.47449908009182));
#29506=CARTESIAN_POINT('Ctrl Pts',(0.000679755635424282,0.347794711905736,
-5.4586134946673));
#29507=CARTESIAN_POINT('Ctrl Pts',(-0.291937160100985,0.18903523018041,
-5.4427279092428));
#29508=CARTESIAN_POINT('Ctrl Pts',(-0.317071130604053,-0.142924881789908,
-5.42684232381829));
#29509=CARTESIAN_POINT('Ctrl Pts',(-0.0516935409033043,-0.343932262990989,
-5.41095673839378));
#29510=CARTESIAN_POINT('Ctrl Pts',(0.26104746277864,-0.229816983432556,
-5.39507115296928));
#29511=CARTESIAN_POINT('Ctrl Pts',(0.334607732615142,0.0948645822810613,
-5.37918556754477));
#29512=CARTESIAN_POINT('Ctrl Pts',(0.101588799630167,0.332627929505195,
-5.36329998212027));
#29513=CARTESIAN_POINT('Ctrl Pts',(-0.224509312854917,0.26562603814126,
-5.34741439669575));
#29514=CARTESIAN_POINT('Ctrl Pts',(-0.3449042109429,-0.0447516365182755,
-5.33152881127126));
#29515=CARTESIAN_POINT('Ctrl Pts',(-0.14928591586817,-0.314126310615031,
-5.31564322584674));
#29516=CARTESIAN_POINT('Ctrl Pts',(0.18311330988511,-0.295687570655462,
-5.29975764042224));
#29517=CARTESIAN_POINT('Ctrl Pts',(0.347737774033734,-0.00632962931557787,
-5.28387205499772));
#29518=CARTESIAN_POINT('Ctrl Pts',(0.193752836298635,0.288827737801347,
-5.26798646957323));
#29519=CARTESIAN_POINT('Ctrl Pts',(-0.137755165929293,0.319351120174961,
-5.25210088414871));
#29520=CARTESIAN_POINT('Ctrl Pts',(-0.343047110252429,0.057273936870683,
-5.23621529872421));
#29521=CARTESIAN_POINT('Ctrl Pts',(-0.23402740143643,-0.257279612628208,
-5.2203297132997));
#29522=CARTESIAN_POINT('Ctrl Pts',(0.0894163244517817,-0.336104663191011,
-5.2044441278752));
#29523=CARTESIAN_POINT('Ctrl Pts',(0.330933714521616,-0.106978971251994,
-5.18855854245068));
#29524=CARTESIAN_POINT('Ctrl Pts',(0.269238164496358,0.220164562261598,
-5.17267295702619));
#29525=CARTESIAN_POINT('Ctrl Pts',(-0.0391427241948519,0.345585692469776,
-5.15678737160167));
#29526=CARTESIAN_POINT('Ctrl Pts',(-0.31165969221056,0.15436923251875,-5.14090178617716));
#29527=CARTESIAN_POINT('Ctrl Pts',(-0.298623247450242,-0.178285669024407,
-5.12501620075266));
#29528=CARTESIAN_POINT('Ctrl Pts',(-0.0119778324735712,-0.347589060855552,
-5.10913061532816));
#29529=CARTESIAN_POINT('Ctrl Pts',(0.285642087791955,-0.198419306971529,
-5.09324502990364));
#29530=CARTESIAN_POINT('Ctrl Pts',(0.321546826274025,0.132549093585398,
-5.07735944447914));
#29531=CARTESIAN_POINT('Ctrl Pts',(0.0628392170425058,0.342071420172299,
-5.06147385905463));
#29532=CARTESIAN_POINT('Ctrl Pts',(-0.253443860981231,0.238176054690927,
-5.04558827363013));
#29533=CARTESIAN_POINT('Ctrl Pts',(-0.337512888682964,-0.0839444677753746,
-5.02970268820562));
#29534=CARTESIAN_POINT('Ctrl Pts',(-0.112340908875126,-0.329152159176147,
-5.01381710278111));
#29535=CARTESIAN_POINT('Ctrl Pts',(0.215761705613502,-0.272779233241759,
-4.99793151735661));
#29536=CARTESIAN_POINT('Ctrl Pts',(0.346175966669865,0.0335234812839203,
-4.9820459319321));
#29537=CARTESIAN_POINT('Ctrl Pts',(0.159411807884773,0.309110820263732,
-4.9661603465076));
#29538=CARTESIAN_POINT('Ctrl Pts',(-0.173410974828944,0.301480111294401,
-4.95027476108308));
#29539=CARTESIAN_POINT('Ctrl Pts',(-0.347348611619563,0.0176228744298602,
-4.93438917565858));
#29540=CARTESIAN_POINT('Ctrl Pts',(-0.203033410619501,-0.282381050832776,
-4.91850359023406));
#29541=CARTESIAN_POINT('Ctrl Pts',(0.127308038750163,-0.323657669408275,
-4.90261800480957));
#29542=CARTESIAN_POINT('Ctrl Pts',(0.341005450255696,-0.0683879126243729,
-4.88673241938505));
#29543=CARTESIAN_POINT('Ctrl Pts',(0.24226184827928,0.249541220173173,-4.87084683396055));
#29544=CARTESIAN_POINT('Ctrl Pts',(-0.0784504563898112,0.3388320374307,
-4.85496124853604));
#29545=CARTESIAN_POINT('Ctrl Pts',(-0.327283733658682,0.117673197371545,
-4.83907566311153));
#29546=CARTESIAN_POINT('Ctrl Pts',(-0.276248309815004,-0.211301904917024,
-4.82319007768704));
#29547=CARTESIAN_POINT('Ctrl Pts',(0.0278953908217769,-0.346674877757401,
-4.80730449226252));
#29548=CARTESIAN_POINT('Ctrl Pts',(0.306480367475419,-0.164412311124628,
-4.79141890683802));
#29549=CARTESIAN_POINT('Ctrl Pts',(0.304257408201531,0.168490513832963,
-4.77553332141351));
#29550=CARTESIAN_POINT('Ctrl Pts',(0.0232632653392378,0.347016489785378,
-4.759647735989));
#29551=CARTESIAN_POINT('Ctrl Pts',(-0.279045487579995,0.207593929483624,
-4.7437621505645));
#29552=CARTESIAN_POINT('Ctrl Pts',(-0.325683092481844,-0.122033384648102,
-4.72787656513998));
#29553=CARTESIAN_POINT('Ctrl Pts',(-0.0739185591989158,-0.339849481834481,
-4.71199097971549));
#29554=CARTESIAN_POINT('Ctrl Pts',(0.24557272019296,-0.246283703874696,
-4.69610539429097));
#29555=CARTESIAN_POINT('Ctrl Pts',(0.340061761283145,0.072935740280159,
-4.68021980886648));
#29556=CARTESIAN_POINT('Ctrl Pts',(0.122974429438251,0.325328931085979,
-4.66433422344196));
#29557=CARTESIAN_POINT('Ctrl Pts',(-0.206786337207292,0.279644478653881,
-4.64844863801746));
#29558=CARTESIAN_POINT('Ctrl Pts',(-0.347082294059265,-0.0222599381797678,
-4.63256305259294));
#29559=CARTESIAN_POINT('Ctrl Pts',(-0.169369422500422,-0.303769028077391,
-4.61667746716844));
#29560=CARTESIAN_POINT('Ctrl Pts',(0.163525584649523,-0.306954405184615,
-4.60079188174393));
#29561=CARTESIAN_POINT('Ctrl Pts',(0.346592783006926,-0.0288975165840105,
-4.58490629631943));
#29562=CARTESIAN_POINT('Ctrl Pts',(0.212099659947135,0.275636278358852,
-4.56902071089492));
#29563=CARTESIAN_POINT('Ctrl Pts',(-0.116726523371279,0.32762256094302,
-4.55313512547042));
#29564=CARTESIAN_POINT('Ctrl Pts',(-0.338603819993014,0.0794296971122733,
-4.5372495400459));
#29565=CARTESIAN_POINT('Ctrl Pts',(-0.250240560024966,-0.241539408411135,
-4.5213639546214));
#29566=CARTESIAN_POINT('Ctrl Pts',(0.0674017748958896,-0.341201735690329,
-4.50547836919689));
#29567=CARTESIAN_POINT('Ctrl Pts',(0.323288267371518,-0.128243205968701,
-4.48959278377238));
#29568=CARTESIAN_POINT('Ctrl Pts',(0.282966843438066,0.20221619423752,-4.47370719834787));
#29569=CARTESIAN_POINT('Ctrl Pts',(-0.0166186106722786,0.34739810804973,
-4.45782161292338));
#29570=CARTESIAN_POINT('Ctrl Pts',(-0.300977517649094,0.174281833726291,
-4.44193602749886));
#29571=CARTESIAN_POINT('Ctrl Pts',(-0.30957039044947,-0.158517497627776,
-4.42605044207436));
#29572=CARTESIAN_POINT('Ctrl Pts',(-0.0345241411668705,-0.34607760310933,
-4.41016485664984));
#29573=CARTESIAN_POINT('Ctrl Pts',(0.272154322931305,-0.216549412853076,
-4.39427927122535));
#29574=CARTESIAN_POINT('Ctrl Pts',(0.329475562925319,0.111388855511911,
-4.37839368580083));
#29575=CARTESIAN_POINT('Ctrl Pts',(0.0849198718593337,0.337268793487633,
-4.36250810037633));
#29576=CARTESIAN_POINT('Ctrl Pts',(-0.237442349303437,0.254131372432594,
-4.34662251495183));
#29577=CARTESIAN_POINT('Ctrl Pts',(-0.34225165978905,-0.0618500207667643,
-4.33073692952732));
#29578=CARTESIAN_POINT('Ctrl Pts',(-0.133478136422044,-0.321162281089338,
-4.31485134410281));
#29579=CARTESIAN_POINT('Ctrl Pts',(0.19759268216448,-0.286214527325668,
-4.2989657586783));
#29580=CARTESIAN_POINT('Ctrl Pts',(0.347622236378851,0.0109728971641897,
-4.28308017325379));
#29581=CARTESIAN_POINT('Ctrl Pts',(0.179148248313675,0.298106572928794,
-4.26719458782929));
#29582=CARTESIAN_POINT('Ctrl Pts',(-0.15346757450713,0.312104673582609,
-4.25130900240478));
#29583=CARTESIAN_POINT('Ctrl Pts',(-0.345471086059395,0.0401416541033478,
-4.23542341698027));
#29584=CARTESIAN_POINT('Ctrl Pts',(-0.220942013818134,-0.268600540258568,
-4.21953783155577));
#29585=CARTESIAN_POINT('Ctrl Pts',(0.106021789792706,-0.331241609382573,
-4.20365224613125));
#29586=CARTESIAN_POINT('Ctrl Pts',(0.335844754659909,-0.0903876344676083,
-4.18776666070676));
#29587=CARTESIAN_POINT('Ctrl Pts',(0.257955114230381,0.233282624169873,
-4.17188107528224));
#29588=CARTESIAN_POINT('Ctrl Pts',(-0.0562819431172887,0.34321125648226,
-4.15599548985774));
#29589=CARTESIAN_POINT('Ctrl Pts',(-0.318951533332058,0.138677839190145,
-4.14010990443324));
#29590=CARTESIAN_POINT('Ctrl Pts',(-0.289386673184354,-0.192917021230238,
-4.12422431900872));
#29591=CARTESIAN_POINT('Ctrl Pts',(0.00532428767735682,-0.347754619894331,
-4.10833873358422));
#29592=CARTESIAN_POINT('Ctrl Pts',(0.295156951620275,-0.183967381913722,
-4.09245314815971));
#29593=CARTESIAN_POINT('Ctrl Pts',(0.314556585731257,0.14837714806886,-4.07656756273521));
#29594=CARTESIAN_POINT('Ctrl Pts',(0.0457485728179687,0.344773391928874,
-4.0606819773107));
#29595=CARTESIAN_POINT('Ctrl Pts',(-0.264975868266788,0.225276303544235,
-4.04479639188619));
#29596=CARTESIAN_POINT('Ctrl Pts',(-0.33292023420213,-0.10062674269826,
-4.02891080646169));
#29597=CARTESIAN_POINT('Ctrl Pts',(-0.0958315419103227,-0.334332079337508,
-4.01302522103718));
#29598=CARTESIAN_POINT('Ctrl Pts',(0.229061330908633,-0.261710776264314,
-3.99713963561267));
#29599=CARTESIAN_POINT('Ctrl Pts',(0.344080272397588,0.0506990115029886,
-3.98125405018816));
#29600=CARTESIAN_POINT('Ctrl Pts',(0.143840942183751,0.316656607518357,
-3.96536846476366));
#29601=CARTESIAN_POINT('Ctrl Pts',(-0.188190445868226,0.292482443903425,
-3.94948287933915));
#29602=CARTESIAN_POINT('Ctrl Pts',(-0.347795222829602,0.000325726836706584,
-3.93359729391464));
#29603=CARTESIAN_POINT('Ctrl Pts',(-0.188737964255785,-0.292129431872098,
-3.91771170849014));
#29604=CARTESIAN_POINT('Ctrl Pts',(0.143247564876018,-0.316925480399863,
-3.90182612306563));
#29605=CARTESIAN_POINT('Ctrl Pts',(0.343984698876466,-0.0513434163372087,
-3.88594053764113));
#29606=CARTESIAN_POINT('Ctrl Pts',(0.229551149674784,0.261281261283245,
-3.87005495221662));
#29607=CARTESIAN_POINT('Ctrl Pts',(-0.0952051604262189,0.334510998804856,
-3.85416936679211));
#29608=CARTESIAN_POINT('Ctrl Pts',(-0.332731123583902,0.101250148833917,
-3.83828378136761));
#29609=CARTESIAN_POINT('Ctrl Pts',(-0.265397450764868,-0.224779567000631,
-3.8223981959431));
#29610=CARTESIAN_POINT('Ctrl Pts',(0.045102860632521,-0.344858510282622,
-3.80651261051859));
#29611=CARTESIAN_POINT('Ctrl Pts',(0.31427779764301,-0.14896602070837,-3.79062702509408));
#29612=CARTESIAN_POINT('Ctrl Pts',(0.295501624885664,0.18341408360049,-3.77474143966957));
#29613=CARTESIAN_POINT('Ctrl Pts',(0.00597449078588094,0.347744266258115,
-3.75885585424507));
#29614=CARTESIAN_POINT('Ctrl Pts',(-0.289022562023056,0.19345828826664,
-3.74297026882056));
#29615=CARTESIAN_POINT('Ctrl Pts',(-0.319215082650408,-0.138079312779645,
-3.72708468339606));
#29616=CARTESIAN_POINT('Ctrl Pts',(-0.0569162995882634,-0.343106888837962,
-3.71119909797154));
#29617=CARTESIAN_POINT('Ctrl Pts',(0.257501441669556,-0.233762188635379,
-3.69531351254704));
#29618=CARTESIAN_POINT('Ctrl Pts',(0.336044900769636,0.0897522187464598,
-3.67942792712253));
#29619=CARTESIAN_POINT('Ctrl Pts',(0.10658126864456,0.33105441587802,-3.66354234169803));
#29620=CARTESIAN_POINT('Ctrl Pts',(-0.220320727040801,0.268990613013312,
-3.64765675627352));
#29621=CARTESIAN_POINT('Ctrl Pts',(-0.345776258125757,-0.0394479644336986,
-3.63177117084901));
#29622=CARTESIAN_POINT('Ctrl Pts',(-0.153577823762402,-0.311920926252076,
-3.61588558542451));
#29623=CARTESIAN_POINT('Ctrl Pts',(0.0670764293281557,-0.302713317039253,
-3.6052951951415));
#29624=CARTESIAN_POINT('Ctrl Pts',(0.151068846355364,-0.252451665989471,
-3.6));
#29625=CARTESIAN_POINT('Ctrl Pts',(0.159774743137966,-0.224059110187412,
-5.98774893273369));
#29626=CARTESIAN_POINT('Ctrl Pts',(0.234320760284833,-0.170900947006113,
-5.98245373759219));
#29627=CARTESIAN_POINT('Ctrl Pts',(0.32488003225337,0.0147687036258942,
-5.97186334730919));
#29628=CARTESIAN_POINT('Ctrl Pts',(0.163354453713877,0.281580260548018,
-5.95597776188468));
#29629=CARTESIAN_POINT('Ctrl Pts',(-0.148004964470583,0.289610074258948,
-5.94009217646017));
#29630=CARTESIAN_POINT('Ctrl Pts',(-0.323671898168684,0.0326796130970632,
-5.92420659103566));
#29631=CARTESIAN_POINT('Ctrl Pts',(-0.20282360260777,-0.25439330273973,
-5.90832100561116));
#29632=CARTESIAN_POINT('Ctrl Pts',(0.103881577158279,-0.308278831742322,
-5.89243542018665));
#29633=CARTESIAN_POINT('Ctrl Pts',(0.315395022308329,-0.0797620994888713,
-5.87654983476214));
#29634=CARTESIAN_POINT('Ctrl Pts',(0.237938737837567,0.221863105115123,
-5.86066424933764));
#29635=CARTESIAN_POINT('Ctrl Pts',(-0.057528433066161,0.320195326115013,
-5.84477866391313));
#29636=CARTESIAN_POINT('Ctrl Pts',(-0.30028442083838,0.125160897558301,
-5.82889307848862));
#29637=CARTESIAN_POINT('Ctrl Pts',(-0.267910261568841,-0.184554115754993,
-5.81300749306412));
#29638=CARTESIAN_POINT('Ctrl Pts',(0.00993300430809844,-0.325172268588677,
-5.7971219076396));
#29639=CARTESIAN_POINT('Ctrl Pts',(0.27867508040525,-0.167857343527245,
-5.78123632221511));
#29640=CARTESIAN_POINT('Ctrl Pts',(0.292085505786177,0.143254828639967,
-5.76535073679059));
#29641=CARTESIAN_POINT('Ctrl Pts',(0.0378770057315835,0.323111686739128,
-5.74946515136609));
#29642=CARTESIAN_POINT('Ctrl Pts',(-0.251035688443259,0.206922559772916,
-5.73357956594158));
#29643=CARTESIAN_POINT('Ctrl Pts',(-0.309940799706874,-0.0988562623142354,
-5.71769398051708));
#29644=CARTESIAN_POINT('Ctrl Pts',(-0.0848673986747166,-0.314059512283639,
-5.70180839509257));
#29645=CARTESIAN_POINT('Ctrl Pts',(0.217964450351541,-0.241510570814654,
-5.68592280966806));
#29646=CARTESIAN_POINT('Ctrl Pts',(0.321089717116476,0.0523187370704123,
-5.67003722424356));
#29647=CARTESIAN_POINT('Ctrl Pts',(0.13002145425739,0.298211799309964,-5.65415163881905));
#29648=CARTESIAN_POINT('Ctrl Pts',(-0.180176971203471,0.270872877105102,
-5.63826605339454));
#29649=CARTESIAN_POINT('Ctrl Pts',(-0.325291010651212,-0.00464916552977893,
-5.62238046797003));
#29650=CARTESIAN_POINT('Ctrl Pts',(-0.172362150716446,-0.275911480827357,
-5.60649488254553));
#29651=CARTESIAN_POINT('Ctrl Pts',(0.138490886051659,-0.294374134102762,
-5.59060929712103));
#29652=CARTESIAN_POINT('Ctrl Pts',(0.322453772680454,-0.0431210018986964,
-5.5747237116965));
#29653=CARTESIAN_POINT('Ctrl Pts',(0.2109733358391,0.247641086807527,-5.55883812627201));
#29654=CARTESIAN_POINT('Ctrl Pts',(-0.0938081840608051,0.311505828078151,
-5.54295254084749));
#29655=CARTESIAN_POINT('Ctrl Pts',(-0.312639394143541,0.0899581321970818,
-5.527066955423));
#29656=CARTESIAN_POINT('Ctrl Pts',(-0.245019554577654,-0.214012322524808,
-5.51118136999848));
#29657=CARTESIAN_POINT('Ctrl Pts',(0.04709569377771,-0.321897269244784,
-5.49529578457399));
#29658=CARTESIAN_POINT('Ctrl Pts',(0.296060235060131,-0.134848780250535,
-5.47941019914947));
#29659=CARTESIAN_POINT('Ctrl Pts',(0.273764126916927,0.175752835346323,
-5.46352461372497));
#29660=CARTESIAN_POINT('Ctrl Pts',(0.000635836459002592,0.325323611241308,
-5.44763902830045));
#29661=CARTESIAN_POINT('Ctrl Pts',(-0.273075029402188,0.176821618123943,
-5.43175344287596));
#29662=CARTESIAN_POINT('Ctrl Pts',(-0.296585087976933,-0.133690470523117,
-5.41586785745144));
#29663=CARTESIAN_POINT('Ctrl Pts',(-0.0483536086916446,-0.321710716087453,
-5.39998227202694));
#29664=CARTESIAN_POINT('Ctrl Pts',(0.244181122913523,-0.214968452410302,
-5.38409668660243));
#29665=CARTESIAN_POINT('Ctrl Pts',(0.312988645880066,0.0887353586184989,
-5.36821110117792));
#29666=CARTESIAN_POINT('Ctrl Pts',(0.0950251226542888,0.311136758329086,
-5.35232551575342));
#29667=CARTESIAN_POINT('Ctrl Pts',(-0.210003711715611,0.248463875411818,
-5.33643993032891));
#29668=CARTESIAN_POINT('Ctrl Pts',(-0.322619866246528,-0.0418602224321043,
-5.3205543449044));
#29669=CARTESIAN_POINT('Ctrl Pts',(-0.139640516647252,-0.293830533521418,
-5.3046687594799));
#29670=CARTESIAN_POINT('Ctrl Pts',(0.171282314534783,-0.276583125021395,
-5.28878317405539));
#29671=CARTESIAN_POINT('Ctrl Pts',(0.325270352139021,-0.00592067043078219,
-5.27289758863089));
#29672=CARTESIAN_POINT('Ctrl Pts',(0.181234418567013,0.270166507631257,
-5.25701200320637));
#29673=CARTESIAN_POINT('Ctrl Pts',(-0.128854771257734,0.298717766868846,
-5.24112641778187));
#29674=CARTESIAN_POINT('Ctrl Pts',(-0.32088275328195,0.0535734539225178,
-5.22524083235736));
#29675=CARTESIAN_POINT('Ctrl Pts',(-0.218906834286065,-0.240656714474884,
-5.20935524693286));
#29676=CARTESIAN_POINT('Ctrl Pts',(0.0836391140485833,-0.314388859408473,
-5.19346966150835));
#29677=CARTESIAN_POINT('Ctrl Pts',(0.309552006986385,-0.100067033980699,
-5.17758407608384));
#29678=CARTESIAN_POINT('Ctrl Pts',(0.251842621407298,0.205939676511578,
-5.16169849065934));
#29679=CARTESIAN_POINT('Ctrl Pts',(-0.0366137032938643,0.323257317086716,
-5.14581290523483));
#29680=CARTESIAN_POINT('Ctrl Pts',(-0.29152328393013,0.14439539897651,-5.12992731981032));
#29681=CARTESIAN_POINT('Ctrl Pts',(-0.279329127026664,-0.166766588720627,
-5.11404173438582));
#29682=CARTESIAN_POINT('Ctrl Pts',(-0.0112039418132435,-0.325131247355339,
-5.09815614896131));
#29683=CARTESIAN_POINT('Ctrl Pts',(0.267186683241381,-0.185599387438274,
-5.0822705635368));
#29684=CARTESIAN_POINT('Ctrl Pts',(0.300771607864467,0.123985064510271,
-5.0663849781123));
#29685=CARTESIAN_POINT('Ctrl Pts',(0.0587791599930511,0.319970102774469,
-5.05049939268778));
#29686=CARTESIAN_POINT('Ctrl Pts',(-0.237068791671855,0.222787442047884,
-5.03461380726328));
#29687=CARTESIAN_POINT('Ctrl Pts',(-0.315706099109945,-0.0785207953587747,
-5.01872822183877));
#29688=CARTESIAN_POINT('Ctrl Pts',(-0.105082535513916,-0.307885558363752,
-5.00284263641427));
#29689=CARTESIAN_POINT('Ctrl Pts',(0.201821289499056,-0.255154900842471,
-4.98695705098976));
#29690=CARTESIAN_POINT('Ctrl Pts',(0.323809453527616,0.0313575210298802,
-4.97107146556525));
#29691=CARTESIAN_POINT('Ctrl Pts',(0.149112172325483,0.2891390952178,-4.95518588014075));
#29692=CARTESIAN_POINT('Ctrl Pts',(-0.162206849699077,0.282001408205161,
-4.93930029471624));
#29693=CARTESIAN_POINT('Ctrl Pts',(-0.324906333602788,0.016484256240009,
-4.92341470929174));
#29694=CARTESIAN_POINT('Ctrl Pts',(-0.189915372730789,-0.264136342670823,
-4.90752912386722));
#29695=CARTESIAN_POINT('Ctrl Pts',(0.119082635498715,-0.302746068912006,
-4.89164353844272));
#29696=CARTESIAN_POINT('Ctrl Pts',(0.318973005432638,-0.0639693530080066,
-4.87575795301821));
#29697=CARTESIAN_POINT('Ctrl Pts',(0.22660925152183,0.233418301432662,-4.8598723675937));
#29698=CARTESIAN_POINT('Ctrl Pts',(-0.0733817533809408,0.316940017337243,
-4.8439867821692));
#29699=CARTESIAN_POINT('Ctrl Pts',(-0.306137852271999,0.110070303557685,
-4.82810119674469));
#29700=CARTESIAN_POINT('Ctrl Pts',(-0.258399839537187,-0.197649637606924,
-4.81221561132018));
#29701=CARTESIAN_POINT('Ctrl Pts',(0.0260930628571135,-0.324276129848818,
-4.79633002589568));
#29702=CARTESIAN_POINT('Ctrl Pts',(0.286678596621933,-0.153789591838562,
-4.78044444047117));
#29703=CARTESIAN_POINT('Ctrl Pts',(0.284599263285723,0.157604300881088,
-4.76455885504666));
#29704=CARTESIAN_POINT('Ctrl Pts',(0.0217602201251315,0.324595670240839,
-4.74867326962215));
#29705=CARTESIAN_POINT('Ctrl Pts',(-0.261016290968563,0.194181235365333,
-4.73278768419765));
#29706=CARTESIAN_POINT('Ctrl Pts',(-0.304640628909697,-0.11414877807711,
-4.71690209877314));
#29707=CARTESIAN_POINT('Ctrl Pts',(-0.0691426631663777,-0.3178917244114,
-4.70101651334863));
#29708=CARTESIAN_POINT('Ctrl Pts',(0.229706207198394,-0.230371254052065,
-4.68513092792413));
#29709=CARTESIAN_POINT('Ctrl Pts',(0.318090288433415,0.0682233444162613,
-4.66924534249962));
#29710=CARTESIAN_POINT('Ctrl Pts',(0.115029021735197,0.30430934996749,-4.65335975707511));
#29711=CARTESIAN_POINT('Ctrl Pts',(-0.193425821821788,0.261576581083932,
-4.63747417165061));
#29712=CARTESIAN_POINT('Ctrl Pts',(-0.324657222884633,-0.0208217181767073,
-4.6215885862261));
#29713=CARTESIAN_POINT('Ctrl Pts',(-0.158426423046438,-0.284142437519818,
-4.6057030008016));
#29714=CARTESIAN_POINT('Ctrl Pts',(0.152960156976014,-0.287122006639801,
-4.58981741537708));
#29715=CARTESIAN_POINT('Ctrl Pts',(0.324199339260075,-0.0270304410308685,
-4.57393182995258));
#29716=CARTESIAN_POINT('Ctrl Pts',(0.198395849491113,0.257827351581814,
-4.55804624452807));
#29717=CARTESIAN_POINT('Ctrl Pts',(-0.109184794394113,0.306454787843342,
-4.54216065910356));
#29718=CARTESIAN_POINT('Ctrl Pts',(-0.31672654508354,0.0742977251228926,
-4.52627507367906));
#29719=CARTESIAN_POINT('Ctrl Pts',(-0.234072456767065,-0.225933488668732,
-4.51038948825454));
#29720=CARTESIAN_POINT('Ctrl Pts',(0.0630469298772648,-0.319156608817747,
-4.49450390283005));
#29721=CARTESIAN_POINT('Ctrl Pts',(0.302400534030411,-0.119957381336518,
-4.47861831740553));
#29722=CARTESIAN_POINT('Ctrl Pts',(0.264684287073851,0.189150956897394,
-4.46273273198104));
#29723=CARTESIAN_POINT('Ctrl Pts',(-0.0155448782073034,0.324952632056601,
-4.44684714655652));
#29724=CARTESIAN_POINT('Ctrl Pts',(-0.281531287257139,0.163021442191914,
-4.43096156113202));
#29725=CARTESIAN_POINT('Ctrl Pts',(-0.289568972462407,-0.14827564367103,
-4.41507597570751));
#29726=CARTESIAN_POINT('Ctrl Pts',(-0.0322935280351681,-0.323717445260577,
-4.399190390283));
#29727=CARTESIAN_POINT('Ctrl Pts',(0.254570366138695,-0.202558102782889,
-4.3833048048585));
#29728=CARTESIAN_POINT('Ctrl Pts',(0.308188066918276,0.104191994549338,
-4.36741921943399));
#29729=CARTESIAN_POINT('Ctrl Pts',(0.0794331783483678,0.31547777496437,
-4.35153363400948));
#29730=CARTESIAN_POINT('Ctrl Pts',(-0.222101141543377,0.237711882841648,
-4.33564804858498));
#29731=CARTESIAN_POINT('Ctrl Pts',(-0.320138697065879,-0.0578538759285308,
-4.31976246316047));
#29732=CARTESIAN_POINT('Ctrl Pts',(-0.12485408166398,-0.300411908237402,
-4.30387687773596));
#29733=CARTESIAN_POINT('Ctrl Pts',(0.184826171060436,-0.267722137318025,
-4.28799129231145));
#29734=CARTESIAN_POINT('Ctrl Pts',(0.325162279400034,0.0102639356178628,
-4.27210570688695));
#29735=CARTESIAN_POINT('Ctrl Pts',(0.167573436552869,0.278845834971323,
-4.25622012146245));
#29736=CARTESIAN_POINT('Ctrl Pts',(-0.143551997307641,0.291939514947838,
-4.24033453603793));
#29737=CARTESIAN_POINT('Ctrl Pts',(-0.323150115424298,0.0375480920987667,
-4.22444895061343));
#29738=CARTESIAN_POINT('Ctrl Pts',(-0.206666896734541,-0.251246194226113,
-4.20856336518893));
#29739=CARTESIAN_POINT('Ctrl Pts',(0.0991716962475789,-0.309840008685721,
-4.19267777976441));
#29740=CARTESIAN_POINT('Ctrl Pts',(0.314145743630585,-0.0845476674887783,
-4.17679219433991));
#29741=CARTESIAN_POINT('Ctrl Pts',(0.241288571754755,0.218210177259282,
-4.16090660891539));
#29742=CARTESIAN_POINT('Ctrl Pts',(-0.0526455531260544,0.321036293984072,
-4.1450210234909));
#29743=CARTESIAN_POINT('Ctrl Pts',(-0.298343997428749,0.129717830375486,
-4.12913543806638));
#29744=CARTESIAN_POINT('Ctrl Pts',(-0.270689330063645,-0.180452605712841,
-4.11324985264189));
#29745=CARTESIAN_POINT('Ctrl Pts',(0.00498028415956703,-0.32528610958448,
-4.09736426721737));
#29746=CARTESIAN_POINT('Ctrl Pts',(0.276086789410728,-0.172081204762544,
-4.08147868179287));
#29747=CARTESIAN_POINT('Ctrl Pts',(0.294233008458059,0.138790464555801,
-4.06559309636836));
#29748=CARTESIAN_POINT('Ctrl Pts',(0.0427927464357516,0.322497499480716,
-4.04970751094385));
#29749=CARTESIAN_POINT('Ctrl Pts',(-0.247855713170579,0.210721146950524,
-4.03382192551934));
#29750=CARTESIAN_POINT('Ctrl Pts',(-0.311410177148678,-0.0941252244540177,
-4.01793634009484));
#29751=CARTESIAN_POINT('Ctrl Pts',(-0.0896398427516596,-0.312730802627535,
-4.00205075467033));
#29752=CARTESIAN_POINT('Ctrl Pts',(0.214261622779169,-0.244801579554058,
-3.98616516924583));
#29753=CARTESIAN_POINT('Ctrl Pts',(0.321849162570404,0.0474233360770221,
-3.97027958382132));
#29754=CARTESIAN_POINT('Ctrl Pts',(0.134547344032802,0.296197347328312,
-3.95439399839681));
#29755=CARTESIAN_POINT('Ctrl Pts',(-0.176031415531,0.273585082285939,-3.93850841297231));
#29756=CARTESIAN_POINT('Ctrl Pts',(-0.325324089154259,0.000304681546809577,
-3.9226228275478));
#29757=CARTESIAN_POINT('Ctrl Pts',(-0.176543558622785,-0.273254878447549,
-3.90673724212329));
#29758=CARTESIAN_POINT('Ctrl Pts',(0.133992304976795,-0.29644884826775,
-3.89085165669878));
#29759=CARTESIAN_POINT('Ctrl Pts',(0.321759764077655,-0.048026105758658,
-3.87496607127428));
#29760=CARTESIAN_POINT('Ctrl Pts',(0.214719794236075,0.244399815640059,
-3.85908048584977));
#29761=CARTESIAN_POINT('Ctrl Pts',(-0.0890539319271196,0.312898162064716,
-3.84319490042526));
#29762=CARTESIAN_POINT('Ctrl Pts',(-0.311233285013347,0.0947083521680955,
-3.82730931500076));
#29763=CARTESIAN_POINT('Ctrl Pts',(-0.248250057121239,-0.210256504675443,
-3.81142372957625));
#29764=CARTESIAN_POINT('Ctrl Pts',(0.0421887538711686,-0.32257711831699,
-3.79553814415174));
#29765=CARTESIAN_POINT('Ctrl Pts',(0.29397223293579,-0.13934128999129,-3.77965255872724));
#29766=CARTESIAN_POINT('Ctrl Pts',(0.276409193252869,0.171563655187485,
-3.76376697330273));
#29767=CARTESIAN_POINT('Ctrl Pts',(0.00558847748759769,0.325276424899211,
-3.74788138787822));
#29768=CARTESIAN_POINT('Ctrl Pts',(-0.270348744212762,0.180958901354783,
-3.73199580245371));
#29769=CARTESIAN_POINT('Ctrl Pts',(-0.298590518761739,-0.12915797490149,
-3.71611021702921));
#29770=CARTESIAN_POINT('Ctrl Pts',(-0.0532389236716297,-0.320938669558577,
-3.7002246316047));
#29771=CARTESIAN_POINT('Ctrl Pts',(0.240864211088085,-0.218658756948394,
-3.68433904618019));
#29772=CARTESIAN_POINT('Ctrl Pts',(0.314332958251634,0.0839533061314393,
-3.66845346075569));
#29773=CARTESIAN_POINT('Ctrl Pts',(0.0996950270351602,0.309664909798885,
-3.65256787533118));
#29774=CARTESIAN_POINT('Ctrl Pts',(-0.206085751446533,0.251611064285594,
-3.63668228990667));
#29775=CARTESIAN_POINT('Ctrl Pts',(-0.323435570249458,-0.0368992218868692,
-3.62079670448217));
#29776=CARTESIAN_POINT('Ctrl Pts',(-0.143655123331798,-0.291767639576884,
-3.60491111905766));
#29777=CARTESIAN_POINT('Ctrl Pts',(0.0627426049655472,-0.283154936227829,
-3.59432072877466));
#29778=CARTESIAN_POINT('Ctrl Pts',(0.141308251563369,-0.236140702639086,
-3.58902553363315));
#29779=CARTESIAN_POINT('Ctrl Pts',(0.148738611075533,-0.208582659521589,
-5.97677446636685));
#29780=CARTESIAN_POINT('Ctrl Pts',(0.218135505940597,-0.159096293881898,
-5.97147927122534));
#29781=CARTESIAN_POINT('Ctrl Pts',(0.302439570951552,0.0137485839223339,
-5.96088888094234));
#29782=CARTESIAN_POINT('Ctrl Pts',(0.152071060051237,0.2621306474205,-5.94500329551783));
#29783=CARTESIAN_POINT('Ctrl Pts',(-0.137781807157274,0.269605817244605,
-5.92911771009332));
#29784=CARTESIAN_POINT('Ctrl Pts',(-0.30131488639741,0.0304223318847445,
-5.91323212466882));
#29785=CARTESIAN_POINT('Ctrl Pts',(-0.188813953649519,-0.236821576259721,
-5.89734653924431));
#29786=CARTESIAN_POINT('Ctrl Pts',(0.0967061576779765,-0.286985066330208,
-5.88146095381981));
#29787=CARTESIAN_POINT('Ctrl Pts',(0.293609719765092,-0.0742526863848491,
-5.8655753683953));
#29788=CARTESIAN_POINT('Ctrl Pts',(0.221503578675544,0.206538339262002,
-5.84968978297079));
#29789=CARTESIAN_POINT('Ctrl Pts',(-0.0535547675656337,0.298078451849551,
-5.83380419754629));
#29790=CARTESIAN_POINT('Ctrl Pts',(-0.279542853932516,0.116515650084404,
-5.81791861212177));
#29791=CARTESIAN_POINT('Ctrl Pts',(-0.249404877241599,-0.171806396346182,
-5.80203302669728));
#29792=CARTESIAN_POINT('Ctrl Pts',(0.00924690120339052,-0.302711621625931,
-5.78614744127276));
#29793=CARTESIAN_POINT('Ctrl Pts',(0.259426136989922,-0.156262921440043,
-5.77026185584826));
#29794=CARTESIAN_POINT('Ctrl Pts',(0.271910263115969,0.133359777792746,
-5.75437627042375));
#29795=CARTESIAN_POINT('Ctrl Pts',(0.0352607246525252,0.300793370491302,
-5.73849068499924));
#29796=CARTESIAN_POINT('Ctrl Pts',(-0.233695882691538,0.192629783258305,
-5.72260509957474));
#29797=CARTESIAN_POINT('Ctrl Pts',(-0.288532237064735,-0.0920279567593562,
-5.70671951415023));
#29798=CARTESIAN_POINT('Ctrl Pts',(-0.0790053468812083,-0.292366457518203,
-5.69083392872573));
#29799=CARTESIAN_POINT('Ctrl Pts',(0.20290897655292,-0.224828694182361,
-5.67494834330121));
#29800=CARTESIAN_POINT('Ctrl Pts',(0.298911064518509,0.0487049212675593,
-5.65906275787671));
#29801=CARTESIAN_POINT('Ctrl Pts',(0.121040473208996,0.277613394736605,
-5.6431771724522));
#29802=CARTESIAN_POINT('Ctrl Pts',(-0.167731594607913,0.252162855826698,
-5.6272915870277));
#29803=CARTESIAN_POINT('Ctrl Pts',(-0.302822161809634,-0.00432803339237701,
-5.61140600160319));
#29804=CARTESIAN_POINT('Ctrl Pts',(-0.160456567765648,-0.256853427719911,
-5.59552041617868));
#29805=CARTESIAN_POINT('Ctrl Pts',(0.128924895345672,-0.274040808847988,
-5.57963483075418));
#29806=CARTESIAN_POINT('Ctrl Pts',(0.300180900576644,-0.0401425019038163,
-5.56374924532967));
#29807=CARTESIAN_POINT('Ctrl Pts',(0.196400759784563,0.230535756613179,
-5.54786365990516));
#29808=CARTESIAN_POINT('Ctrl Pts',(-0.087328564769926,0.289989164121325,
-5.53197807448066));
#29809=CARTESIAN_POINT('Ctrl Pts',(-0.291044431298209,0.0837444478091843,
-5.51609248905615));
#29810=CARTESIAN_POINT('Ctrl Pts',(-0.228095301663273,-0.199229834329336,
-5.50020690363164));
#29811=CARTESIAN_POINT('Ctrl Pts',(0.043842649611312,-0.2996628365419,-5.48432131820714));
#29812=CARTESIAN_POINT('Ctrl Pts',(0.275610445635422,-0.125534360974531,
-5.46843573278262));
#29813=CARTESIAN_POINT('Ctrl Pts',(0.254854398137061,0.163613047397773,
-5.45255014735812));
#29814=CARTESIAN_POINT('Ctrl Pts',(0.000591917282580738,0.302852510576879,
-5.43666456193361));
#29815=CARTESIAN_POINT('Ctrl Pts',(-0.25421289870339,0.164608006067476,
-5.4207789765091));
#29816=CARTESIAN_POINT('Ctrl Pts',(-0.276099045349813,-0.124456059256326,
-5.4048933910846));
#29817=CARTESIAN_POINT('Ctrl Pts',(-0.0450136764799851,-0.299489169183916,
-5.38900780566009));
#29818=CARTESIAN_POINT('Ctrl Pts',(0.227314783048407,-0.200119921388048,
-5.37312222023559));
#29819=CARTESIAN_POINT('Ctrl Pts',(0.29136955914499,0.0826061349559363,
-5.35723663481108));
#29820=CARTESIAN_POINT('Ctrl Pts',(0.0884614456784106,0.289645587152977,
-5.34135104938657));
#29821=CARTESIAN_POINT('Ctrl Pts',(-0.195498110576304,0.231301712682376,
-5.32546546396206));
#29822=CARTESIAN_POINT('Ctrl Pts',(-0.300335521550154,-0.0389688083459327,
-5.30957987853756));
#29823=CARTESIAN_POINT('Ctrl Pts',(-0.129995117426334,-0.273534756427806,
-5.29369429311305));
#29824=CARTESIAN_POINT('Ctrl Pts',(0.159451319184456,-0.257478679387327,
-5.27780870768854));
#29825=CARTESIAN_POINT('Ctrl Pts',(0.302802930244308,-0.00551171154598658,
-5.26192312226404));
#29826=CARTESIAN_POINT('Ctrl Pts',(0.168716000835391,0.251505277461166,
-5.24603753683952));
#29827=CARTESIAN_POINT('Ctrl Pts',(-0.119954376586175,0.278084413562731,
-5.23015195141503));
#29828=CARTESIAN_POINT('Ctrl Pts',(-0.298718396311471,0.0498729709743527,
-5.21426636599051));
#29829=CARTESIAN_POINT('Ctrl Pts',(-0.2037862671357,-0.22403381632156,-5.19838078056602));
#29830=CARTESIAN_POINT('Ctrl Pts',(0.0778619036453848,-0.292673055625936,
-5.1824951951415));
#29831=CARTESIAN_POINT('Ctrl Pts',(0.288170299451153,-0.0931550967094044,
-5.166609609717));
#29832=CARTESIAN_POINT('Ctrl Pts',(0.234447078318237,0.191714790761558,
-5.15072402429248));
#29833=CARTESIAN_POINT('Ctrl Pts',(-0.0340846823928767,0.300928941703655,
-5.13483843886799));
#29834=CARTESIAN_POINT('Ctrl Pts',(-0.2713868756497,0.134421565434269,-5.11895285344347));
#29835=CARTESIAN_POINT('Ctrl Pts',(-0.260035006603086,-0.155247508416846,
-5.10306726801897));
#29836=CARTESIAN_POINT('Ctrl Pts',(-0.0104300511529157,-0.302673433855126,
-5.08718168259447));
#29837=CARTESIAN_POINT('Ctrl Pts',(0.248731278690807,-0.172779467905019,
-5.07129609716995));
#29838=CARTESIAN_POINT('Ctrl Pts',(0.279996389454909,0.115421035435144,
-5.05541051174546));
#29839=CARTESIAN_POINT('Ctrl Pts',(0.0547191029435964,0.297868785376638,
-5.03952492632093));
#29840=CARTESIAN_POINT('Ctrl Pts',(-0.22069372236248,0.207398829404841,
-5.02363934089644));
#29841=CARTESIAN_POINT('Ctrl Pts',(-0.293899309536927,-0.0730971229421753,
-5.00775375547193));
#29842=CARTESIAN_POINT('Ctrl Pts',(-0.0978241621527061,-0.286618957551357,
-4.99186817004742));
#29843=CARTESIAN_POINT('Ctrl Pts',(0.18788087338461,-0.237530568443184,
-4.97598258462292));
#29844=CARTESIAN_POINT('Ctrl Pts',(0.301442940385367,0.0291915607758403,
-4.9600969991984));
#29845=CARTESIAN_POINT('Ctrl Pts',(0.138812536766193,0.269167370171868,
-4.9442114137739));
#29846=CARTESIAN_POINT('Ctrl Pts',(-0.15100272456921,0.262522705115921,
-4.92832582834939));
#29847=CARTESIAN_POINT('Ctrl Pts',(-0.302464055586014,0.0153456380501578,
-4.91244024292488));
#29848=CARTESIAN_POINT('Ctrl Pts',(-0.176797334842078,-0.245891634508871,
-4.89655465750038));
#29849=CARTESIAN_POINT('Ctrl Pts',(0.110857232247267,-0.281834468415737,
-4.88066907207587));
#29850=CARTESIAN_POINT('Ctrl Pts',(0.29694056060958,-0.0595507933916408,
-4.86478348665137));
#29851=CARTESIAN_POINT('Ctrl Pts',(0.210956654764379,0.21729538269215,-4.84889790122686));
#29852=CARTESIAN_POINT('Ctrl Pts',(-0.0683130503720702,0.295047997243785,
-4.83301231580235));
#29853=CARTESIAN_POINT('Ctrl Pts',(-0.284991970885316,0.102467409743826,
-4.81712673037784));
#29854=CARTESIAN_POINT('Ctrl Pts',(-0.240551369259371,-0.183997370296825,
-4.80124114495333));
#29855=CARTESIAN_POINT('Ctrl Pts',(0.0242907348924498,-0.301877381940235,
-4.78535555952883));
#29856=CARTESIAN_POINT('Ctrl Pts',(0.266876825768449,-0.143166872552496,
-4.76946997410432));
#29857=CARTESIAN_POINT('Ctrl Pts',(0.264941118369915,0.146718087929213,
-4.75358438867982));
#29858=CARTESIAN_POINT('Ctrl Pts',(0.0202571749110258,0.302174850696298,
-4.73769880325531));
#29859=CARTESIAN_POINT('Ctrl Pts',(-0.242987094357132,0.180768541247043,
-4.72181321783081));
#29860=CARTESIAN_POINT('Ctrl Pts',(-0.283598165337549,-0.106264171506117,
-4.70592763240629));
#29861=CARTESIAN_POINT('Ctrl Pts',(-0.0643667671338396,-0.295933966988319,
-4.69004204698179));
#29862=CARTESIAN_POINT('Ctrl Pts',(0.213839694203828,-0.214458804229434,
-4.67415646155728));
#29863=CARTESIAN_POINT('Ctrl Pts',(0.296118815583686,0.0635109485523635,
-4.65827087613277));
#29864=CARTESIAN_POINT('Ctrl Pts',(0.107083614032142,0.283289768849002,
-4.64238529070827));
#29865=CARTESIAN_POINT('Ctrl Pts',(-0.180065306436283,0.243508683513982,
-4.62649970528376));
#29866=CARTESIAN_POINT('Ctrl Pts',(-0.302232151710002,-0.0193834981736465,
-4.61061411985926));
#29867=CARTESIAN_POINT('Ctrl Pts',(-0.147483423592454,-0.264515846962246,
-4.59472853443474));
#29868=CARTESIAN_POINT('Ctrl Pts',(0.142394729302505,-0.267289608094988,
-4.57884294901024));
#29869=CARTESIAN_POINT('Ctrl Pts',(0.301805895513226,-0.0251633654777264,
-4.56295736358573));
#29870=CARTESIAN_POINT('Ctrl Pts',(0.184692039035091,0.240018424804776,
-4.54707177816123));
#29871=CARTESIAN_POINT('Ctrl Pts',(-0.101643065416946,0.285287014743665,
-4.53118619273672));
#29872=CARTESIAN_POINT('Ctrl Pts',(-0.294849270174067,0.0691657531335122,
-4.51530060731221));
#29873=CARTESIAN_POINT('Ctrl Pts',(-0.217904353509163,-0.210327568926329,
-4.4994150218877));
#29874=CARTESIAN_POINT('Ctrl Pts',(0.0586920848586398,-0.297111481945164,
-4.4835294364632));
#29875=CARTESIAN_POINT('Ctrl Pts',(0.281512800689305,-0.111671556704335,
-4.46764385103869));
#29876=CARTESIAN_POINT('Ctrl Pts',(0.246401730709637,0.176085719557269,
-4.45175826561419));
#29877=CARTESIAN_POINT('Ctrl Pts',(-0.0144711457423287,0.302507156063472,
-4.43587268018968));
#29878=CARTESIAN_POINT('Ctrl Pts',(-0.262085056865184,0.151761050657536,
-4.41998709476516));
#29879=CARTESIAN_POINT('Ctrl Pts',(-0.269567554475346,-0.138033789714284,
-4.40410150934067));
#29880=CARTESIAN_POINT('Ctrl Pts',(-0.0300629149034655,-0.301357287411823,
-4.38821592391615));
#29881=CARTESIAN_POINT('Ctrl Pts',(0.236986409346085,-0.188566792712703,
-4.37233033849166));
#29882=CARTESIAN_POINT('Ctrl Pts',(0.286900570911232,0.0969951335867651,
-4.35644475306714));
#29883=CARTESIAN_POINT('Ctrl Pts',(0.0739464848374023,0.293686756441107,
-4.34055916764264));
#29884=CARTESIAN_POINT('Ctrl Pts',(-0.206759933783318,0.221292393250703,
-4.32467358221813));
#29885=CARTESIAN_POINT('Ctrl Pts',(-0.298025734342708,-0.0538577310902972,
-4.30878799679363));
#29886=CARTESIAN_POINT('Ctrl Pts',(-0.116230026905917,-0.279661535385465,
-4.29290241136911));
#29887=CARTESIAN_POINT('Ctrl Pts',(0.172059659956391,-0.249229747310381,
-4.27701682594461));
#29888=CARTESIAN_POINT('Ctrl Pts',(0.302702322421217,0.00955497407153588,
-4.2611312405201));
#29889=CARTESIAN_POINT('Ctrl Pts',(0.155998624792064,0.259585097013851,
-4.2452456550956));
#29890=CARTESIAN_POINT('Ctrl Pts',(-0.133636420108152,0.271774356313068,
-4.22936006967109));
#29891=CARTESIAN_POINT('Ctrl Pts',(-0.3008291447892,0.0349545300941856,
-4.21347448424658));
#29892=CARTESIAN_POINT('Ctrl Pts',(-0.192391779650948,-0.233891848193658,
-4.19758889882208));
#29893=CARTESIAN_POINT('Ctrl Pts',(0.0923216027024518,-0.288438407988869,
-4.18170331339757));
#29894=CARTESIAN_POINT('Ctrl Pts',(0.292446732601261,-0.0787077005099487,
-4.16581772797307));
#29895=CARTESIAN_POINT('Ctrl Pts',(0.224622029279129,0.203137730348692,
-4.14993214254855));
#29896=CARTESIAN_POINT('Ctrl Pts',(-0.0490091631348199,0.298861331485884,
-4.13404655712405));
#29897=CARTESIAN_POINT('Ctrl Pts',(-0.27773646152544,0.120757821560827,
-4.11816097169954));
#29898=CARTESIAN_POINT('Ctrl Pts',(-0.251991986942937,-0.167988190195444,
-4.10227538627504));
#29899=CARTESIAN_POINT('Ctrl Pts',(0.00463628064177704,-0.302817599274629,
-4.08638980085052));
#29900=CARTESIAN_POINT('Ctrl Pts',(0.257016627201181,-0.160195027611366,
-4.07050421542602));
#29901=CARTESIAN_POINT('Ctrl Pts',(0.273909431184861,0.12920378104274,-4.05461863000152));
#29902=CARTESIAN_POINT('Ctrl Pts',(0.0398369200535349,0.300221607032558,
-4.038733044577));
#29903=CARTESIAN_POINT('Ctrl Pts',(-0.230735558074371,0.196165990356812,
-4.0228474591525));
#29904=CARTESIAN_POINT('Ctrl Pts',(-0.289900120095227,-0.087623706209775,
-4.00696187372799));
#29905=CARTESIAN_POINT('Ctrl Pts',(-0.0834481435929966,-0.291129525917563,
-3.99107628830349));
#29906=CARTESIAN_POINT('Ctrl Pts',(0.199461914649706,-0.227892382843801,
-3.97519070287898));
#29907=CARTESIAN_POINT('Ctrl Pts',(0.29961805274322,0.0441476606510558,
-3.95930511745447));
#29908=CARTESIAN_POINT('Ctrl Pts',(0.125253745881852,0.275738087138265,
-3.94341953202996));
#29909=CARTESIAN_POINT('Ctrl Pts',(-0.163872385193774,0.254687720668454,
-3.92753394660546));
#29910=CARTESIAN_POINT('Ctrl Pts',(-0.302852955478915,0.000283636256912637,
-3.91164836118095));
#29911=CARTESIAN_POINT('Ctrl Pts',(-0.164349152989785,-0.254380325023001,
-3.89576277575645));
#29912=CARTESIAN_POINT('Ctrl Pts',(0.124737045077571,-0.275972216135638,
-3.87987719033194));
#29913=CARTESIAN_POINT('Ctrl Pts',(0.299534829278844,-0.0447087951801068,
-3.86399160490743));
#29914=CARTESIAN_POINT('Ctrl Pts',(0.199888438797366,0.227518369996871,
-3.84810601948293));
#29915=CARTESIAN_POINT('Ctrl Pts',(-0.0829027034280202,0.291285325324577,
-3.83222043405842));
#29916=CARTESIAN_POINT('Ctrl Pts',(-0.289735446442791,0.0881665555022742,
-3.81633484863391));
#29917=CARTESIAN_POINT('Ctrl Pts',(-0.231102663477611,-0.195733442350255,
-3.8004492632094));
#29918=CARTESIAN_POINT('Ctrl Pts',(0.0392746471098163,-0.300295726351358,
-3.78456367778489));
#29919=CARTESIAN_POINT('Ctrl Pts',(0.273666668228569,-0.12971655927421,
-3.76867809236039));
#29920=CARTESIAN_POINT('Ctrl Pts',(0.257316761620074,0.15971322677448,-3.75279250693588));
#29921=CARTESIAN_POINT('Ctrl Pts',(0.00520246418931447,0.302808583540306,
-3.73690692151138));
#29922=CARTESIAN_POINT('Ctrl Pts',(-0.251674926402469,0.168459514442926,
-3.72102133608687));
#29923=CARTESIAN_POINT('Ctrl Pts',(-0.27796595487307,-0.120236637023335,
-3.70513575066236));
#29924=CARTESIAN_POINT('Ctrl Pts',(-0.0495615477549964,-0.298770450279193,
-3.68925016523786));
#29925=CARTESIAN_POINT('Ctrl Pts',(0.224226980506614,-0.20355532526141,
-3.67336457981335));
#29926=CARTESIAN_POINT('Ctrl Pts',(0.292621015733633,0.0781543935164189,
-3.65747899438884));
#29927=CARTESIAN_POINT('Ctrl Pts',(0.0928087854257608,0.288275403719751,
-3.64159340896433));
#29928=CARTESIAN_POINT('Ctrl Pts',(-0.191850775852264,0.234231515557876,
-3.62570782353983));
#29929=CARTESIAN_POINT('Ctrl Pts',(-0.301094882373159,-0.0343504793400395,
-3.60982223811532));
#29930=CARTESIAN_POINT('Ctrl Pts',(-0.133732422901194,-0.271614352901692,
-3.59393665269081));
#29931=CARTESIAN_POINT('Ctrl Pts',(0.058408780602939,-0.263596555416404,
-3.58334626240781));
#29932=CARTESIAN_POINT('Ctrl Pts',(0.131547656771374,-0.219829739288701,
-3.57805106726631));
#29933=CARTESIAN_POINT('Ctrl Pts',(0.137702479013101,-0.193106208855765,
-5.9658));
#29934=CARTESIAN_POINT('Ctrl Pts',(0.201950251596361,-0.147291640757684,
-5.9605048048585));
#29935=CARTESIAN_POINT('Ctrl Pts',(0.279999109649734,0.0127284642187734,
-5.9499144145755));
#29936=CARTESIAN_POINT('Ctrl Pts',(0.140787666388597,0.242681034292982,
-5.93402882915098));
#29937=CARTESIAN_POINT('Ctrl Pts',(-0.127558649843965,0.249601560230261,
-5.91814324372648));
#29938=CARTESIAN_POINT('Ctrl Pts',(-0.278957874626137,0.0281650506724263,
-5.90225765830197));
#29939=CARTESIAN_POINT('Ctrl Pts',(-0.174804304691268,-0.219249849779713,
-5.88637207287746));
#29940=CARTESIAN_POINT('Ctrl Pts',(0.0895307381976737,-0.265691300918094,
-5.87048648745296));
#29941=CARTESIAN_POINT('Ctrl Pts',(0.271824417221856,-0.0687432732808278,
-5.85460090202845));
#29942=CARTESIAN_POINT('Ctrl Pts',(0.205068419513521,0.191213573408882,
-5.83871531660395));
#29943=CARTESIAN_POINT('Ctrl Pts',(-0.0495811020651061,0.275961577584089,
-5.82282973117944));
#29944=CARTESIAN_POINT('Ctrl Pts',(-0.258801287026652,0.107870402610509,
-5.80694414575493));
#29945=CARTESIAN_POINT('Ctrl Pts',(-0.230899492914356,-0.159058676937372,
-5.79105856033042));
#29946=CARTESIAN_POINT('Ctrl Pts',(0.00856079809868226,-0.280250974663184,
-5.77517297490592));
#29947=CARTESIAN_POINT('Ctrl Pts',(0.240177193574594,-0.144668499352843,
-5.75928738948141));
#29948=CARTESIAN_POINT('Ctrl Pts',(0.251735020445761,0.123464726945526,
-5.74340180405691));
#29949=CARTESIAN_POINT('Ctrl Pts',(0.0326444435734673,0.278475054243476,
-5.72751621863239));
#29950=CARTESIAN_POINT('Ctrl Pts',(-0.216356076939817,0.178337006743693,
-5.7116306332079));
#29951=CARTESIAN_POINT('Ctrl Pts',(-0.267123674422595,-0.0851996512044772,
-5.69574504778338));
#29952=CARTESIAN_POINT('Ctrl Pts',(-0.0731432950877003,-0.270673402752768,
-5.67985946235888));
#29953=CARTESIAN_POINT('Ctrl Pts',(0.187853502754299,-0.208146817550068,
-5.66397387693437));
#29954=CARTESIAN_POINT('Ctrl Pts',(0.276732411920541,0.0450911054647064,
-5.64808829150987));
#29955=CARTESIAN_POINT('Ctrl Pts',(0.112059492160603,0.257014990163246,
-5.63220270608536));
#29956=CARTESIAN_POINT('Ctrl Pts',(-0.155286218012354,0.233452834548294,
-5.61631712066085));
#29957=CARTESIAN_POINT('Ctrl Pts',(-0.280353312968057,-0.00400690125497473,
-5.60043153523634));
#29958=CARTESIAN_POINT('Ctrl Pts',(-0.14855098481485,-0.237795374612464,
-5.58454594981183));
#29959=CARTESIAN_POINT('Ctrl Pts',(0.119358904639683,-0.253707483593214,
-5.56866036438733));
#29960=CARTESIAN_POINT('Ctrl Pts',(0.277908028472834,-0.0371640019089366,
-5.55277477896282));
#29961=CARTESIAN_POINT('Ctrl Pts',(0.181828183730025,0.21343042641883,-5.53688919353832));
#29962=CARTESIAN_POINT('Ctrl Pts',(-0.0808489454790468,0.268472500164499,
-5.52100360811381));
#29963=CARTESIAN_POINT('Ctrl Pts',(-0.269449468452876,0.0775307634212869,
-5.5051180226893));
#29964=CARTESIAN_POINT('Ctrl Pts',(-0.211171048748891,-0.184447346133863,
-5.48923243726479));
#29965=CARTESIAN_POINT('Ctrl Pts',(0.040589605444914,-0.277428403839015,
-5.47334685184029));
#29966=CARTESIAN_POINT('Ctrl Pts',(0.255160656210713,-0.116219941698528,
-5.45746126641578));
#29967=CARTESIAN_POINT('Ctrl Pts',(0.235944669357195,0.151473259449223,
-5.44157568099128));
#29968=CARTESIAN_POINT('Ctrl Pts',(0.000547998106158669,0.280381409912451,
-5.42569009556676));
#29969=CARTESIAN_POINT('Ctrl Pts',(-0.235350768004592,0.152394394011009,
-5.40980451014226));
#29970=CARTESIAN_POINT('Ctrl Pts',(-0.255613002722693,-0.115221647989535,
-5.39391892471775));
#29971=CARTESIAN_POINT('Ctrl Pts',(-0.0416737442683253,-0.27726762228038,
-5.37803333929325));
#29972=CARTESIAN_POINT('Ctrl Pts',(0.21044844318329,-0.185271390365794,
-5.36214775386874));
#29973=CARTESIAN_POINT('Ctrl Pts',(0.269750472409913,0.0764769112933738,
-5.34626216844423));
#29974=CARTESIAN_POINT('Ctrl Pts',(0.0818977687025324,0.268154415976868,
-5.33037658301972));
#29975=CARTESIAN_POINT('Ctrl Pts',(-0.180992509436998,0.214139549952934,
-5.31449099759522));
#29976=CARTESIAN_POINT('Ctrl Pts',(-0.278051176853781,-0.0360773942597614,
-5.2986054121707));
#29977=CARTESIAN_POINT('Ctrl Pts',(-0.120349718205416,-0.253238979334194,
-5.28271982674621));
#29978=CARTESIAN_POINT('Ctrl Pts',(0.147620323834129,-0.23837423375326,
-5.2668342413217));
#29979=CARTESIAN_POINT('Ctrl Pts',(0.280335508349595,-0.00510275266119098,
-5.25094865589719));
#29980=CARTESIAN_POINT('Ctrl Pts',(0.156197583103769,0.232844047291076,
-5.23506307047268));
#29981=CARTESIAN_POINT('Ctrl Pts',(-0.111053981914616,0.257451060256615,
-5.21917748504818));
#29982=CARTESIAN_POINT('Ctrl Pts',(-0.276554039340992,0.0461724880261877,
-5.20329189962367));
#29983=CARTESIAN_POINT('Ctrl Pts',(-0.188665699985335,-0.207410918168237,
-5.18740631419917));
#29984=CARTESIAN_POINT('Ctrl Pts',(0.0720846932421861,-0.270957251843399,
-5.17152072877465));
#29985=CARTESIAN_POINT('Ctrl Pts',(0.266788591915922,-0.0862431594381096,
-5.15563514335015));
#29986=CARTESIAN_POINT('Ctrl Pts',(0.217051535229177,0.177489905011538,
-5.13974955792564));
#29987=CARTESIAN_POINT('Ctrl Pts',(-0.0315556614918893,0.278600566320595,
-5.12386397250114));
#29988=CARTESIAN_POINT('Ctrl Pts',(-0.251250467369271,0.124447731892029,
-5.10797838707663));
#29989=CARTESIAN_POINT('Ctrl Pts',(-0.240740886179508,-0.143728428113065,
-5.09209280165212));
#29990=CARTESIAN_POINT('Ctrl Pts',(-0.00965616049258788,-0.280215620354914,
-5.07620721622762));
#29991=CARTESIAN_POINT('Ctrl Pts',(0.230275874140234,-0.159959548371763,
-5.0603216308031));
#29992=CARTESIAN_POINT('Ctrl Pts',(0.25922117104535,0.106857006360016,-5.04443604537861));
#29993=CARTESIAN_POINT('Ctrl Pts',(0.0506590458941416,0.275767467978807,
-5.02855045995409));
#29994=CARTESIAN_POINT('Ctrl Pts',(-0.204318653053104,0.192010216761797,
-5.01266487452959));
#29995=CARTESIAN_POINT('Ctrl Pts',(-0.272092519963909,-0.0676734505255753,
-4.99677928910508));
#29996=CARTESIAN_POINT('Ctrl Pts',(-0.0905657887914961,-0.265352356738962,
-4.98089370368057));
#29997=CARTESIAN_POINT('Ctrl Pts',(0.173940457270164,-0.219906236043896,
-4.96500811825607));
#29998=CARTESIAN_POINT('Ctrl Pts',(0.279076427243118,0.0270256005218002,
-4.94912253283156));
#29999=CARTESIAN_POINT('Ctrl Pts',(0.128512901206904,0.249195645125937,
-4.93323694740706));
#30000=CARTESIAN_POINT('Ctrl Pts',(-0.139798599439343,0.243044002026681,
-4.91735136198254));
#30001=CARTESIAN_POINT('Ctrl Pts',(-0.280021777569238,0.0142070198603066,
-4.90146577655804));
#30002=CARTESIAN_POINT('Ctrl Pts',(-0.163679296953366,-0.227646926346919,
-4.88558019113353));
#30003=CARTESIAN_POINT('Ctrl Pts',(0.102631828995819,-0.260922867919469,
-4.86969460570902));
#30004=CARTESIAN_POINT('Ctrl Pts',(0.274908115786522,-0.0551322337752745,
-4.85380902028452));
#30005=CARTESIAN_POINT('Ctrl Pts',(0.195304058006928,0.201172463951639,
-4.83792343486001));
#30006=CARTESIAN_POINT('Ctrl Pts',(-0.0632443473631996,0.273155977150327,
-4.82203784943551));
#30007=CARTESIAN_POINT('Ctrl Pts',(-0.263846089498633,0.0948645159299668,
-4.806152264011));
#30008=CARTESIAN_POINT('Ctrl Pts',(-0.222702898981555,-0.170345102986727,
-4.79026667858649));
#30009=CARTESIAN_POINT('Ctrl Pts',(0.0224884069277866,-0.279478634031651,
-4.77438109316199));
#30010=CARTESIAN_POINT('Ctrl Pts',(0.247075054914963,-0.13254415326643,
-4.75849550773747));
#30011=CARTESIAN_POINT('Ctrl Pts',(0.245282973454107,0.135831874977338,
-4.74260992231297));
#30012=CARTESIAN_POINT('Ctrl Pts',(0.0187541296969196,0.279754031151758,
-4.72672433688846));
#30013=CARTESIAN_POINT('Ctrl Pts',(-0.224957897745701,0.167355847128752,
-4.71083875146396));
#30014=CARTESIAN_POINT('Ctrl Pts',(-0.262555701765402,-0.0983795649351243,
-4.69495316603945));
#30015=CARTESIAN_POINT('Ctrl Pts',(-0.0595908711013016,-0.273976209565238,
-4.67906758061494));
#30016=CARTESIAN_POINT('Ctrl Pts',(0.197973181209263,-0.198546354406802,
-4.66318199519043));
#30017=CARTESIAN_POINT('Ctrl Pts',(0.274147342733956,0.0587985526884655,
-4.64729640976593));
#30018=CARTESIAN_POINT('Ctrl Pts',(0.0991382063290872,0.262270187730513,
-4.63141082434142));
#30019=CARTESIAN_POINT('Ctrl Pts',(-0.16670479105078,0.225440785944032,
-4.61552523891691));
#30020=CARTESIAN_POINT('Ctrl Pts',(-0.279807080535371,-0.0179452781705858,
-4.59963965349241));
#30021=CARTESIAN_POINT('Ctrl Pts',(-0.13654042413847,-0.244889256404674,
-4.5837540680679));
#30022=CARTESIAN_POINT('Ctrl Pts',(0.131829301628996,-0.247457209550174,
-4.56786848264339));
#30023=CARTESIAN_POINT('Ctrl Pts',(0.279412451766375,-0.0232962899245847,
-4.55198289721889));
#30024=CARTESIAN_POINT('Ctrl Pts',(0.170988228579068,0.222209498027739,
-4.53609731179438));
#30025=CARTESIAN_POINT('Ctrl Pts',(-0.0941013364397791,0.264119241643986,
-4.52021172636988));
#30026=CARTESIAN_POINT('Ctrl Pts',(-0.272971995264593,0.0640337811441318,
-4.50432614094536));
#30027=CARTESIAN_POINT('Ctrl Pts',(-0.201736250251262,-0.194721649183925,
-4.48844055552086));
#30028=CARTESIAN_POINT('Ctrl Pts',(0.0543372398400151,-0.275066355072582,
-4.47255497009635));
#30029=CARTESIAN_POINT('Ctrl Pts',(0.260625067348198,-0.103385732072151,
-4.45666938467185));
#30030=CARTESIAN_POINT('Ctrl Pts',(0.228119174345422,0.163020482217144,
-4.44078379924733));
#30031=CARTESIAN_POINT('Ctrl Pts',(-0.0133974132773538,0.280061680070342,
-4.42489821382283));
#30032=CARTESIAN_POINT('Ctrl Pts',(-0.242638826473229,0.140500659123159,
-4.40901262839833));
#30033=CARTESIAN_POINT('Ctrl Pts',(-0.249566136488284,-0.127791935757538,
-4.39312704297382));
#30034=CARTESIAN_POINT('Ctrl Pts',(-0.0278323017717629,-0.27899712956307,
-4.37724145754931));
#30035=CARTESIAN_POINT('Ctrl Pts',(0.219402452553475,-0.174575482642516,
-4.36135587212481));
#30036=CARTESIAN_POINT('Ctrl Pts',(0.265613074904189,0.0897982726241923,
-4.3454702867003));
#30037=CARTESIAN_POINT('Ctrl Pts',(0.0684597913264363,0.271895737917843,
-4.32958470127579));
#30038=CARTESIAN_POINT('Ctrl Pts',(-0.191418726023258,0.204872903659757,
-4.31369911585128));
#30039=CARTESIAN_POINT('Ctrl Pts',(-0.275912771619538,-0.0498615862520642,
-4.29781353042678));
#30040=CARTESIAN_POINT('Ctrl Pts',(-0.107605972147853,-0.258911162533527,
-4.28192794500227));
#30041=CARTESIAN_POINT('Ctrl Pts',(0.159293148852347,-0.230737357302738,
-4.26604235957777));
#30042=CARTESIAN_POINT('Ctrl Pts',(0.2802423654424,0.00884601252520937,
-4.25015677415325));
#30043=CARTESIAN_POINT('Ctrl Pts',(0.144423813031258,0.240324359056379,
-4.23427118872875));
#30044=CARTESIAN_POINT('Ctrl Pts',(-0.123720842908662,0.251609197678298,
-4.21838560330425));
#30045=CARTESIAN_POINT('Ctrl Pts',(-0.278508174154103,0.0323609680896043,
-4.20250001787973));
#30046=CARTESIAN_POINT('Ctrl Pts',(-0.178116662567355,-0.216537502161203,
-4.18661443245523));
#30047=CARTESIAN_POINT('Ctrl Pts',(0.0854715091573248,-0.267036807292018,
-4.17072884703072));
#30048=CARTESIAN_POINT('Ctrl Pts',(0.270747721571937,-0.0728677335311189,
-4.15484326160622));
#30049=CARTESIAN_POINT('Ctrl Pts',(0.207955486803503,0.188065283438102,
-4.1389576761817));
#30050=CARTESIAN_POINT('Ctrl Pts',(-0.0453727731435854,0.276686368987695,
-4.12307209075721));
#30051=CARTESIAN_POINT('Ctrl Pts',(-0.257128925622131,0.111797812746169,
-4.10718650533269));
#30052=CARTESIAN_POINT('Ctrl Pts',(-0.233294643822228,-0.155523774678048,
-4.09130091990819));
#30053=CARTESIAN_POINT('Ctrl Pts',(0.00429227712398719,-0.280349088964778,
-4.07541533448367));
#30054=CARTESIAN_POINT('Ctrl Pts',(0.237946464991633,-0.148308850460187,
-4.05952974905918));
#30055=CARTESIAN_POINT('Ctrl Pts',(0.253585853911662,0.11961709752968,-4.04364416363466));
#30056=CARTESIAN_POINT('Ctrl Pts',(0.0368810936713182,0.2779457145844,-4.02775857821017));
#30057=CARTESIAN_POINT('Ctrl Pts',(-0.213615402978162,0.1816108337631,-4.01187299278565));
#30058=CARTESIAN_POINT('Ctrl Pts',(-0.268390063041775,-0.0811221879655325,
-3.99598740736115));
#30059=CARTESIAN_POINT('Ctrl Pts',(-0.0772564444343335,-0.269528249207591,
-3.98010182193664));
#30060=CARTESIAN_POINT('Ctrl Pts',(0.184662206520241,-0.210983186133545,
-3.96421623651213));
#30061=CARTESIAN_POINT('Ctrl Pts',(0.277386942916036,0.0408719852250892,
-3.94833065108763));
#30062=CARTESIAN_POINT('Ctrl Pts',(0.115960147730902,0.25527882694822,-3.93244506566312));
#30063=CARTESIAN_POINT('Ctrl Pts',(-0.151713354856548,0.235790359050968,
-3.91655948023861));
#30064=CARTESIAN_POINT('Ctrl Pts',(-0.280381821803572,0.000262590967015663,
-3.9006738948141));
#30065=CARTESIAN_POINT('Ctrl Pts',(-0.152154747356785,-0.235505771598453,
-3.8847883093896));
#30066=CARTESIAN_POINT('Ctrl Pts',(0.115481785178347,-0.255495584003526,
-3.86890272396509));
#30067=CARTESIAN_POINT('Ctrl Pts',(0.277309894480033,-0.0413914846015558,
-3.85301713854059));
#30068=CARTESIAN_POINT('Ctrl Pts',(0.185057083358657,0.210636924353684,
-3.83713155311608));
#30069=CARTESIAN_POINT('Ctrl Pts',(-0.0767514749289204,0.269672488584438,
-3.82124596769156));
#30070=CARTESIAN_POINT('Ctrl Pts',(-0.268237607872236,0.0816247588364526,
-3.80536038226707));
#30071=CARTESIAN_POINT('Ctrl Pts',(-0.213955269833982,-0.181210380025067,
-3.78947479684255));
#30072=CARTESIAN_POINT('Ctrl Pts',(0.0363605403484637,-0.278014334385727,
-3.77358921141805));
#30073=CARTESIAN_POINT('Ctrl Pts',(0.253361103521349,-0.12009182855713,
-3.75770362599354));
#30074=CARTESIAN_POINT('Ctrl Pts',(0.238224329987279,0.147862798361475,
-3.74181804056903));
#30075=CARTESIAN_POINT('Ctrl Pts',(0.00481645089103148,0.280340742181402,
-3.72593245514453));
#30076=CARTESIAN_POINT('Ctrl Pts',(-0.233001108592176,0.155960127531069,
-3.71004686972002));
#30077=CARTESIAN_POINT('Ctrl Pts',(-0.2573413909844,-0.111315299145181,
-3.69416128429552));
#30078=CARTESIAN_POINT('Ctrl Pts',(-0.0458841718383633,-0.276602230999808,
-3.67827569887101));
#30079=CARTESIAN_POINT('Ctrl Pts',(0.207589749925143,-0.188451893574426,
-3.6623901134465));
#30080=CARTESIAN_POINT('Ctrl Pts',(0.27090907321563,0.0723554809013986,
-3.64650452802199));
#30081=CARTESIAN_POINT('Ctrl Pts',(0.0859225438163616,0.266885897640616,
-3.63061894259749));
#30082=CARTESIAN_POINT('Ctrl Pts',(-0.177615800257995,0.216851966830158,
-3.61473335717298));
#30083=CARTESIAN_POINT('Ctrl Pts',(-0.27875419449686,-0.0318017367932098,
-3.59884777174848));
#30084=CARTESIAN_POINT('Ctrl Pts',(-0.123809722470591,-0.251461066226499,
-3.58296218632396));
#30085=CARTESIAN_POINT('Ctrl Pts',(0.0540749562403304,-0.24403817460498,
-3.57237179604096));
#30086=CARTESIAN_POINT('Ctrl Pts',(0.12178706197938,-0.203518775938317,
-3.56707660089946));
#30087=CARTESIAN_POINT('',(0.151068846355364,-0.252451665989471,-3.6));
#30088=CARTESIAN_POINT('Ctrl Pts',(-0.237357402024655,-0.00992348605842327,
-3.6));
#30089=CARTESIAN_POINT('Ctrl Pts',(-0.237818158165497,-0.0156781358441794,
-3.6));
#30090=CARTESIAN_POINT('Ctrl Pts',(-0.238053973041474,-0.0214395997296665,
-3.6));
#30091=CARTESIAN_POINT('Ctrl Pts',(-0.238060167870929,-0.0271962756202516,
-3.6));
#30092=CARTESIAN_POINT('Ctrl Pts',(-0.23807319373073,-0.0393008304937199,
-3.6));
#30093=CARTESIAN_POINT('Ctrl Pts',(-0.237072714474431,-0.0513839386958204,
-3.6));
#30094=CARTESIAN_POINT('Ctrl Pts',(-0.235138076370835,-0.0633587566056082,
-3.6));
#30095=CARTESIAN_POINT('Ctrl Pts',(-0.234045286901415,-0.0701227890547415,
-3.6));
#30096=CARTESIAN_POINT('Ctrl Pts',(-0.232652433897081,-0.0768567577364692,
-3.6));
#30097=CARTESIAN_POINT('Ctrl Pts',(-0.230979008350505,-0.0835169074499154,
-3.6));
#30098=CARTESIAN_POINT('Ctrl Pts',(-0.228489157220848,-0.0934263900209443,
-3.6));
#30099=CARTESIAN_POINT('Ctrl Pts',(-0.225377725547669,-0.103183572699323,
-3.6));
#30100=CARTESIAN_POINT('Ctrl Pts',(-0.22168847500784,-0.112738759405678,
-3.6));
#30101=CARTESIAN_POINT('Ctrl Pts',(-0.219352585423726,-0.118788731035598,
-3.6));
#30102=CARTESIAN_POINT('Ctrl Pts',(-0.216784829686237,-0.124757762683027,
-3.6));
#30103=CARTESIAN_POINT('Ctrl Pts',(-0.213994183376544,-0.130633189689497,
-3.6));
#30104=CARTESIAN_POINT('Ctrl Pts',(-0.21192012642273,-0.134999909397786,
-3.6));
#30105=CARTESIAN_POINT('Ctrl Pts',(-0.209722616116855,-0.139314910937566,
-3.6));
#30106=CARTESIAN_POINT('Ctrl Pts',(-0.207412785002291,-0.143559868692326,
-3.6));
#30107=CARTESIAN_POINT('Ctrl Pts',(-0.199758222129867,-0.157627259082777,
-3.6));
#30108=CARTESIAN_POINT('Ctrl Pts',(-0.190857579307457,-0.170962640513682,
-3.6));
#30109=CARTESIAN_POINT('Ctrl Pts',(-0.18085588350525,-0.18338771537786,
-3.6));
#30110=CARTESIAN_POINT('Ctrl Pts',(-0.173977043171628,-0.19193327683206,
-3.6));
#30111=CARTESIAN_POINT('Ctrl Pts',(-0.166576167133203,-0.200048359000074,
-3.6));
#30112=CARTESIAN_POINT('Ctrl Pts',(-0.158687164513189,-0.207670103762131,
-3.6));
#30113=CARTESIAN_POINT('Ctrl Pts',(-0.154249377376733,-0.211957550793344,
-3.6));
#30114=CARTESIAN_POINT('Ctrl Pts',(-0.149652386008849,-0.216092093447304,
-3.6));
#30115=CARTESIAN_POINT('Ctrl Pts',(-0.14492682489689,-0.220041323919562,
-3.6));
#30116=CARTESIAN_POINT('Ctrl Pts',(-0.136444610605299,-0.227130052296771,
-3.6));
#30117=CARTESIAN_POINT('Ctrl Pts',(-0.127537649227004,-0.233634454227581,
-3.6));
#30118=CARTESIAN_POINT('Ctrl Pts',(-0.118247429613959,-0.239497288460027,
-3.6));
#30119=CARTESIAN_POINT('Ctrl Pts',(-0.108421132217647,-0.245698428492541,
-3.6));
#30120=CARTESIAN_POINT('Ctrl Pts',(-0.0981660718109667,-0.251182303133843,
-3.6));
#30121=CARTESIAN_POINT('Ctrl Pts',(-0.0875605794596233,-0.255961502708628,
-3.6));
#30122=CARTESIAN_POINT('Ctrl Pts',(-0.0808528732519119,-0.25898422580282,
-3.6));
#30123=CARTESIAN_POINT('Ctrl Pts',(-0.0740047561970901,-0.261724835303419,
-3.6));
#30124=CARTESIAN_POINT('Ctrl Pts',(-0.0670343043536097,-0.264184035594139,
-3.6));
#30125=CARTESIAN_POINT('Ctrl Pts',(-0.0628591814074491,-0.265657033872234,
-3.6));
#30126=CARTESIAN_POINT('Ctrl Pts',(-0.0586406755024959,-0.2670286085373,
-3.6));
#30127=CARTESIAN_POINT('Ctrl Pts',(-0.0543960005259033,-0.268295339221923,
-3.6));
#30128=CARTESIAN_POINT('Ctrl Pts',(-0.0385528896482364,-0.273023370178188,
-3.6));
#30129=CARTESIAN_POINT('Ctrl Pts',(-0.0223017363277034,-0.27631099702761,
-3.6));
#30130=CARTESIAN_POINT('Ctrl Pts',(-0.00585688672513749,-0.278193970555172,
-3.6));
#30131=CARTESIAN_POINT('Ctrl Pts',(0.00913418873160995,-0.279910483561794,
-3.6));
#30132=CARTESIAN_POINT('Ctrl Pts',(0.0242875292752077,-0.280459386992588,
-3.6));
#30133=CARTESIAN_POINT('Ctrl Pts',(0.039455058586787,-0.279835389708545,
-3.6));
#30134=CARTESIAN_POINT('Ctrl Pts',(0.0439432239296933,-0.279650745068882,
-3.6));
#30135=CARTESIAN_POINT('Ctrl Pts',(0.0484311331096738,-0.27936305622478,
-3.6));
#30136=CARTESIAN_POINT('Ctrl Pts',(0.0529025262859033,-0.278973505850679,
-3.6));
#30137=CARTESIAN_POINT('Ctrl Pts',(0.0703010175478352,-0.27745773917288,
-3.6));
#30138=CARTESIAN_POINT('Ctrl Pts',(0.0874990268864668,-0.27440207329904,
-3.6));
#30139=CARTESIAN_POINT('Ctrl Pts',(0.104273027409705,-0.269821510755089,
-3.6));
#30140=CARTESIAN_POINT('Ctrl Pts',(0.120323834386248,-0.265438434390266,
-3.6));
#30141=CARTESIAN_POINT('Ctrl Pts',(0.135987913442794,-0.259659004054616,
-3.6));
#30142=CARTESIAN_POINT('Ctrl Pts',(0.151068846355364,-0.252451665989471,
-3.6));
#30143=CARTESIAN_POINT('Ctrl Pts',(0.151068846355364,-0.252451665989471,
-3.6));
#30144=CARTESIAN_POINT('Ctrl Pts',(0.0670764293281557,-0.302713317039253,
-3.6052951951415));
#30145=CARTESIAN_POINT('Ctrl Pts',(-0.043250697217123,-0.307317121645665,
-3.610590390283));
#30146=CARTESIAN_POINT('Ctrl Pts',(-0.130447332883655,-0.264206863645807,
-3.61588558542451));
#30147=CARTESIAN_POINT('Ctrl Pts',(-0.217643968550187,-0.22109660564595,
-3.62118078056601));
#30148=CARTESIAN_POINT('Ctrl Pts',(-0.281710113337973,-0.130272285039823,
-3.62647597570751));
#30149=CARTESIAN_POINT('Ctrl Pts',(-0.292833930551039,-0.033453695162257,
-3.63177117084901));
#30150=CARTESIAN_POINT('Ctrl Pts',(-0.294102228269998,-0.0224147869940842,
-3.63237490999636));
#30151=CARTESIAN_POINT('Ctrl Pts',(-0.294682289386786,-0.0112979548715849,
-3.6329786491437));
#30152=CARTESIAN_POINT('Ctrl Pts',(-0.294602820716591,-0.000172945526623114,
-3.63358238829104));
#30153=CARTESIAN_POINT('Origin',(0.,0.,0.225002200032268));
#30154=CARTESIAN_POINT('',(0.,0.,0.150004400064535));
#30155=CARTESIAN_POINT('',(-0.249992666559108,-3.06152718911923E-17,0.3));
#30156=CARTESIAN_POINT('',(-0.124996333279554,-1.53076359455962E-17,0.225002200032268));
#30157=CARTESIAN_POINT('Origin',(0.,0.,0.3));
#30158=CARTESIAN_POINT('Origin',(0.144337567297406,0.25,0.6));
#30159=CARTESIAN_POINT('',(0.144337567297406,0.25,0.6));
#30160=CARTESIAN_POINT('',(0.288675134594813,0.,0.6));
#30161=CARTESIAN_POINT('',(0.180421959121758,0.1875,0.6));
#30162=CARTESIAN_POINT('',(0.144337567297406,0.25,0.3));
#30163=CARTESIAN_POINT('',(0.144337567297406,0.25,0.6));
#30164=CARTESIAN_POINT('',(0.288675134594813,0.,0.3));
#30165=CARTESIAN_POINT('',(0.288675134594813,0.,0.3));
#30166=CARTESIAN_POINT('',(0.288675134594813,0.,0.6));
#30167=CARTESIAN_POINT('Origin',(-0.144337567297406,0.25,0.6));
#30168=CARTESIAN_POINT('',(-0.144337567297406,0.25,0.6));
#30169=CARTESIAN_POINT('',(-0.0721687836487032,0.25,0.6));
#30170=CARTESIAN_POINT('',(-0.144337567297406,0.25,0.3));
#30171=CARTESIAN_POINT('',(-0.144337567297406,0.25,0.6));
#30172=CARTESIAN_POINT('',(0.144337567297406,0.25,0.3));
#30173=CARTESIAN_POINT('Origin',(-0.288675134594813,5.55111512312578E-17,
0.6));
#30174=CARTESIAN_POINT('',(-0.288675134594813,3.53525079574969E-17,0.6));
#30175=CARTESIAN_POINT('',(-0.252590742770461,0.0625000000000001,0.6));
#30176=CARTESIAN_POINT('',(-0.288675134594813,5.55111512312578E-17,0.3));
#30177=CARTESIAN_POINT('',(-0.288675134594813,3.53525079574969E-17,0.6));
#30178=CARTESIAN_POINT('',(-0.144337567297406,0.25,0.3));
#30179=CARTESIAN_POINT('Origin',(-0.144337567297407,-0.25,0.6));
#30180=CARTESIAN_POINT('',(-0.144337567297407,-0.25,0.6));
#30181=CARTESIAN_POINT('',(-0.180421959121758,-0.1875,0.6));
#30182=CARTESIAN_POINT('',(-0.144337567297407,-0.25,0.3));
#30183=CARTESIAN_POINT('',(-0.144337567297407,-0.25,0.6));
#30184=CARTESIAN_POINT('',(-0.288675134594813,3.53525079574969E-17,0.3));
#30185=CARTESIAN_POINT('Origin',(0.144337567297406,-0.25,0.6));
#30186=CARTESIAN_POINT('',(0.144337567297406,-0.25,0.6));
#30187=CARTESIAN_POINT('',(0.0721687836487032,-0.25,0.6));
#30188=CARTESIAN_POINT('',(0.144337567297406,-0.25,0.3));
#30189=CARTESIAN_POINT('',(0.144337567297406,-0.25,0.6));
#30190=CARTESIAN_POINT('',(-0.144337567297407,-0.25,0.3));
#30191=CARTESIAN_POINT('Origin',(0.288675134594813,0.,0.6));
#30192=CARTESIAN_POINT('',(0.252590742770461,-0.0625,0.6));
#30193=CARTESIAN_POINT('',(0.144337567297406,-0.25,0.3));
#30194=CARTESIAN_POINT('Origin',(0.,0.,0.3));
#30195=CARTESIAN_POINT('Origin',(0.497072620864318,-0.210994809384208,0.56));
#30196=CARTESIAN_POINT('',(0.466514061501753,-0.179901724341759,0.1));
#30197=CARTESIAN_POINT('',(0.466514061501753,-0.179901724341759,0.56));
#30198=CARTESIAN_POINT('',(0.466514061501753,-0.179901724341759,0.29));
#30199=CARTESIAN_POINT('',(0.451052457977236,-0.164169668796321,0.1));
#30200=CARTESIAN_POINT('',(0.497072620864318,-0.210994809384208,0.1));
#30201=CARTESIAN_POINT('',(0.451052457977236,-0.164169668796321,0.56));
#30202=CARTESIAN_POINT('',(0.451052457977236,-0.164169668796321,0.56));
#30203=CARTESIAN_POINT('',(0.497072620864318,-0.210994809384208,0.56));
#30204=CARTESIAN_POINT('Origin',(0.483728513098638,-0.184437764967243,0.56));
#30205=CARTESIAN_POINT('',(0.473009103818409,-0.162056742238344,0.56));
#30206=CARTESIAN_POINT('Origin',(0.,0.,0.56));
#30207=CARTESIAN_POINT('',(0.451052457977236,-0.164169668796321,0.56));
#30208=CARTESIAN_POINT('Origin',(0.451052457977236,-0.164169668796321,0.56));
#30209=CARTESIAN_POINT('',(0.473009103818409,-0.162056742238344,0.1));
#30210=CARTESIAN_POINT('',(0.473009103818409,-0.162056742238344,0.29));
#30211=CARTESIAN_POINT('',(0.451052457977236,-0.164169668796321,0.1));
#30212=CARTESIAN_POINT('Origin',(0.483728513098638,-0.184437764967243,0.1));
#30213=CARTESIAN_POINT('Origin',(0.,0.,0.1));
#30214=CARTESIAN_POINT('Origin',(0.394930998874352,-0.368279114433749,0.56));
#30215=CARTESIAN_POINT('',(0.376849807542158,-0.328609529008881,0.1));
#30216=CARTESIAN_POINT('',(0.376849807542158,-0.328609529008881,0.56));
#30217=CARTESIAN_POINT('',(0.376849807542158,-0.328609529008881,0.29));
#30218=CARTESIAN_POINT('',(0.367701332697109,-0.308538052649539,0.1));
#30219=CARTESIAN_POINT('',(0.394930998874352,-0.368279114433749,0.1));
#30220=CARTESIAN_POINT('',(0.367701332697109,-0.308538052649539,0.56));
#30221=CARTESIAN_POINT('',(0.367701332697109,-0.308538052649539,0.56));
#30222=CARTESIAN_POINT('',(0.394930998874352,-0.368279114433749,0.56));
#30223=CARTESIAN_POINT('Origin',(0.399482254061324,-0.338408583541644,0.56));
#30224=CARTESIAN_POINT('',(0.389056494215466,-0.314062166312295,0.56));
#30225=CARTESIAN_POINT('Origin',(0.,0.,0.56));
#30226=CARTESIAN_POINT('',(0.367701332697109,-0.308538052649539,0.56));
#30227=CARTESIAN_POINT('Origin',(0.367701332697109,-0.308538052649539,0.56));
#30228=CARTESIAN_POINT('',(0.389056494215466,-0.314062166312295,0.1));
#30229=CARTESIAN_POINT('',(0.389056494215466,-0.314062166312295,0.29));
#30230=CARTESIAN_POINT('',(0.367701332697109,-0.308538052649539,0.1));
#30231=CARTESIAN_POINT('Origin',(0.399482254061324,-0.338408583541644,0.1));
#30232=CARTESIAN_POINT('Origin',(0.,0.,0.1));
#30233=CARTESIAN_POINT('Origin',(0.245154869859355,-0.481143523061719,0.56));
#30234=CARTESIAN_POINT('',(0.241731905082157,-0.437682174717398,0.1));
#30235=CARTESIAN_POINT('',(0.241731905082157,-0.437682174717398,0.56));
#30236=CARTESIAN_POINT('',(0.241731905082157,-0.437682174717398,0.29));
#30237=CARTESIAN_POINT('',(0.24,-0.41569219381653,0.1));
#30238=CARTESIAN_POINT('',(0.245154869859355,-0.481143523061719,0.1));
#30239=CARTESIAN_POINT('',(0.24,-0.41569219381653,0.56));
#30240=CARTESIAN_POINT('',(0.24,-0.41569219381653,0.56));
#30241=CARTESIAN_POINT('',(0.245154869859355,-0.481143523061719,0.56));
#30242=CARTESIAN_POINT('Origin',(0.267052539454057,-0.448417858439125,0.56));
#30243=CARTESIAN_POINT('',(0.258177929547807,-0.428187058065056,0.56));
#30244=CARTESIAN_POINT('Origin',(0.,0.,0.56));
#30245=CARTESIAN_POINT('',(0.24,-0.41569219381653,0.56));
#30246=CARTESIAN_POINT('Origin',(0.24,-0.41569219381653,0.56));
#30247=CARTESIAN_POINT('',(0.258177929547807,-0.428187058065056,0.1));
#30248=CARTESIAN_POINT('',(0.258177929547807,-0.428187058065056,0.29));
#30249=CARTESIAN_POINT('',(0.24,-0.41569219381653,0.1));
#30250=CARTESIAN_POINT('Origin',(0.267052539454057,-0.448417858439125,0.1));
#30251=CARTESIAN_POINT('Origin',(0.,0.,0.1));
#30252=CARTESIAN_POINT('Origin',(0.0658094454387798,-0.535974921886314,
0.56));
#30253=CARTESIAN_POINT('',(0.0774575672862877,-0.493963890654054,0.1));
#30254=CARTESIAN_POINT('',(0.0774575672862877,-0.493963890654054,0.56));
#30255=CARTESIAN_POINT('',(0.0774575672862877,-0.493963890654054,0.29));
#30256=CARTESIAN_POINT('',(0.0833511252801264,-0.47270772144586,0.1));
#30257=CARTESIAN_POINT('',(0.0658094454387798,-0.535974921886314,0.1));
#30258=CARTESIAN_POINT('',(0.0833511252801264,-0.47270772144586,0.56));
#30259=CARTESIAN_POINT('',(0.0833511252801264,-0.47270772144586,0.56));
#30260=CARTESIAN_POINT('',(0.0658094454387798,-0.535974921886314,0.56));
#30261=CARTESIAN_POINT('Origin',(0.0936415073922334,-0.504341321666087,
0.56));
#30262=CARTESIAN_POINT('',(0.0961592962762517,-0.490666271247226,0.56));
#30263=CARTESIAN_POINT('Origin',(0.,0.,0.56));
#30264=CARTESIAN_POINT('',(0.0833511252801264,-0.47270772144586,0.56));
#30265=CARTESIAN_POINT('Origin',(0.0833511252801264,-0.47270772144586,0.56));
#30266=CARTESIAN_POINT('',(0.0961592962762517,-0.490666271247226,0.1));
#30267=CARTESIAN_POINT('',(0.0961592962762517,-0.490666271247226,0.29));
#30268=CARTESIAN_POINT('',(0.0833511252801264,-0.47270772144586,0.1));
#30269=CARTESIAN_POINT('Origin',(0.0936415073922334,-0.504341321666087,
0.1));
#30270=CARTESIAN_POINT('Origin',(0.,0.,0.1));
#30271=CARTESIAN_POINT('Origin',(-0.121473569345687,-0.526159834984027,
0.56));
#30272=CARTESIAN_POINT('',(-0.0961592962762519,-0.490666271247226,0.1));
#30273=CARTESIAN_POINT('',(-0.0961592962762519,-0.490666271247226,0.56));
#30274=CARTESIAN_POINT('',(-0.0961592962762519,-0.490666271247226,0.29));
#30275=CARTESIAN_POINT('',(-0.0833511252801266,-0.47270772144586,0.1));
#30276=CARTESIAN_POINT('',(-0.121473569345687,-0.526159834984027,0.1));
#30277=CARTESIAN_POINT('',(-0.0833511252801266,-0.47270772144586,0.56));
#30278=CARTESIAN_POINT('',(-0.0833511252801266,-0.47270772144586,0.56));
#30279=CARTESIAN_POINT('',(-0.121473569345687,-0.526159834984027,0.56));
#30280=CARTESIAN_POINT('Origin',(-0.0936415073922334,-0.504341321666087,
0.56));
#30281=CARTESIAN_POINT('',(-0.0774575672862877,-0.493963890654054,0.56));
#30282=CARTESIAN_POINT('Origin',(0.,0.,0.56));
#30283=CARTESIAN_POINT('',(-0.0833511252801266,-0.47270772144586,0.56));
#30284=CARTESIAN_POINT('Origin',(-0.0833511252801266,-0.47270772144586,
0.56));
#30285=CARTESIAN_POINT('',(-0.0774575672862877,-0.493963890654054,0.1));
#30286=CARTESIAN_POINT('',(-0.0774575672862877,-0.493963890654054,0.29));
#30287=CARTESIAN_POINT('',(-0.0833511252801266,-0.47270772144586,0.1));
#30288=CARTESIAN_POINT('Origin',(-0.0936415073922334,-0.504341321666087,
0.1));
#30289=CARTESIAN_POINT('Origin',(0.,0.,0.1));
#30290=CARTESIAN_POINT('Origin',(-0.294105078908115,-0.452882106690529,
0.56));
#30291=CARTESIAN_POINT('',(-0.258177929547807,-0.428187058065056,0.1));
#30292=CARTESIAN_POINT('',(-0.258177929547807,-0.428187058065056,0.56));
#30293=CARTESIAN_POINT('',(-0.258177929547807,-0.428187058065056,0.29));
#30294=CARTESIAN_POINT('',(-0.24,-0.41569219381653,0.1));
#30295=CARTESIAN_POINT('',(-0.294105078908115,-0.452882106690529,0.1));
#30296=CARTESIAN_POINT('',(-0.24,-0.41569219381653,0.56));
#30297=CARTESIAN_POINT('',(-0.24,-0.41569219381653,0.56));
#30298=CARTESIAN_POINT('',(-0.294105078908115,-0.452882106690529,0.56));
#30299=CARTESIAN_POINT('Origin',(-0.267052539454057,-0.448417858439125,
0.56));
#30300=CARTESIAN_POINT('',(-0.241731905082157,-0.437682174717398,0.56));
#30301=CARTESIAN_POINT('Origin',(0.,0.,0.56));
#30302=CARTESIAN_POINT('',(-0.24,-0.41569219381653,0.56));
#30303=CARTESIAN_POINT('Origin',(-0.24,-0.41569219381653,0.56));
#30304=CARTESIAN_POINT('',(-0.241731905082157,-0.437682174717398,0.1));
#30305=CARTESIAN_POINT('',(-0.241731905082157,-0.437682174717398,0.29));
#30306=CARTESIAN_POINT('',(-0.24,-0.41569219381653,0.1));
#30307=CARTESIAN_POINT('Origin',(-0.267052539454057,-0.448417858439125,
0.1));
#30308=CARTESIAN_POINT('Origin',(0.,0.,0.1));
#30309=CARTESIAN_POINT('Origin',(-0.431263175425538,-0.324980112502106,
0.56));
#30310=CARTESIAN_POINT('',(-0.389056494215466,-0.314062166312295,0.1));
#30311=CARTESIAN_POINT('',(-0.389056494215466,-0.314062166312295,0.56));
#30312=CARTESIAN_POINT('',(-0.389056494215466,-0.314062166312295,0.29));
#30313=CARTESIAN_POINT('',(-0.367701332697109,-0.308538052649539,0.1));
#30314=CARTESIAN_POINT('',(-0.431263175425538,-0.324980112502106,0.1));
#30315=CARTESIAN_POINT('',(-0.367701332697109,-0.308538052649539,0.56));
#30316=CARTESIAN_POINT('',(-0.367701332697109,-0.308538052649539,0.56));
#30317=CARTESIAN_POINT('',(-0.431263175425538,-0.324980112502106,0.56));
#30318=CARTESIAN_POINT('Origin',(-0.399482254061324,-0.338408583541644,
0.56));
#30319=CARTESIAN_POINT('',(-0.376849807542158,-0.328609529008881,0.56));
#30320=CARTESIAN_POINT('Origin',(0.,0.,0.56));
#30321=CARTESIAN_POINT('',(-0.367701332697109,-0.308538052649539,0.56));
#30322=CARTESIAN_POINT('Origin',(-0.367701332697109,-0.308538052649539,
0.56));
#30323=CARTESIAN_POINT('',(-0.376849807542158,-0.328609529008881,0.1));
#30324=CARTESIAN_POINT('',(-0.376849807542158,-0.328609529008881,0.29));
#30325=CARTESIAN_POINT('',(-0.367701332697109,-0.308538052649539,0.1));
#30326=CARTESIAN_POINT('Origin',(-0.399482254061324,-0.338408583541644,
0.1));
#30327=CARTESIAN_POINT('Origin',(0.,0.,0.1));
#30328=CARTESIAN_POINT('Origin',(-0.516404568220039,-0.157880720550278,
0.56));
#30329=CARTESIAN_POINT('',(-0.473009103818409,-0.162056742238344,0.1));
#30330=CARTESIAN_POINT('',(-0.473009103818409,-0.162056742238344,0.56));
#30331=CARTESIAN_POINT('',(-0.473009103818409,-0.162056742238344,0.29));
#30332=CARTESIAN_POINT('',(-0.451052457977236,-0.164169668796321,0.1));
#30333=CARTESIAN_POINT('',(-0.516404568220039,-0.157880720550278,0.1));
#30334=CARTESIAN_POINT('',(-0.451052457977236,-0.164169668796321,0.56));
#30335=CARTESIAN_POINT('',(-0.451052457977236,-0.164169668796321,0.56));
#30336=CARTESIAN_POINT('',(-0.516404568220039,-0.157880720550278,0.56));
#30337=CARTESIAN_POINT('Origin',(-0.483728513098638,-0.184437764967243,
0.56));
#30338=CARTESIAN_POINT('',(-0.466514061501753,-0.179901724341759,0.56));
#30339=CARTESIAN_POINT('Origin',(0.,0.,0.56));
#30340=CARTESIAN_POINT('',(-0.451052457977236,-0.164169668796321,0.56));
#30341=CARTESIAN_POINT('Origin',(-0.451052457977236,-0.164169668796321,
0.56));
#30342=CARTESIAN_POINT('',(-0.466514061501753,-0.179901724341759,0.1));
#30343=CARTESIAN_POINT('',(-0.466514061501753,-0.179901724341759,0.29));
#30344=CARTESIAN_POINT('',(-0.451052457977236,-0.164169668796321,0.1));
#30345=CARTESIAN_POINT('Origin',(-0.483728513098638,-0.184437764967243,
0.1));
#30346=CARTESIAN_POINT('Origin',(0.,0.,0.1));
#30347=CARTESIAN_POINT('Origin',(-0.53925994876747,0.0282614163711897,0.56));
#30348=CARTESIAN_POINT('',(-0.499909834629965,0.00949511665234234,0.1));
#30349=CARTESIAN_POINT('',(-0.499909834629965,0.00949511665234234,0.56));
#30350=CARTESIAN_POINT('',(-0.499909834629965,0.00949511665234234,0.29));
#30351=CARTESIAN_POINT('',(-0.48,5.87830463590729E-17,0.1));
#30352=CARTESIAN_POINT('',(-0.53925994876747,0.0282614163711897,0.1));
#30353=CARTESIAN_POINT('',(-0.48,5.87830463590729E-17,0.56));
#30354=CARTESIAN_POINT('',(-0.48,5.87830463590729E-17,0.56));
#30355=CARTESIAN_POINT('',(-0.53925994876747,0.0282614163711897,0.56));
#30356=CARTESIAN_POINT('Origin',(-0.509629974383735,6.59194920871187E-17,
0.56));
#30357=CARTESIAN_POINT('',(-0.5,-6.12323399573677E-17,0.56));
#30358=CARTESIAN_POINT('Origin',(0.,0.,0.56));
#30359=CARTESIAN_POINT('',(-0.499909834629965,-0.00949511665234226,0.56));
#30360=CARTESIAN_POINT('',(-0.48,5.87830463590729E-17,0.56));
#30361=CARTESIAN_POINT('Origin',(0.,0.,0.56));
#30362=CARTESIAN_POINT('Origin',(-0.48,5.87830463590729E-17,0.56));
#30363=CARTESIAN_POINT('',(-0.499909834629965,-0.00949511665234226,0.1));
#30364=CARTESIAN_POINT('',(-0.499909834629965,-0.00949511665234226,0.29));
#30365=CARTESIAN_POINT('',(-0.48,5.87830463590729E-17,0.1));
#30366=CARTESIAN_POINT('Origin',(-0.509629974383735,6.59194920871187E-17,
0.1));
#30367=CARTESIAN_POINT('',(-0.5,-6.12323399573677E-17,0.1));
#30368=CARTESIAN_POINT('Origin',(0.,0.,0.1));
#30369=CARTESIAN_POINT('Origin',(0.,0.,0.1));
#30370=CARTESIAN_POINT('Origin',(-0.526159834984027,0.121473569345687,0.56));
#30371=CARTESIAN_POINT('',(-0.490666271247226,0.0961592962762519,0.1));
#30372=CARTESIAN_POINT('',(-0.490666271247226,0.0961592962762519,0.56));
#30373=CARTESIAN_POINT('',(-0.490666271247226,0.0961592962762519,0.29));
#30374=CARTESIAN_POINT('',(-0.47270772144586,0.0833511252801265,0.1));
#30375=CARTESIAN_POINT('',(-0.526159834984027,0.121473569345687,0.1));
#30376=CARTESIAN_POINT('',(-0.47270772144586,0.0833511252801265,0.56));
#30377=CARTESIAN_POINT('',(-0.47270772144586,0.0833511252801265,0.56));
#30378=CARTESIAN_POINT('',(-0.526159834984027,0.121473569345687,0.56));
#30379=CARTESIAN_POINT('Origin',(-0.504341321666087,0.0936415073922334,
0.56));
#30380=CARTESIAN_POINT('',(-0.493963890654054,0.0774575672862877,0.56));
#30381=CARTESIAN_POINT('Origin',(0.,0.,0.56));
#30382=CARTESIAN_POINT('',(-0.47270772144586,0.0833511252801265,0.56));
#30383=CARTESIAN_POINT('Origin',(-0.47270772144586,0.0833511252801265,0.56));
#30384=CARTESIAN_POINT('',(-0.493963890654054,0.0774575672862877,0.1));
#30385=CARTESIAN_POINT('',(-0.493963890654054,0.0774575672862877,0.29));
#30386=CARTESIAN_POINT('',(-0.47270772144586,0.0833511252801265,0.1));
#30387=CARTESIAN_POINT('Origin',(-0.504341321666087,0.0936415073922334,
0.1));
#30388=CARTESIAN_POINT('Origin',(0.,0.,0.1));
#30389=CARTESIAN_POINT('Origin',(-0.452882106690529,0.294105078908115,0.56));
#30390=CARTESIAN_POINT('',(-0.428187058065056,0.258177929547807,0.1));
#30391=CARTESIAN_POINT('',(-0.428187058065056,0.258177929547807,0.56));
#30392=CARTESIAN_POINT('',(-0.428187058065056,0.258177929547807,0.29));
#30393=CARTESIAN_POINT('',(-0.415692193816531,0.24,0.1));
#30394=CARTESIAN_POINT('',(-0.452882106690529,0.294105078908115,0.1));
#30395=CARTESIAN_POINT('',(-0.415692193816531,0.24,0.56));
#30396=CARTESIAN_POINT('',(-0.415692193816531,0.24,0.56));
#30397=CARTESIAN_POINT('',(-0.452882106690529,0.294105078908115,0.56));
#30398=CARTESIAN_POINT('Origin',(-0.448417858439125,0.267052539454057,0.56));
#30399=CARTESIAN_POINT('',(-0.437682174717398,0.241731905082157,0.56));
#30400=CARTESIAN_POINT('Origin',(0.,0.,0.56));
#30401=CARTESIAN_POINT('',(-0.415692193816531,0.24,0.56));
#30402=CARTESIAN_POINT('Origin',(-0.415692193816531,0.24,0.56));
#30403=CARTESIAN_POINT('',(-0.437682174717398,0.241731905082157,0.1));
#30404=CARTESIAN_POINT('',(-0.437682174717398,0.241731905082157,0.29));
#30405=CARTESIAN_POINT('',(-0.415692193816531,0.24,0.1));
#30406=CARTESIAN_POINT('Origin',(-0.448417858439125,0.267052539454057,0.1));
#30407=CARTESIAN_POINT('Origin',(0.,0.,0.1));
#30408=CARTESIAN_POINT('Origin',(-0.324980112502106,0.431263175425538,0.56));
#30409=CARTESIAN_POINT('',(-0.314062166312295,0.389056494215465,0.1));
#30410=CARTESIAN_POINT('',(-0.314062166312295,0.389056494215465,0.56));
#30411=CARTESIAN_POINT('',(-0.314062166312295,0.389056494215465,0.29));
#30412=CARTESIAN_POINT('',(-0.308538052649539,0.367701332697109,0.1));
#30413=CARTESIAN_POINT('',(-0.324980112502106,0.431263175425538,0.1));
#30414=CARTESIAN_POINT('',(-0.308538052649539,0.367701332697109,0.56));
#30415=CARTESIAN_POINT('',(-0.308538052649539,0.367701332697109,0.56));
#30416=CARTESIAN_POINT('',(-0.324980112502106,0.431263175425538,0.56));
#30417=CARTESIAN_POINT('Origin',(-0.338408583541644,0.399482254061324,0.56));
#30418=CARTESIAN_POINT('',(-0.328609529008881,0.376849807542158,0.56));
#30419=CARTESIAN_POINT('Origin',(0.,0.,0.56));
#30420=CARTESIAN_POINT('',(-0.308538052649539,0.367701332697109,0.56));
#30421=CARTESIAN_POINT('Origin',(-0.308538052649539,0.367701332697109,0.56));
#30422=CARTESIAN_POINT('',(-0.328609529008881,0.376849807542158,0.1));
#30423=CARTESIAN_POINT('',(-0.328609529008881,0.376849807542158,0.29));
#30424=CARTESIAN_POINT('',(-0.308538052649539,0.367701332697109,0.1));
#30425=CARTESIAN_POINT('Origin',(-0.338408583541644,0.399482254061324,0.1));
#30426=CARTESIAN_POINT('Origin',(0.,0.,0.1));
#30427=CARTESIAN_POINT('Origin',(-0.157880720550278,0.516404568220039,0.56));
#30428=CARTESIAN_POINT('',(-0.162056742238344,0.473009103818409,0.1));
#30429=CARTESIAN_POINT('',(-0.162056742238344,0.473009103818409,0.56));
#30430=CARTESIAN_POINT('',(-0.162056742238344,0.473009103818409,0.29));
#30431=CARTESIAN_POINT('',(-0.164169668796321,0.451052457977236,0.1));
#30432=CARTESIAN_POINT('',(-0.157880720550278,0.516404568220039,0.1));
#30433=CARTESIAN_POINT('',(-0.164169668796321,0.451052457977236,0.56));
#30434=CARTESIAN_POINT('',(-0.164169668796321,0.451052457977236,0.56));
#30435=CARTESIAN_POINT('',(-0.157880720550278,0.516404568220039,0.56));
#30436=CARTESIAN_POINT('Origin',(-0.184437764967243,0.483728513098638,0.56));
#30437=CARTESIAN_POINT('',(-0.179901724341759,0.466514061501753,0.56));
#30438=CARTESIAN_POINT('Origin',(0.,0.,0.56));
#30439=CARTESIAN_POINT('',(-0.164169668796321,0.451052457977236,0.56));
#30440=CARTESIAN_POINT('Origin',(-0.164169668796321,0.451052457977236,0.56));
#30441=CARTESIAN_POINT('',(-0.179901724341759,0.466514061501753,0.1));
#30442=CARTESIAN_POINT('',(-0.179901724341759,0.466514061501753,0.29));
#30443=CARTESIAN_POINT('',(-0.164169668796321,0.451052457977236,0.1));
#30444=CARTESIAN_POINT('Origin',(-0.184437764967243,0.483728513098638,0.1));
#30445=CARTESIAN_POINT('Origin',(0.,0.,0.1));
#30446=CARTESIAN_POINT('Origin',(0.0282614163711897,0.53925994876747,0.56));
#30447=CARTESIAN_POINT('',(0.00949511665234237,0.499909834629964,0.1));
#30448=CARTESIAN_POINT('',(0.00949511665234237,0.499909834629964,0.56));
#30449=CARTESIAN_POINT('',(0.00949511665234237,0.499909834629964,0.29));
#30450=CARTESIAN_POINT('',(2.93915231795365E-17,0.48,0.1));
#30451=CARTESIAN_POINT('',(0.0282614163711897,0.53925994876747,0.1));
#30452=CARTESIAN_POINT('',(2.93915231795365E-17,0.48,0.56));
#30453=CARTESIAN_POINT('',(2.93915231795365E-17,0.48,0.56));
#30454=CARTESIAN_POINT('',(0.0282614163711897,0.53925994876747,0.56));
#30455=CARTESIAN_POINT('Origin',(3.46944695195361E-17,0.509629974383735,
0.56));
#30456=CARTESIAN_POINT('',(-0.00949511665234229,0.499909834629964,0.56));
#30457=CARTESIAN_POINT('Origin',(0.,0.,0.56));
#30458=CARTESIAN_POINT('',(2.93915231795365E-17,0.48,0.56));
#30459=CARTESIAN_POINT('Origin',(2.93915231795365E-17,0.48,0.56));
#30460=CARTESIAN_POINT('',(-0.00949511665234229,0.499909834629964,0.1));
#30461=CARTESIAN_POINT('',(-0.00949511665234229,0.499909834629964,0.29));
#30462=CARTESIAN_POINT('',(2.93915231795365E-17,0.48,0.1));
#30463=CARTESIAN_POINT('Origin',(3.46944695195361E-17,0.509629974383735,
0.1));
#30464=CARTESIAN_POINT('Origin',(0.,0.,0.1));
#30465=CARTESIAN_POINT('Origin',(0.210994809384208,0.497072620864318,0.56));
#30466=CARTESIAN_POINT('',(0.179901724341759,0.466514061501753,0.1));
#30467=CARTESIAN_POINT('',(0.179901724341759,0.466514061501753,0.56));
#30468=CARTESIAN_POINT('',(0.179901724341759,0.466514061501753,0.29));
#30469=CARTESIAN_POINT('',(0.164169668796321,0.451052457977236,0.1));
#30470=CARTESIAN_POINT('',(0.210994809384208,0.497072620864318,0.1));
#30471=CARTESIAN_POINT('',(0.164169668796321,0.451052457977236,0.56));
#30472=CARTESIAN_POINT('',(0.164169668796321,0.451052457977236,0.56));
#30473=CARTESIAN_POINT('',(0.210994809384208,0.497072620864318,0.56));
#30474=CARTESIAN_POINT('Origin',(0.184437764967243,0.483728513098638,0.56));
#30475=CARTESIAN_POINT('',(0.162056742238344,0.473009103818409,0.56));
#30476=CARTESIAN_POINT('Origin',(0.,0.,0.56));
#30477=CARTESIAN_POINT('',(0.164169668796321,0.451052457977236,0.56));
#30478=CARTESIAN_POINT('Origin',(0.164169668796321,0.451052457977236,0.56));
#30479=CARTESIAN_POINT('',(0.162056742238344,0.473009103818409,0.1));
#30480=CARTESIAN_POINT('',(0.162056742238344,0.473009103818409,0.29));
#30481=CARTESIAN_POINT('',(0.164169668796321,0.451052457977236,0.1));
#30482=CARTESIAN_POINT('Origin',(0.184437764967243,0.483728513098638,0.1));
#30483=CARTESIAN_POINT('Origin',(0.,0.,0.1));
#30484=CARTESIAN_POINT('Origin',(0.368279114433749,0.394930998874352,0.56));
#30485=CARTESIAN_POINT('',(0.328609529008881,0.376849807542157,0.1));
#30486=CARTESIAN_POINT('',(0.328609529008881,0.376849807542157,0.56));
#30487=CARTESIAN_POINT('',(0.328609529008881,0.376849807542157,0.29));
#30488=CARTESIAN_POINT('',(0.308538052649539,0.367701332697109,0.1));
#30489=CARTESIAN_POINT('',(0.368279114433749,0.394930998874352,0.1));
#30490=CARTESIAN_POINT('',(0.308538052649539,0.367701332697109,0.56));
#30491=CARTESIAN_POINT('',(0.308538052649539,0.367701332697109,0.56));
#30492=CARTESIAN_POINT('',(0.368279114433749,0.394930998874352,0.56));
#30493=CARTESIAN_POINT('Origin',(0.338408583541644,0.399482254061324,0.56));
#30494=CARTESIAN_POINT('',(0.314062166312295,0.389056494215466,0.56));
#30495=CARTESIAN_POINT('Origin',(0.,0.,0.56));
#30496=CARTESIAN_POINT('',(0.308538052649539,0.367701332697109,0.56));
#30497=CARTESIAN_POINT('Origin',(0.308538052649539,0.367701332697109,0.56));
#30498=CARTESIAN_POINT('',(0.314062166312295,0.389056494215466,0.1));
#30499=CARTESIAN_POINT('',(0.314062166312295,0.389056494215466,0.29));
#30500=CARTESIAN_POINT('',(0.308538052649539,0.367701332697109,0.1));
#30501=CARTESIAN_POINT('Origin',(0.338408583541644,0.399482254061324,0.1));
#30502=CARTESIAN_POINT('Origin',(0.,0.,0.1));
#30503=CARTESIAN_POINT('Origin',(0.481143523061719,0.245154869859355,0.56));
#30504=CARTESIAN_POINT('',(0.437682174717398,0.241731905082157,0.1));
#30505=CARTESIAN_POINT('',(0.437682174717398,0.241731905082157,0.56));
#30506=CARTESIAN_POINT('',(0.437682174717398,0.241731905082157,0.29));
#30507=CARTESIAN_POINT('',(0.415692193816531,0.24,0.1));
#30508=CARTESIAN_POINT('',(0.481143523061719,0.245154869859355,0.1));
#30509=CARTESIAN_POINT('',(0.415692193816531,0.24,0.56));
#30510=CARTESIAN_POINT('',(0.415692193816531,0.24,0.56));
#30511=CARTESIAN_POINT('',(0.481143523061719,0.245154869859355,0.56));
#30512=CARTESIAN_POINT('Origin',(0.448417858439125,0.267052539454057,0.56));
#30513=CARTESIAN_POINT('',(0.428187058065056,0.258177929547807,0.56));
#30514=CARTESIAN_POINT('Origin',(0.,0.,0.56));
#30515=CARTESIAN_POINT('',(0.415692193816531,0.24,0.56));
#30516=CARTESIAN_POINT('Origin',(0.415692193816531,0.24,0.56));
#30517=CARTESIAN_POINT('',(0.428187058065056,0.258177929547807,0.1));
#30518=CARTESIAN_POINT('',(0.428187058065056,0.258177929547807,0.29));
#30519=CARTESIAN_POINT('',(0.415692193816531,0.24,0.1));
#30520=CARTESIAN_POINT('Origin',(0.448417858439125,0.267052539454057,0.1));
#30521=CARTESIAN_POINT('Origin',(0.,0.,0.1));
#30522=CARTESIAN_POINT('Origin',(0.535974921886314,0.0658094454387796,0.56));
#30523=CARTESIAN_POINT('',(0.493963890654054,0.0774575672862878,0.1));
#30524=CARTESIAN_POINT('',(0.493963890654054,0.0774575672862878,0.56));
#30525=CARTESIAN_POINT('',(0.493963890654054,0.0774575672862878,0.29));
#30526=CARTESIAN_POINT('',(0.47270772144586,0.0833511252801266,0.1));
#30527=CARTESIAN_POINT('',(0.535974921886314,0.0658094454387796,0.1));
#30528=CARTESIAN_POINT('',(0.47270772144586,0.0833511252801266,0.56));
#30529=CARTESIAN_POINT('',(0.47270772144586,0.0833511252801266,0.56));
#30530=CARTESIAN_POINT('',(0.535974921886314,0.0658094454387796,0.56));
#30531=CARTESIAN_POINT('Origin',(0.504341321666087,0.0936415073922334,0.56));
#30532=CARTESIAN_POINT('',(0.490666271247226,0.0961592962762519,0.56));
#30533=CARTESIAN_POINT('Origin',(0.,0.,0.56));
#30534=CARTESIAN_POINT('',(0.47270772144586,0.0833511252801266,0.56));
#30535=CARTESIAN_POINT('Origin',(0.47270772144586,0.0833511252801266,0.56));
#30536=CARTESIAN_POINT('',(0.490666271247226,0.0961592962762519,0.1));
#30537=CARTESIAN_POINT('',(0.490666271247226,0.0961592962762519,0.29));
#30538=CARTESIAN_POINT('',(0.47270772144586,0.0833511252801266,0.1));
#30539=CARTESIAN_POINT('Origin',(0.504341321666087,0.0936415073922334,0.1));
#30540=CARTESIAN_POINT('Origin',(0.,0.,0.1));
#30541=CARTESIAN_POINT('Origin',(0.516404568220039,0.157880720550278,0.56));
#30542=CARTESIAN_POINT('',(0.473009103818409,0.162056742238344,0.1));
#30543=CARTESIAN_POINT('',(0.473009103818409,0.162056742238344,0.56));
#30544=CARTESIAN_POINT('',(0.473009103818409,0.162056742238344,0.29));
#30545=CARTESIAN_POINT('',(0.451052457977236,0.164169668796321,0.1));
#30546=CARTESIAN_POINT('',(0.516404568220039,0.157880720550278,0.1));
#30547=CARTESIAN_POINT('',(0.451052457977236,0.164169668796321,0.56));
#30548=CARTESIAN_POINT('',(0.451052457977236,0.164169668796321,0.56));
#30549=CARTESIAN_POINT('',(0.516404568220039,0.157880720550278,0.56));
#30550=CARTESIAN_POINT('Origin',(0.483728513098638,0.184437764967243,0.56));
#30551=CARTESIAN_POINT('',(0.466514061501753,0.179901724341759,0.56));
#30552=CARTESIAN_POINT('Origin',(0.,0.,0.56));
#30553=CARTESIAN_POINT('',(0.451052457977236,0.164169668796321,0.56));
#30554=CARTESIAN_POINT('Origin',(0.451052457977236,0.164169668796321,0.56));
#30555=CARTESIAN_POINT('',(0.466514061501753,0.179901724341759,0.1));
#30556=CARTESIAN_POINT('',(0.466514061501753,0.179901724341759,0.29));
#30557=CARTESIAN_POINT('',(0.451052457977236,0.164169668796321,0.1));
#30558=CARTESIAN_POINT('Origin',(0.483728513098638,0.184437764967243,0.1));
#30559=CARTESIAN_POINT('Origin',(0.,0.,0.1));
#30560=CARTESIAN_POINT('Origin',(0.431263175425538,0.324980112502106,0.56));
#30561=CARTESIAN_POINT('',(0.389056494215466,0.314062166312295,0.1));
#30562=CARTESIAN_POINT('',(0.389056494215466,0.314062166312295,0.56));
#30563=CARTESIAN_POINT('',(0.389056494215466,0.314062166312295,0.29));
#30564=CARTESIAN_POINT('',(0.367701332697109,0.308538052649539,0.1));
#30565=CARTESIAN_POINT('',(0.431263175425538,0.324980112502106,0.1));
#30566=CARTESIAN_POINT('',(0.367701332697109,0.308538052649539,0.56));
#30567=CARTESIAN_POINT('',(0.367701332697109,0.308538052649539,0.56));
#30568=CARTESIAN_POINT('',(0.431263175425538,0.324980112502106,0.56));
#30569=CARTESIAN_POINT('Origin',(0.399482254061324,0.338408583541644,0.56));
#30570=CARTESIAN_POINT('',(0.376849807542158,0.328609529008881,0.56));
#30571=CARTESIAN_POINT('Origin',(0.,0.,0.56));
#30572=CARTESIAN_POINT('',(0.367701332697109,0.308538052649539,0.56));
#30573=CARTESIAN_POINT('Origin',(0.367701332697109,0.308538052649539,0.56));
#30574=CARTESIAN_POINT('',(0.376849807542158,0.328609529008881,0.1));
#30575=CARTESIAN_POINT('',(0.376849807542158,0.328609529008881,0.29));
#30576=CARTESIAN_POINT('',(0.367701332697109,0.308538052649539,0.1));
#30577=CARTESIAN_POINT('Origin',(0.399482254061324,0.338408583541644,0.1));
#30578=CARTESIAN_POINT('Origin',(0.,0.,0.1));
#30579=CARTESIAN_POINT('Origin',(0.294105078908115,0.452882106690529,0.56));
#30580=CARTESIAN_POINT('',(0.258177929547807,0.428187058065056,0.1));
#30581=CARTESIAN_POINT('',(0.258177929547807,0.428187058065056,0.56));
#30582=CARTESIAN_POINT('',(0.258177929547807,0.428187058065056,0.29));
#30583=CARTESIAN_POINT('',(0.24,0.41569219381653,0.1));
#30584=CARTESIAN_POINT('',(0.294105078908115,0.452882106690529,0.1));
#30585=CARTESIAN_POINT('',(0.24,0.41569219381653,0.56));
#30586=CARTESIAN_POINT('',(0.24,0.41569219381653,0.56));
#30587=CARTESIAN_POINT('',(0.294105078908115,0.452882106690529,0.56));
#30588=CARTESIAN_POINT('Origin',(0.267052539454057,0.448417858439125,0.56));
#30589=CARTESIAN_POINT('',(0.241731905082157,0.437682174717398,0.56));
#30590=CARTESIAN_POINT('Origin',(0.,0.,0.56));
#30591=CARTESIAN_POINT('',(0.24,0.41569219381653,0.56));
#30592=CARTESIAN_POINT('Origin',(0.24,0.41569219381653,0.56));
#30593=CARTESIAN_POINT('',(0.241731905082157,0.437682174717398,0.1));
#30594=CARTESIAN_POINT('',(0.241731905082157,0.437682174717398,0.29));
#30595=CARTESIAN_POINT('',(0.24,0.41569219381653,0.1));
#30596=CARTESIAN_POINT('Origin',(0.267052539454057,0.448417858439125,0.1));
#30597=CARTESIAN_POINT('Origin',(0.,0.,0.1));
#30598=CARTESIAN_POINT('Origin',(0.121473569345687,0.526159834984027,0.56));
#30599=CARTESIAN_POINT('',(0.0961592962762519,0.490666271247226,0.1));
#30600=CARTESIAN_POINT('',(0.0961592962762519,0.490666271247226,0.56));
#30601=CARTESIAN_POINT('',(0.0961592962762519,0.490666271247226,0.29));
#30602=CARTESIAN_POINT('',(0.0833511252801266,0.47270772144586,0.1));
#30603=CARTESIAN_POINT('',(0.121473569345687,0.526159834984027,0.1));
#30604=CARTESIAN_POINT('',(0.0833511252801266,0.47270772144586,0.56));
#30605=CARTESIAN_POINT('',(0.0833511252801266,0.47270772144586,0.56));
#30606=CARTESIAN_POINT('',(0.121473569345687,0.526159834984027,0.56));
#30607=CARTESIAN_POINT('Origin',(0.0936415073922334,0.504341321666087,0.56));
#30608=CARTESIAN_POINT('',(0.0774575672862878,0.493963890654054,0.56));
#30609=CARTESIAN_POINT('Origin',(0.,0.,0.56));
#30610=CARTESIAN_POINT('',(0.0833511252801266,0.47270772144586,0.56));
#30611=CARTESIAN_POINT('Origin',(0.0833511252801266,0.47270772144586,0.56));
#30612=CARTESIAN_POINT('',(0.0774575672862878,0.493963890654054,0.1));
#30613=CARTESIAN_POINT('',(0.0774575672862878,0.493963890654054,0.29));
#30614=CARTESIAN_POINT('',(0.0833511252801266,0.47270772144586,0.1));
#30615=CARTESIAN_POINT('Origin',(0.0936415073922334,0.504341321666087,0.1));
#30616=CARTESIAN_POINT('Origin',(0.,0.,0.1));
#30617=CARTESIAN_POINT('Origin',(-0.0658094454387796,0.535974921886314,
0.56));
#30618=CARTESIAN_POINT('',(-0.0774575672862878,0.493963890654054,0.1));
#30619=CARTESIAN_POINT('',(-0.0774575672862878,0.493963890654054,0.56));
#30620=CARTESIAN_POINT('',(-0.0774575672862878,0.493963890654054,0.29));
#30621=CARTESIAN_POINT('',(-0.0833511252801265,0.47270772144586,0.1));
#30622=CARTESIAN_POINT('',(-0.0658094454387796,0.535974921886314,0.1));
#30623=CARTESIAN_POINT('',(-0.0833511252801265,0.47270772144586,0.56));
#30624=CARTESIAN_POINT('',(-0.0833511252801265,0.47270772144586,0.56));
#30625=CARTESIAN_POINT('',(-0.0658094454387796,0.535974921886314,0.56));
#30626=CARTESIAN_POINT('Origin',(-0.0936415073922333,0.504341321666087,
0.56));
#30627=CARTESIAN_POINT('',(-0.0961592962762518,0.490666271247226,0.56));
#30628=CARTESIAN_POINT('Origin',(0.,0.,0.56));
#30629=CARTESIAN_POINT('',(-0.0833511252801265,0.47270772144586,0.56));
#30630=CARTESIAN_POINT('Origin',(-0.0833511252801265,0.47270772144586,0.56));
#30631=CARTESIAN_POINT('',(-0.0961592962762518,0.490666271247226,0.1));
#30632=CARTESIAN_POINT('',(-0.0961592962762518,0.490666271247226,0.29));
#30633=CARTESIAN_POINT('',(-0.0833511252801265,0.47270772144586,0.1));
#30634=CARTESIAN_POINT('Origin',(-0.0936415073922333,0.504341321666087,
0.1));
#30635=CARTESIAN_POINT('Origin',(0.,0.,0.1));
#30636=CARTESIAN_POINT('Origin',(-0.245154869859355,0.481143523061719,0.56));
#30637=CARTESIAN_POINT('',(-0.241731905082157,0.437682174717398,0.1));
#30638=CARTESIAN_POINT('',(-0.241731905082157,0.437682174717398,0.56));
#30639=CARTESIAN_POINT('',(-0.241731905082157,0.437682174717398,0.29));
#30640=CARTESIAN_POINT('',(-0.24,0.415692193816531,0.1));
#30641=CARTESIAN_POINT('',(-0.245154869859355,0.481143523061719,0.1));
#30642=CARTESIAN_POINT('',(-0.24,0.415692193816531,0.56));
#30643=CARTESIAN_POINT('',(-0.24,0.415692193816531,0.56));
#30644=CARTESIAN_POINT('',(-0.245154869859355,0.481143523061719,0.56));
#30645=CARTESIAN_POINT('Origin',(-0.267052539454057,0.448417858439125,0.56));
#30646=CARTESIAN_POINT('',(-0.258177929547807,0.428187058065056,0.56));
#30647=CARTESIAN_POINT('Origin',(0.,0.,0.56));
#30648=CARTESIAN_POINT('',(-0.24,0.415692193816531,0.56));
#30649=CARTESIAN_POINT('Origin',(-0.24,0.415692193816531,0.56));
#30650=CARTESIAN_POINT('',(-0.258177929547807,0.428187058065056,0.1));
#30651=CARTESIAN_POINT('',(-0.258177929547807,0.428187058065056,0.29));
#30652=CARTESIAN_POINT('',(-0.24,0.415692193816531,0.1));
#30653=CARTESIAN_POINT('Origin',(-0.267052539454057,0.448417858439125,0.1));
#30654=CARTESIAN_POINT('Origin',(0.,0.,0.1));
#30655=CARTESIAN_POINT('Origin',(-0.394930998874352,0.368279114433749,0.56));
#30656=CARTESIAN_POINT('',(-0.376849807542157,0.328609529008881,0.1));
#30657=CARTESIAN_POINT('',(-0.376849807542157,0.328609529008881,0.56));
#30658=CARTESIAN_POINT('',(-0.376849807542157,0.328609529008881,0.29));
#30659=CARTESIAN_POINT('',(-0.367701332697109,0.308538052649539,0.1));
#30660=CARTESIAN_POINT('',(-0.394930998874352,0.368279114433749,0.1));
#30661=CARTESIAN_POINT('',(-0.367701332697109,0.308538052649539,0.56));
#30662=CARTESIAN_POINT('',(-0.367701332697109,0.308538052649539,0.56));
#30663=CARTESIAN_POINT('',(-0.394930998874352,0.368279114433749,0.56));
#30664=CARTESIAN_POINT('Origin',(-0.399482254061324,0.338408583541644,0.56));
#30665=CARTESIAN_POINT('',(-0.389056494215466,0.314062166312295,0.56));
#30666=CARTESIAN_POINT('Origin',(0.,0.,0.56));
#30667=CARTESIAN_POINT('',(-0.367701332697109,0.308538052649539,0.56));
#30668=CARTESIAN_POINT('Origin',(-0.367701332697109,0.308538052649539,0.56));
#30669=CARTESIAN_POINT('',(-0.389056494215466,0.314062166312295,0.1));
#30670=CARTESIAN_POINT('',(-0.389056494215466,0.314062166312295,0.29));
#30671=CARTESIAN_POINT('',(-0.367701332697109,0.308538052649539,0.1));
#30672=CARTESIAN_POINT('Origin',(-0.399482254061324,0.338408583541644,0.1));
#30673=CARTESIAN_POINT('Origin',(0.,0.,0.1));
#30674=CARTESIAN_POINT('Origin',(-0.497072620864318,0.210994809384208,0.56));
#30675=CARTESIAN_POINT('',(-0.466514061501753,0.179901724341759,0.1));
#30676=CARTESIAN_POINT('',(-0.466514061501753,0.179901724341759,0.56));
#30677=CARTESIAN_POINT('',(-0.466514061501753,0.179901724341759,0.29));
#30678=CARTESIAN_POINT('',(-0.451052457977236,0.164169668796321,0.1));
#30679=CARTESIAN_POINT('',(-0.497072620864318,0.210994809384208,0.1));
#30680=CARTESIAN_POINT('',(-0.451052457977236,0.164169668796321,0.56));
#30681=CARTESIAN_POINT('',(-0.451052457977236,0.164169668796321,0.56));
#30682=CARTESIAN_POINT('',(-0.497072620864318,0.210994809384208,0.56));
#30683=CARTESIAN_POINT('Origin',(-0.483728513098638,0.184437764967243,0.56));
#30684=CARTESIAN_POINT('',(-0.473009103818409,0.162056742238344,0.56));
#30685=CARTESIAN_POINT('Origin',(0.,0.,0.56));
#30686=CARTESIAN_POINT('',(-0.451052457977236,0.164169668796321,0.56));
#30687=CARTESIAN_POINT('Origin',(-0.451052457977236,0.164169668796321,0.56));
#30688=CARTESIAN_POINT('',(-0.473009103818409,0.162056742238344,0.1));
#30689=CARTESIAN_POINT('',(-0.473009103818409,0.162056742238344,0.29));
#30690=CARTESIAN_POINT('',(-0.451052457977236,0.164169668796321,0.1));
#30691=CARTESIAN_POINT('Origin',(-0.483728513098638,0.184437764967243,0.1));
#30692=CARTESIAN_POINT('Origin',(0.,0.,0.1));
#30693=CARTESIAN_POINT('Origin',(0.509629974383735,0.,0.56));
#30694=CARTESIAN_POINT('',(0.499909834629964,-0.00949511665234232,0.56));
#30695=CARTESIAN_POINT('',(0.499909834629965,0.00949511665234234,0.56));
#30696=CARTESIAN_POINT('Origin',(0.,0.,0.56));
#30697=CARTESIAN_POINT('',(0.48,0.,0.56));
#30698=CARTESIAN_POINT('',(0.53925994876747,-0.0282614163711897,0.56));
#30699=CARTESIAN_POINT('',(0.48,0.,0.56));
#30700=CARTESIAN_POINT('Origin',(0.53925994876747,-0.0282614163711897,0.56));
#30701=CARTESIAN_POINT('',(0.499909834629964,-0.00949511665234232,0.1));
#30702=CARTESIAN_POINT('',(0.499909834629964,-0.00949511665234232,0.29));
#30703=CARTESIAN_POINT('',(0.48,0.,0.1));
#30704=CARTESIAN_POINT('',(0.53925994876747,-0.0282614163711897,0.1));
#30705=CARTESIAN_POINT('',(0.48,0.,0.56));
#30706=CARTESIAN_POINT('Origin',(0.48,0.,0.56));
#30707=CARTESIAN_POINT('',(0.499909834629965,0.00949511665234234,0.1));
#30708=CARTESIAN_POINT('',(0.499909834629965,0.00949511665234234,0.29));
#30709=CARTESIAN_POINT('',(0.48,0.,0.1));
#30710=CARTESIAN_POINT('Origin',(0.509629974383735,0.,0.1));
#30711=CARTESIAN_POINT('Origin',(0.,0.,0.1));
#30712=CARTESIAN_POINT('Origin',(-0.535974921886314,-0.0658094454387796,
0.56));
#30713=CARTESIAN_POINT('',(-0.493963890654054,-0.0774575672862878,0.1));
#30714=CARTESIAN_POINT('',(-0.493963890654054,-0.0774575672862878,0.56));
#30715=CARTESIAN_POINT('',(-0.493963890654054,-0.0774575672862878,0.29));
#30716=CARTESIAN_POINT('',(-0.47270772144586,-0.0833511252801266,0.1));
#30717=CARTESIAN_POINT('',(-0.535974921886314,-0.0658094454387796,0.1));
#30718=CARTESIAN_POINT('',(-0.47270772144586,-0.0833511252801266,0.56));
#30719=CARTESIAN_POINT('',(-0.47270772144586,-0.0833511252801266,0.56));
#30720=CARTESIAN_POINT('',(-0.535974921886314,-0.0658094454387796,0.56));
#30721=CARTESIAN_POINT('Origin',(-0.504341321666087,-0.0936415073922333,
0.56));
#30722=CARTESIAN_POINT('',(-0.490666271247226,-0.0961592962762519,0.56));
#30723=CARTESIAN_POINT('Origin',(0.,0.,0.56));
#30724=CARTESIAN_POINT('',(-0.47270772144586,-0.0833511252801266,0.56));
#30725=CARTESIAN_POINT('Origin',(-0.47270772144586,-0.0833511252801266,
0.56));
#30726=CARTESIAN_POINT('',(-0.490666271247226,-0.0961592962762519,0.1));
#30727=CARTESIAN_POINT('',(-0.490666271247226,-0.0961592962762519,0.29));
#30728=CARTESIAN_POINT('',(-0.47270772144586,-0.0833511252801266,0.1));
#30729=CARTESIAN_POINT('Origin',(-0.504341321666087,-0.0936415073922333,
0.1));
#30730=CARTESIAN_POINT('Origin',(0.,0.,0.1));
#30731=CARTESIAN_POINT('Origin',(-0.481143523061719,-0.245154869859355,
0.56));
#30732=CARTESIAN_POINT('',(-0.437682174717398,-0.241731905082157,0.1));
#30733=CARTESIAN_POINT('',(-0.437682174717398,-0.241731905082157,0.56));
#30734=CARTESIAN_POINT('',(-0.437682174717398,-0.241731905082157,0.29));
#30735=CARTESIAN_POINT('',(-0.41569219381653,-0.24,0.1));
#30736=CARTESIAN_POINT('',(-0.481143523061719,-0.245154869859355,0.1));
#30737=CARTESIAN_POINT('',(-0.41569219381653,-0.24,0.56));
#30738=CARTESIAN_POINT('',(-0.41569219381653,-0.24,0.56));
#30739=CARTESIAN_POINT('',(-0.481143523061719,-0.245154869859355,0.56));
#30740=CARTESIAN_POINT('Origin',(-0.448417858439125,-0.267052539454057,
0.56));
#30741=CARTESIAN_POINT('',(-0.428187058065056,-0.258177929547807,0.56));
#30742=CARTESIAN_POINT('Origin',(0.,0.,0.56));
#30743=CARTESIAN_POINT('',(-0.41569219381653,-0.24,0.56));
#30744=CARTESIAN_POINT('Origin',(-0.41569219381653,-0.24,0.56));
#30745=CARTESIAN_POINT('',(-0.428187058065056,-0.258177929547807,0.1));
#30746=CARTESIAN_POINT('',(-0.428187058065056,-0.258177929547807,0.29));
#30747=CARTESIAN_POINT('',(-0.41569219381653,-0.24,0.1));
#30748=CARTESIAN_POINT('Origin',(-0.448417858439125,-0.267052539454057,
0.1));
#30749=CARTESIAN_POINT('Origin',(0.,0.,0.1));
#30750=CARTESIAN_POINT('Origin',(-0.368279114433749,-0.394930998874352,
0.56));
#30751=CARTESIAN_POINT('',(-0.328609529008881,-0.376849807542157,0.1));
#30752=CARTESIAN_POINT('',(-0.328609529008881,-0.376849807542157,0.56));
#30753=CARTESIAN_POINT('',(-0.328609529008881,-0.376849807542157,0.29));
#30754=CARTESIAN_POINT('',(-0.308538052649539,-0.367701332697109,0.1));
#30755=CARTESIAN_POINT('',(-0.368279114433749,-0.394930998874352,0.1));
#30756=CARTESIAN_POINT('',(-0.308538052649539,-0.367701332697109,0.56));
#30757=CARTESIAN_POINT('',(-0.308538052649539,-0.367701332697109,0.56));
#30758=CARTESIAN_POINT('',(-0.368279114433749,-0.394930998874352,0.56));
#30759=CARTESIAN_POINT('Origin',(-0.338408583541644,-0.399482254061324,
0.56));
#30760=CARTESIAN_POINT('',(-0.314062166312295,-0.389056494215465,0.56));
#30761=CARTESIAN_POINT('Origin',(0.,0.,0.56));
#30762=CARTESIAN_POINT('',(-0.308538052649539,-0.367701332697109,0.56));
#30763=CARTESIAN_POINT('Origin',(-0.308538052649539,-0.367701332697109,
0.56));
#30764=CARTESIAN_POINT('',(-0.314062166312295,-0.389056494215465,0.1));
#30765=CARTESIAN_POINT('',(-0.314062166312295,-0.389056494215465,0.29));
#30766=CARTESIAN_POINT('',(-0.308538052649539,-0.367701332697109,0.1));
#30767=CARTESIAN_POINT('Origin',(-0.338408583541644,-0.399482254061324,
0.1));
#30768=CARTESIAN_POINT('Origin',(0.,0.,0.1));
#30769=CARTESIAN_POINT('Origin',(-0.210994809384208,-0.497072620864318,
0.56));
#30770=CARTESIAN_POINT('',(-0.179901724341759,-0.466514061501753,0.1));
#30771=CARTESIAN_POINT('',(-0.179901724341759,-0.466514061501753,0.56));
#30772=CARTESIAN_POINT('',(-0.179901724341759,-0.466514061501753,0.29));
#30773=CARTESIAN_POINT('',(-0.164169668796321,-0.451052457977236,0.1));
#30774=CARTESIAN_POINT('',(-0.210994809384208,-0.497072620864318,0.1));
#30775=CARTESIAN_POINT('',(-0.164169668796321,-0.451052457977236,0.56));
#30776=CARTESIAN_POINT('',(-0.164169668796321,-0.451052457977236,0.56));
#30777=CARTESIAN_POINT('',(-0.210994809384208,-0.497072620864318,0.56));
#30778=CARTESIAN_POINT('Origin',(-0.184437764967243,-0.483728513098638,
0.56));
#30779=CARTESIAN_POINT('',(-0.162056742238344,-0.473009103818409,0.56));
#30780=CARTESIAN_POINT('Origin',(0.,0.,0.56));
#30781=CARTESIAN_POINT('',(-0.164169668796321,-0.451052457977236,0.56));
#30782=CARTESIAN_POINT('Origin',(-0.164169668796321,-0.451052457977236,
0.56));
#30783=CARTESIAN_POINT('',(-0.162056742238344,-0.473009103818409,0.1));
#30784=CARTESIAN_POINT('',(-0.162056742238344,-0.473009103818409,0.29));
#30785=CARTESIAN_POINT('',(-0.164169668796321,-0.451052457977236,0.1));
#30786=CARTESIAN_POINT('Origin',(-0.184437764967243,-0.483728513098638,
0.1));
#30787=CARTESIAN_POINT('Origin',(0.,0.,0.1));
#30788=CARTESIAN_POINT('Origin',(-0.0282614163711899,-0.53925994876747,
0.56));
#30789=CARTESIAN_POINT('',(-0.00949511665234243,-0.499909834629964,0.1));
#30790=CARTESIAN_POINT('',(-0.00949511665234243,-0.499909834629964,0.56));
#30791=CARTESIAN_POINT('',(-0.00949511665234243,-0.499909834629964,0.29));
#30792=CARTESIAN_POINT('',(-8.81745695386094E-17,-0.48,0.1));
#30793=CARTESIAN_POINT('',(-0.0282614163711899,-0.53925994876747,0.1));
#30794=CARTESIAN_POINT('',(-8.81745695386094E-17,-0.48,0.56));
#30795=CARTESIAN_POINT('',(-8.81745695386094E-17,-0.48,0.56));
#30796=CARTESIAN_POINT('',(-0.0282614163711899,-0.53925994876747,0.56));
#30797=CARTESIAN_POINT('Origin',(-9.71445146547012E-17,-0.509629974383735,
0.56));
#30798=CARTESIAN_POINT('',(0.00949511665234229,-0.499909834629964,0.56));
#30799=CARTESIAN_POINT('Origin',(0.,0.,0.56));
#30800=CARTESIAN_POINT('',(-8.81745695386094E-17,-0.48,0.56));
#30801=CARTESIAN_POINT('Origin',(-8.81745695386094E-17,-0.48,0.56));
#30802=CARTESIAN_POINT('',(0.00949511665234229,-0.499909834629964,0.1));
#30803=CARTESIAN_POINT('',(0.00949511665234229,-0.499909834629964,0.29));
#30804=CARTESIAN_POINT('',(-8.81745695386094E-17,-0.48,0.1));
#30805=CARTESIAN_POINT('Origin',(-9.71445146547012E-17,-0.509629974383735,
0.1));
#30806=CARTESIAN_POINT('Origin',(0.,0.,0.1));
#30807=CARTESIAN_POINT('Origin',(0.157880720550278,-0.516404568220039,0.56));
#30808=CARTESIAN_POINT('',(0.162056742238344,-0.473009103818409,0.1));
#30809=CARTESIAN_POINT('',(0.162056742238344,-0.473009103818409,0.56));
#30810=CARTESIAN_POINT('',(0.162056742238344,-0.473009103818409,0.29));
#30811=CARTESIAN_POINT('',(0.164169668796321,-0.451052457977236,0.1));
#30812=CARTESIAN_POINT('',(0.157880720550278,-0.516404568220039,0.1));
#30813=CARTESIAN_POINT('',(0.164169668796321,-0.451052457977236,0.56));
#30814=CARTESIAN_POINT('',(0.164169668796321,-0.451052457977236,0.56));
#30815=CARTESIAN_POINT('',(0.157880720550278,-0.516404568220039,0.56));
#30816=CARTESIAN_POINT('Origin',(0.184437764967243,-0.483728513098638,0.56));
#30817=CARTESIAN_POINT('',(0.179901724341759,-0.466514061501753,0.56));
#30818=CARTESIAN_POINT('Origin',(0.,0.,0.56));
#30819=CARTESIAN_POINT('',(0.164169668796321,-0.451052457977236,0.56));
#30820=CARTESIAN_POINT('Origin',(0.164169668796321,-0.451052457977236,0.56));
#30821=CARTESIAN_POINT('',(0.179901724341759,-0.466514061501753,0.1));
#30822=CARTESIAN_POINT('',(0.179901724341759,-0.466514061501753,0.29));
#30823=CARTESIAN_POINT('',(0.164169668796321,-0.451052457977236,0.1));
#30824=CARTESIAN_POINT('Origin',(0.184437764967243,-0.483728513098638,0.1));
#30825=CARTESIAN_POINT('Origin',(0.,0.,0.1));
#30826=CARTESIAN_POINT('Origin',(0.324980112502106,-0.431263175425538,0.56));
#30827=CARTESIAN_POINT('',(0.314062166312295,-0.389056494215466,0.1));
#30828=CARTESIAN_POINT('',(0.314062166312295,-0.389056494215466,0.56));
#30829=CARTESIAN_POINT('',(0.314062166312295,-0.389056494215466,0.29));
#30830=CARTESIAN_POINT('',(0.308538052649539,-0.367701332697109,0.1));
#30831=CARTESIAN_POINT('',(0.324980112502106,-0.431263175425538,0.1));
#30832=CARTESIAN_POINT('',(0.308538052649539,-0.367701332697109,0.56));
#30833=CARTESIAN_POINT('',(0.308538052649539,-0.367701332697109,0.56));
#30834=CARTESIAN_POINT('',(0.324980112502106,-0.431263175425538,0.56));
#30835=CARTESIAN_POINT('Origin',(0.338408583541644,-0.399482254061324,0.56));
#30836=CARTESIAN_POINT('',(0.328609529008881,-0.376849807542158,0.56));
#30837=CARTESIAN_POINT('Origin',(0.,0.,0.56));
#30838=CARTESIAN_POINT('',(0.308538052649539,-0.367701332697109,0.56));
#30839=CARTESIAN_POINT('Origin',(0.308538052649539,-0.367701332697109,0.56));
#30840=CARTESIAN_POINT('',(0.328609529008881,-0.376849807542158,0.1));
#30841=CARTESIAN_POINT('',(0.328609529008881,-0.376849807542158,0.29));
#30842=CARTESIAN_POINT('',(0.308538052649539,-0.367701332697109,0.1));
#30843=CARTESIAN_POINT('Origin',(0.338408583541644,-0.399482254061324,0.1));
#30844=CARTESIAN_POINT('Origin',(0.,0.,0.1));
#30845=CARTESIAN_POINT('Origin',(0.452882106690529,-0.294105078908115,0.56));
#30846=CARTESIAN_POINT('',(0.428187058065056,-0.258177929547807,0.1));
#30847=CARTESIAN_POINT('',(0.428187058065056,-0.258177929547807,0.56));
#30848=CARTESIAN_POINT('',(0.428187058065056,-0.258177929547807,0.29));
#30849=CARTESIAN_POINT('',(0.41569219381653,-0.24,0.1));
#30850=CARTESIAN_POINT('',(0.452882106690529,-0.294105078908115,0.1));
#30851=CARTESIAN_POINT('',(0.41569219381653,-0.24,0.56));
#30852=CARTESIAN_POINT('',(0.41569219381653,-0.24,0.56));
#30853=CARTESIAN_POINT('',(0.452882106690529,-0.294105078908115,0.56));
#30854=CARTESIAN_POINT('Origin',(0.448417858439125,-0.267052539454057,0.56));
#30855=CARTESIAN_POINT('',(0.437682174717398,-0.241731905082157,0.56));
#30856=CARTESIAN_POINT('Origin',(0.,0.,0.56));
#30857=CARTESIAN_POINT('',(0.41569219381653,-0.24,0.56));
#30858=CARTESIAN_POINT('Origin',(0.41569219381653,-0.24,0.56));
#30859=CARTESIAN_POINT('',(0.437682174717398,-0.241731905082157,0.1));
#30860=CARTESIAN_POINT('',(0.437682174717398,-0.241731905082157,0.29));
#30861=CARTESIAN_POINT('',(0.41569219381653,-0.24,0.1));
#30862=CARTESIAN_POINT('Origin',(0.448417858439125,-0.267052539454057,0.1));
#30863=CARTESIAN_POINT('Origin',(0.,0.,0.1));
#30864=CARTESIAN_POINT('Origin',(0.526159834984027,-0.121473569345687,0.56));
#30865=CARTESIAN_POINT('',(0.490666271247226,-0.096159296276252,0.1));
#30866=CARTESIAN_POINT('',(0.490666271247226,-0.096159296276252,0.56));
#30867=CARTESIAN_POINT('',(0.490666271247226,-0.096159296276252,0.29));
#30868=CARTESIAN_POINT('',(0.47270772144586,-0.0833511252801266,0.1));
#30869=CARTESIAN_POINT('',(0.526159834984027,-0.121473569345687,0.1));
#30870=CARTESIAN_POINT('',(0.47270772144586,-0.0833511252801266,0.56));
#30871=CARTESIAN_POINT('',(0.47270772144586,-0.0833511252801266,0.56));
#30872=CARTESIAN_POINT('',(0.526159834984027,-0.121473569345687,0.56));
#30873=CARTESIAN_POINT('Origin',(0.504341321666087,-0.0936415073922334,
0.56));
#30874=CARTESIAN_POINT('',(0.493963890654054,-0.0774575672862878,0.56));
#30875=CARTESIAN_POINT('Origin',(0.,0.,0.56));
#30876=CARTESIAN_POINT('',(0.47270772144586,-0.0833511252801266,0.56));
#30877=CARTESIAN_POINT('Origin',(0.47270772144586,-0.0833511252801266,0.56));
#30878=CARTESIAN_POINT('',(0.493963890654054,-0.0774575672862878,0.1));
#30879=CARTESIAN_POINT('',(0.493963890654054,-0.0774575672862878,0.29));
#30880=CARTESIAN_POINT('',(0.47270772144586,-0.0833511252801266,0.1));
#30881=CARTESIAN_POINT('Origin',(0.504341321666087,-0.0936415073922334,
0.1));
#30882=CARTESIAN_POINT('Origin',(0.,0.,0.1));
#30883=CARTESIAN_POINT('Origin',(0.,0.,-0.0249999999999999));
#30884=CARTESIAN_POINT('',(-0.298,-3.64944746145911E-17,-0.0249999999999999));
#30885=CARTESIAN_POINT('Origin',(0.,0.,-0.0249999999999999));
#30886=CARTESIAN_POINT('',(-0.323,-3.95560916124595E-17,0.));
#30887=CARTESIAN_POINT('Origin',(-0.323,-3.95560916124595E-17,-0.0249999999999999));
#30888=CARTESIAN_POINT('Origin',(0.,0.,0.));
#30889=CARTESIAN_POINT('Origin',(0.,0.,-1.8));
#30890=CARTESIAN_POINT('',(-0.298,-3.64944746145911E-17,-3.6));
#30891=CARTESIAN_POINT('',(-0.298,-3.64944746145911E-17,-1.8));
#30892=CARTESIAN_POINT('Origin',(0.,0.,-3.6));
#30893=CARTESIAN_POINT('Origin',(0.48,0.,0.));
#30894=CARTESIAN_POINT('',(-0.48,-5.8783046359073E-17,3.46944695195361E-18));
#30895=CARTESIAN_POINT('Origin',(0.,0.,0.));
#30896=CARTESIAN_POINT('Origin',(0.26,0.,-6.));
#30897=CARTESIAN_POINT('',(-0.26,-3.18408167778312E-17,-6.));
#30898=CARTESIAN_POINT('Origin',(0.,0.,-6.));
#30899=CARTESIAN_POINT('Origin',(0.,0.,-5.98));
#30900=CARTESIAN_POINT('',(-0.28,-3.42901103761259E-17,-5.98));
#30901=CARTESIAN_POINT('Origin',(0.,0.,-4.78));
#30902=CARTESIAN_POINT('Origin',(0.,0.,-3.6));
#30903=CARTESIAN_POINT('Origin',(0.298,0.,-3.6));
#30904=CARTESIAN_POINT('Origin',(0.,0.,0.01));
#30905=CARTESIAN_POINT('',(-0.5,-6.12323399573677E-17,0.02));
#30906=CARTESIAN_POINT('Origin',(0.,0.,0.02));
#30907=CARTESIAN_POINT('',(-0.49,-6.00076931582203E-17,0.01));
#30908=CARTESIAN_POINT('Origin',(0.,0.,0.29));
#30909=CARTESIAN_POINT('Origin',(0.,0.,0.56));
#30910=CARTESIAN_POINT('Origin',(0.,0.,0.56));
#30911=CARTESIAN_POINT('Origin',(0.,0.,0.56));
#30912=CARTESIAN_POINT('Origin',(0.,0.,0.56));
#30913=CARTESIAN_POINT('Origin',(0.,0.,0.56));
#30914=CARTESIAN_POINT('Origin',(0.,0.,0.56));
#30915=CARTESIAN_POINT('Origin',(0.,0.,0.56));
#30916=CARTESIAN_POINT('Origin',(0.,0.,0.56));
#30917=CARTESIAN_POINT('Origin',(0.,0.,0.56));
#30918=CARTESIAN_POINT('Origin',(0.,0.,0.56));
#30919=CARTESIAN_POINT('Origin',(0.,0.,0.56));
#30920=CARTESIAN_POINT('Origin',(0.,0.,0.56));
#30921=CARTESIAN_POINT('Origin',(0.,0.,0.56));
#30922=CARTESIAN_POINT('Origin',(0.,0.,0.56));
#30923=CARTESIAN_POINT('Origin',(0.,0.,0.56));
#30924=CARTESIAN_POINT('Origin',(0.,0.,0.56));
#30925=CARTESIAN_POINT('',(-0.5,-6.12323399573677E-17,0.29));
#30926=CARTESIAN_POINT('Origin',(0.,0.,0.56));
#30927=CARTESIAN_POINT('Origin',(0.,0.,0.56));
#30928=CARTESIAN_POINT('Origin',(0.,0.,0.56));
#30929=CARTESIAN_POINT('Origin',(0.,0.,0.56));
#30930=CARTESIAN_POINT('Origin',(0.,0.,0.56));
#30931=CARTESIAN_POINT('Origin',(0.,0.,0.56));
#30932=CARTESIAN_POINT('Origin',(0.,0.,0.56));
#30933=CARTESIAN_POINT('Origin',(0.,0.,0.56));
#30934=CARTESIAN_POINT('Origin',(0.,0.,0.56));
#30935=CARTESIAN_POINT('Origin',(0.,0.,0.56));
#30936=CARTESIAN_POINT('Origin',(0.,0.,0.56));
#30937=CARTESIAN_POINT('Origin',(0.,0.,0.56));
#30938=CARTESIAN_POINT('Origin',(0.,0.,0.56));
#30939=CARTESIAN_POINT('Origin',(0.,0.,0.56));
#30940=CARTESIAN_POINT('Origin',(0.,0.,0.56));
#30941=CARTESIAN_POINT('Origin',(0.,0.,0.56));
#30942=CARTESIAN_POINT('Origin',(0.,0.,0.56));
#30943=CARTESIAN_POINT('Origin',(0.,0.,0.56));
#30944=CARTESIAN_POINT('Origin',(0.,0.,0.56));
#30945=CARTESIAN_POINT('Origin',(0.,0.,0.56));
#30946=CARTESIAN_POINT('Origin',(0.,0.,0.58));
#30947=CARTESIAN_POINT('',(-0.46,-5.63337527607782E-17,0.6));
#30948=CARTESIAN_POINT('Origin',(0.,0.,0.6));
#30949=CARTESIAN_POINT('',(-0.48,-5.87830463590729E-17,0.58));
#30950=CARTESIAN_POINT('Origin',(0.,0.,0.6));
#31622=UNCERTAINTY_MEASURE_WITH_UNIT(LENGTH_MEASURE(0.001),#31639,
'DISTANCE_ACCURACY_VALUE',
'Maximum model space distance between geometric entities at asserted c
onnectivities');
#31625=UNCERTAINTY_MEASURE_WITH_UNIT(LENGTH_MEASURE(0.001),#31639,
'DISTANCE_ACCURACY_VALUE',
'Maximum model space distance between geometric entities at asserted c
onnectivities');
#31635=(
GEOMETRIC_REPRESENTATION_CONTEXT(3)
GLOBAL_UNCERTAINTY_ASSIGNED_CONTEXT((#31622))
GLOBAL_UNIT_ASSIGNED_CONTEXT((#31639,#31641,#31642))
REPRESENTATION_CONTEXT('','3D')
);
#31638=(
GEOMETRIC_REPRESENTATION_CONTEXT(3)
GLOBAL_UNCERTAINTY_ASSIGNED_CONTEXT((#31625))
GLOBAL_UNIT_ASSIGNED_CONTEXT((#31639,#31641,#31642))
REPRESENTATION_CONTEXT('','3D')
);
#31639=(
LENGTH_UNIT()
NAMED_UNIT(*)
SI_UNIT(.CENTI.,.METRE.)
);
#31641=(
NAMED_UNIT(*)
PLANE_ANGLE_UNIT()
SI_UNIT($,.RADIAN.)
);
#31642=(
NAMED_UNIT(*)
SI_UNIT($,.STERADIAN.)
SOLID_ANGLE_UNIT()
);
#31652=SHAPE_DEFINITION_REPRESENTATION(#31664,#31713);
#31664=PRODUCT_DEFINITION_SHAPE('',$,#31726);
#31713=SHAPE_REPRESENTATION('',(#13175),#31635);
#31716=PRODUCT_DEFINITION_CONTEXT('part definition',#31754,'design');
#31726=PRODUCT_DEFINITION('2026-10-22-02-42-24-626',
'09_ISO_4762_M6x60-8.8_Socket_Head_Cap_Screw',#31738,#31716);
#31738=PRODUCT_DEFINITION_FORMATION('',$,#31765);
#31754=APPLICATION_CONTEXT(
'Core Data for Automotive Mechanical Design Process');
#31755=PRODUCT_CONTEXT('part definition',#31754,'mechanical');
#31765=PRODUCT('2026-10-22-02-42-24-626',
'09_ISO_4762_M6x60-8.8_Socket_Head_Cap_Screw',$,(#31755));
#31831=COLOUR_RGB('Black',0.12,0.14,0.17);
#31832=FILL_AREA_STYLE_COLOUR('',#31831);
#31833=FILL_AREA_STYLE('',(#31832));
#31834=SURFACE_STYLE_FILL_AREA(#31833);
#31835=SURFACE_SIDE_STYLE('',(#31834));
#31836=SURFACE_STYLE_USAGE(.BOTH.,#31835);
#31837=PRESENTATION_STYLE_ASSIGNMENT((#31836));
ENDSEC;
END-ISO-10303-21;
